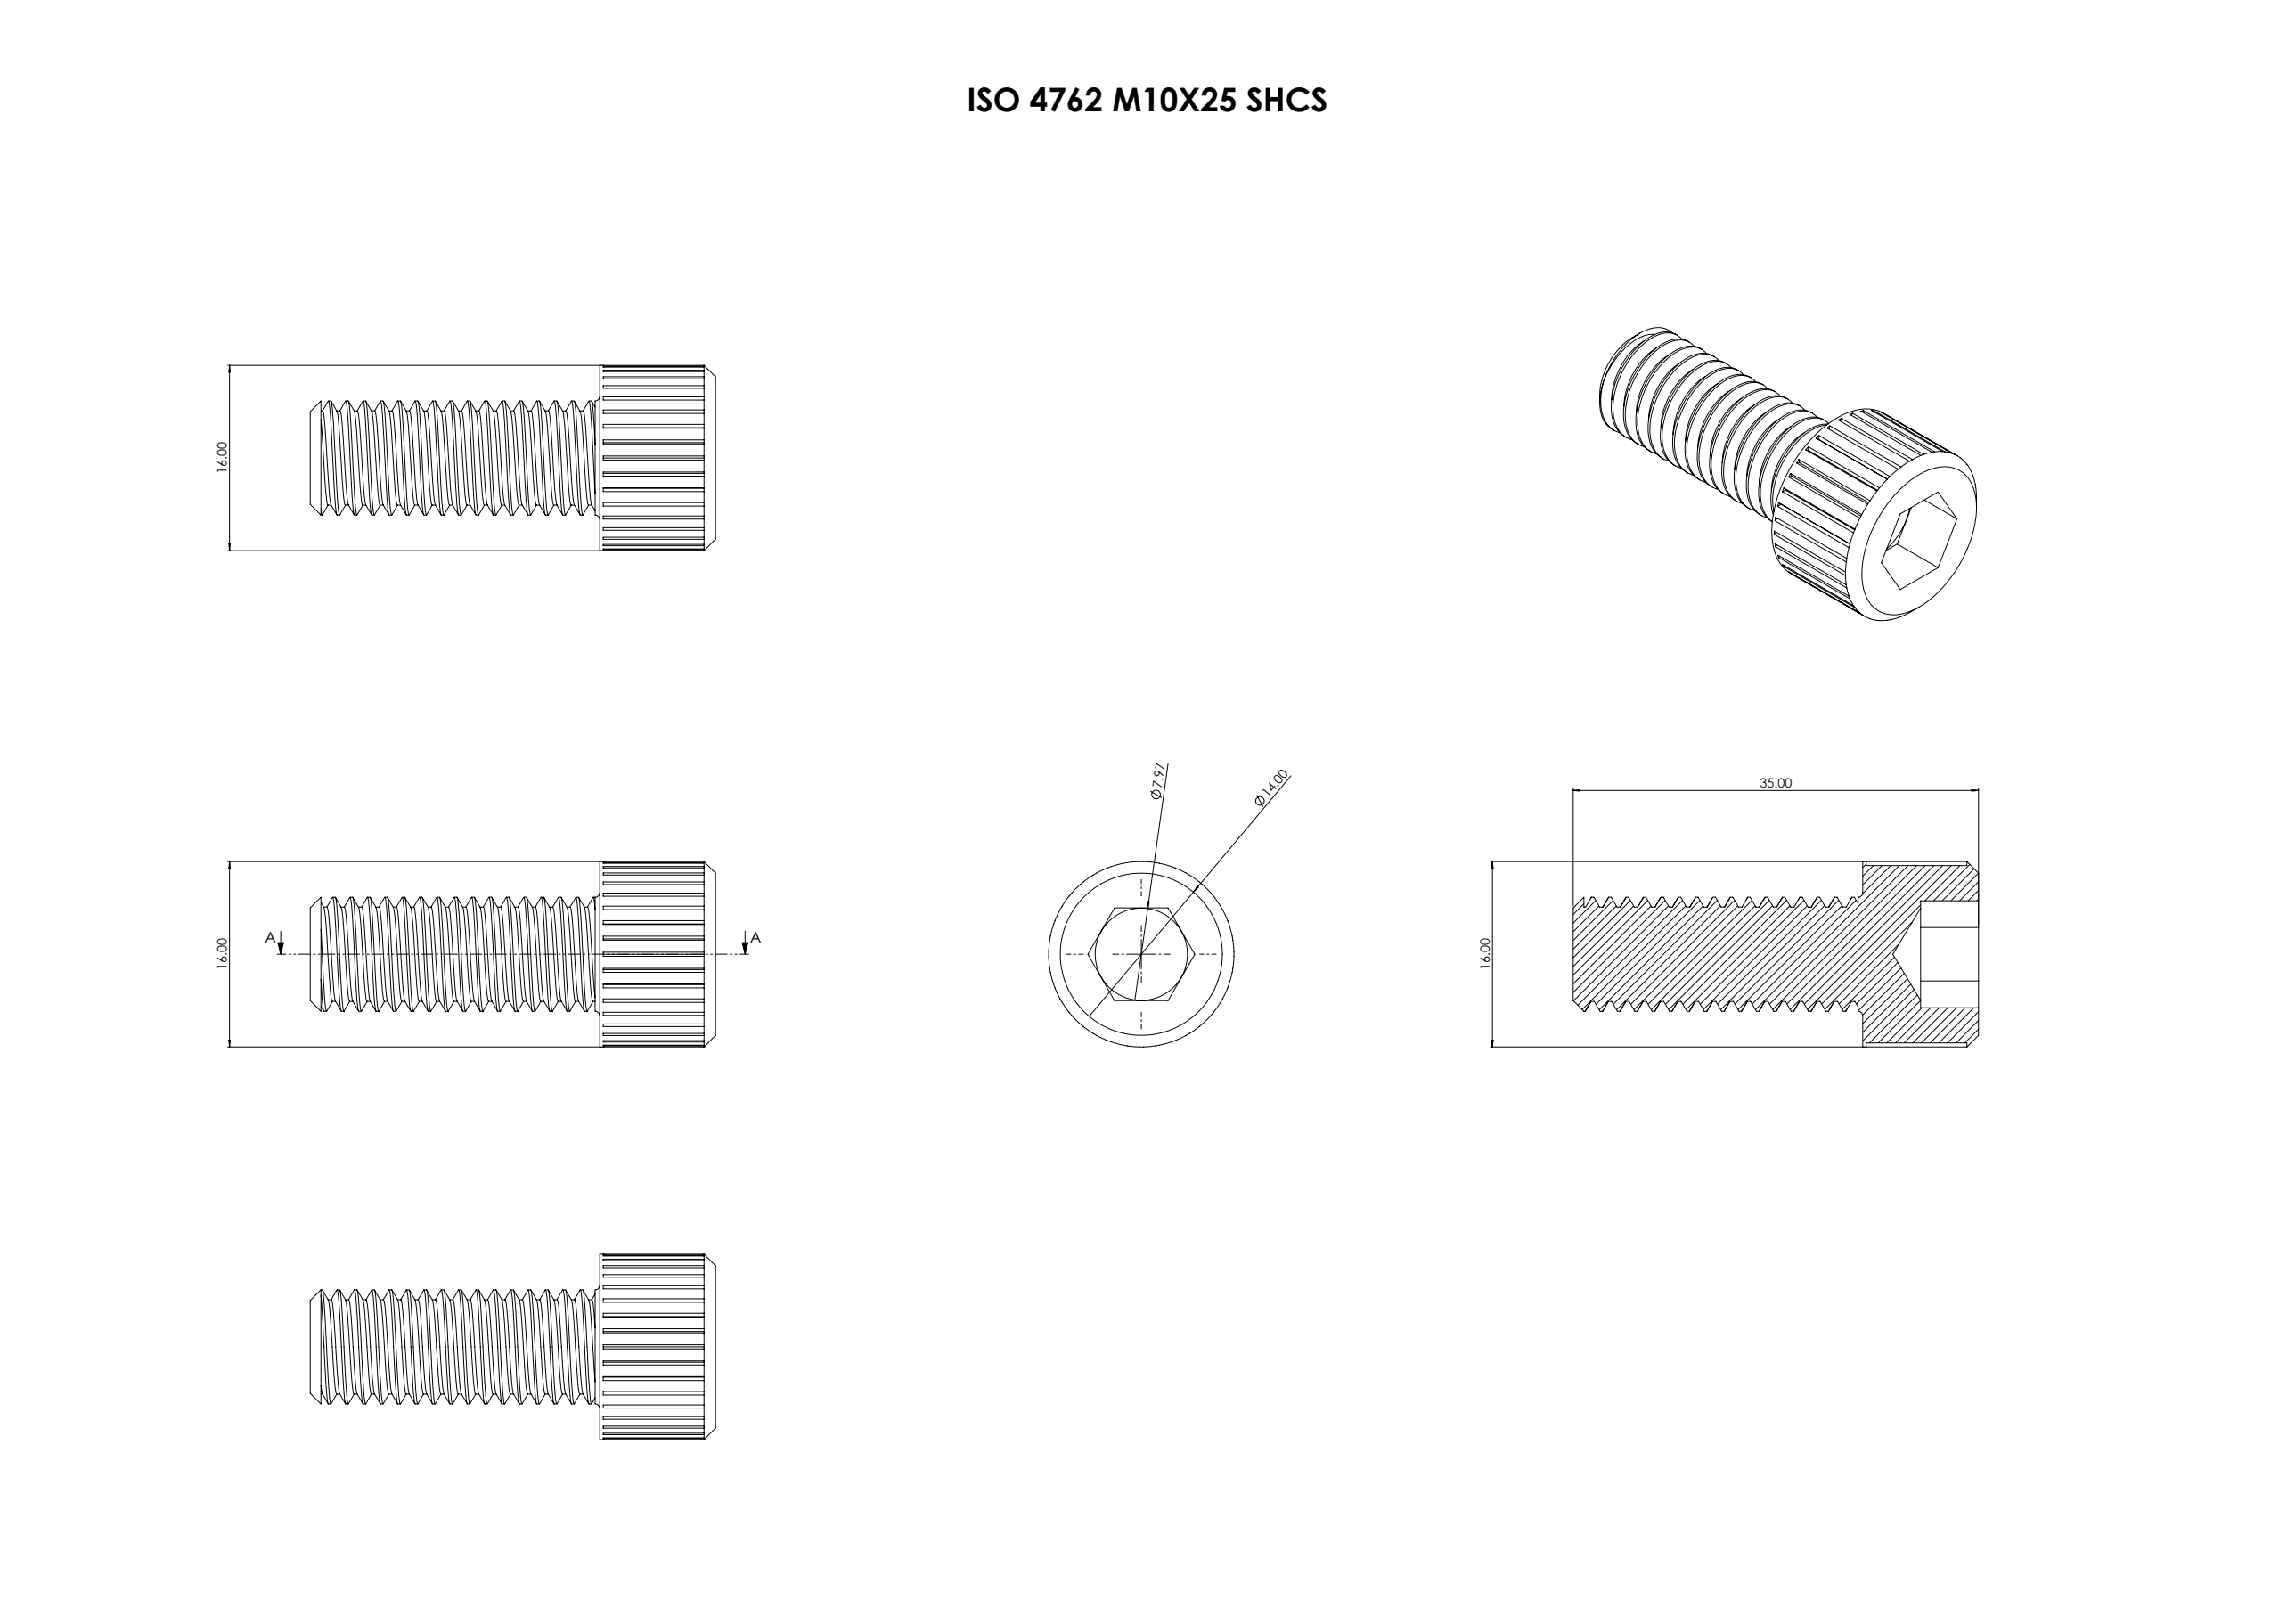
ISO-10303-21;
HEADER;
/* Generated by software containing ST-Developer
 * from STEP Tools, Inc. (www.steptools.com) 
 */

FILE_DESCRIPTION(
/* description */ (''),
/* implementation_level */ '2;1');

FILE_NAME(
/* name */ '06_ISO_4762_M10x25_SHCS.step',
/* time_stamp */ '2026-10-11T08:27:52-07:00',
/* author */ (''),
/* organization */ (''),
/* preprocessor_version */ 'ST-DEVELOPER v20.2',
/* originating_system */ 'Autodesk Translation Framework v15.15.0.0',
/* authorisation */ '');

FILE_SCHEMA (('AUTOMOTIVE_DESIGN { 1 0 10303 214 3 1 1 }'));
ENDSEC;

DATA;
#10=MECHANICAL_DESIGN_GEOMETRIC_PRESENTATION_REPRESENTATION('',(#924),#94301);
#479=B_SPLINE_CURVE_WITH_KNOTS('',3,(#84087,#84088,#84089,#84090,#84091,
#84092,#84093,#84094,#84095,#84096),.UNSPECIFIED.,.F.,.F.,(4,3,3,4),(-4.0932327200247,
-3.97004432054779,-2.97753324041084,-2.06652207565086),.UNSPECIFIED.);
#480=B_SPLINE_CURVE_WITH_KNOTS('',3,(#84099,#84100,#84101,#84102,#84103,
#84104,#84105,#84106,#84107,#84108),.UNSPECIFIED.,.F.,.F.,(4,3,3,4),(0.,
0.496255540068463,0.992511080136944,1.11488200921589),.UNSPECIFIED.);
#481=B_SPLINE_CURVE_WITH_KNOTS('',3,(#84113,#84114,#84115,#84116,#84117,
#84118,#84119,#84120,#84121,#84122,#84123,#84124,#84125,#84126,#84127,#84128,
#84129,#84130,#84131,#84132,#84133,#84134),.UNSPECIFIED.,.F.,.F.,(4,3,3,
3,3,3,3,4),(-10.3764180272043,-9.92511080136948,-8.93259972123253,-7.94008864109558,
-6.94757756095863,-5.95506648082169,-4.96255540068474,-4.0932327200247),
 .UNSPECIFIED.);
#482=B_SPLINE_CURVE_WITH_KNOTS('',3,(#84135,#84136,#84137,#84138,#84139,
#84140,#84141,#84142,#84143,#84144,#84145,#84146,#84147,#84148,#84149,#84150,
#84151,#84152,#84153,#84154,#84155,#84156),.UNSPECIFIED.,.F.,.F.,(4,3,3,
3,3,3,3,4),(1.11488200921589,1.98502216027389,2.97753324041084,3.97004432054779,
4.96255540068474,5.95506648082169,6.94757756095864,7.39806731639547),
 .UNSPECIFIED.);
#483=B_SPLINE_CURVE_WITH_KNOTS('',3,(#84161,#84162,#84163,#84164,#84165,
#84166,#84167,#84168,#84169,#84170,#84171,#84172,#84173,#84174,#84175,#84176,
#84177,#84178,#84179,#84180,#84181,#84182),.UNSPECIFIED.,.F.,.F.,(4,3,3,
3,3,3,3,4),(-16.6596033343839,-15.8801772821912,-14.8876662020542,-13.8951551219173,
-12.9026440417803,-11.9101329616434,-10.9176218815064,-10.3764180272043),
 .UNSPECIFIED.);
#484=B_SPLINE_CURVE_WITH_KNOTS('',3,(#84183,#84184,#84185,#84186,#84187,
#84188,#84189,#84190,#84191,#84192,#84193,#84194,#84195,#84196,#84197,#84198,
#84199,#84200,#84201,#84202,#84203,#84204),.UNSPECIFIED.,.F.,.F.,(4,3,3,
3,3,3,3,4),(7.39806731639547,7.94008864109559,8.93259972123253,9.92511080136948,
10.9176218815064,11.9101329616434,12.9026440417803,13.681252623575),
 .UNSPECIFIED.);
#485=B_SPLINE_CURVE_WITH_KNOTS('',3,(#84209,#84210,#84211,#84212,#84213,
#84214,#84215,#84216,#84217,#84218,#84219,#84220,#84221,#84222,#84223,#84224,
#84225,#84226,#84227,#84228,#84229,#84230,#84231,#84232,#84233),
 .UNSPECIFIED.,.F.,.F.,(4,3,3,3,3,3,3,3,4),(-22.9427886415635,-22.8277548431498,
-21.8352437630129,-20.8427326828759,-19.850221602739,-18.857710522602,-17.8651994424651,
-16.8726883623281,-16.6596033343839),.UNSPECIFIED.);
#486=B_SPLINE_CURVE_WITH_KNOTS('',3,(#84234,#84235,#84236,#84237,#84238,
#84239,#84240,#84241,#84242,#84243,#84244,#84245,#84246,#84247,#84248,#84249,
#84250,#84251,#84252,#84253,#84254,#84255,#84256,#84257,#84258),
 .UNSPECIFIED.,.F.,.F.,(4,3,3,3,3,3,3,3,4),(13.681252623575,13.8951551219173,
14.8876662020542,15.8801772821912,16.8726883623281,17.8651994424651,18.857710522602,
19.8502216027389,19.9644379307546),.UNSPECIFIED.);
#487=B_SPLINE_CURVE_WITH_KNOTS('',3,(#84263,#84264,#84265,#84266,#84267,
#84268,#84269,#84270,#84271,#84272,#84273,#84274,#84275,#84276,#84277,#84278,
#84279,#84280,#84281,#84282,#84283,#84284),.UNSPECIFIED.,.F.,.F.,(4,3,3,
3,3,3,3,4),(-29.225973948743,-28.7828213239715,-27.7903102438345,-26.7977991636976,
-25.8052880835606,-24.8127770034237,-23.8202659232867,-22.9427886415635),
 .UNSPECIFIED.);
#488=B_SPLINE_CURVE_WITH_KNOTS('',3,(#84285,#84286,#84287,#84288,#84289,
#84290,#84291,#84292,#84293,#84294,#84295,#84296,#84297,#84298,#84299,#84300,
#84301,#84302,#84303,#84304,#84305,#84306),.UNSPECIFIED.,.F.,.F.,(4,3,3,
3,3,3,3,4),(19.9644379307546,20.8427326828759,21.8352437630128,22.8277548431498,
23.8202659232867,24.8127770034237,25.8052880835606,26.2476232379342),
 .UNSPECIFIED.);
#489=B_SPLINE_CURVE_WITH_KNOTS('',3,(#84311,#84312,#84313,#84314,#84315,
#84316,#84317,#84318,#84319,#84320,#84321,#84322,#84323,#84324,#84325,#84326,
#84327,#84328,#84329,#84330,#84331,#84332),.UNSPECIFIED.,.F.,.F.,(4,3,3,
3,3,3,3,4),(-35.5091592559226,-34.7378878047932,-33.7453767246562,-32.7528656445193,
-31.7603545643823,-30.7678434842454,-29.7753324041084,-29.225973948743),
 .UNSPECIFIED.);
#490=B_SPLINE_CURVE_WITH_KNOTS('',3,(#84333,#84334,#84335,#84336,#84337,
#84338,#84339,#84340,#84341,#84342,#84343,#84344,#84345,#84346,#84347,#84348,
#84349,#84350,#84351,#84352,#84353,#84354),.UNSPECIFIED.,.F.,.F.,(4,3,3,
3,3,3,3,4),(26.2476232379342,26.7977991636976,27.7903102438345,28.7828213239715,
29.7753324041084,30.7678434842454,31.7603545643823,32.5308085451138),
 .UNSPECIFIED.);
#491=B_SPLINE_CURVE_WITH_KNOTS('',3,(#84359,#84360,#84361,#84362,#84363,
#84364,#84365,#84366,#84367,#84368,#84369,#84370,#84371,#84372,#84373,#84374,
#84375,#84376,#84377,#84378,#84379,#84380,#84381,#84382,#84383),
 .UNSPECIFIED.,.F.,.F.,(4,3,3,3,3,3,3,3,4),(-41.7923445631022,-41.6854653657518,
-40.6929542856149,-39.7004432054779,-38.707932125341,-37.715421045204,-36.7229099650671,
-35.7303988849301,-35.5091592559226),.UNSPECIFIED.);
#492=B_SPLINE_CURVE_WITH_KNOTS('',3,(#84384,#84385,#84386,#84387,#84388,
#84389,#84390,#84391,#84392,#84393,#84394,#84395,#84396,#84397,#84398,#84399,
#84400,#84401,#84402,#84403,#84404,#84405,#84406,#84407,#84408),
 .UNSPECIFIED.,.F.,.F.,(4,3,3,3,3,3,3,3,4),(32.5308085451138,32.7528656445192,
33.7453767246562,34.7378878047931,35.7303988849301,36.722909965067,37.715421045204,
38.7079321253409,38.8139938522934),.UNSPECIFIED.);
#493=B_SPLINE_CURVE_WITH_KNOTS('',3,(#84413,#84414,#84415,#84416,#84417,
#84418,#84419,#84420,#84421,#84422,#84423,#84424,#84425,#84426,#84427,#84428,
#84429,#84430,#84431,#84432,#84433,#84434),.UNSPECIFIED.,.F.,.F.,(4,3,3,
3,3,3,3,4),(-48.0755298702818,-47.6405318465735,-46.6480207664365,-45.6555096862996,
-44.6629986061626,-43.6704875260257,-42.6779764458888,-41.7923445631022),
 .UNSPECIFIED.);
#494=B_SPLINE_CURVE_WITH_KNOTS('',3,(#84435,#84436,#84437,#84438,#84439,
#84440,#84441,#84442,#84443,#84444,#84445,#84446,#84447,#84448,#84449,#84450,
#84451,#84452,#84453,#84454,#84455,#84456),.UNSPECIFIED.,.F.,.F.,(4,3,3,
3,3,3,3,4),(38.8139938522934,39.7004432054779,40.6929542856148,41.6854653657518,
42.6779764458887,43.6704875260257,44.6629986061626,45.097179159473),
 .UNSPECIFIED.);
#495=B_SPLINE_CURVE_WITH_KNOTS('',3,(#84461,#84462,#84463,#84464,#84465,
#84466,#84467,#84468,#84469,#84470,#84471,#84472,#84473,#84474,#84475,#84476,
#84477,#84478,#84479,#84480,#84481,#84482),.UNSPECIFIED.,.F.,.F.,(4,3,3,
3,3,3,3,4),(-54.3587151774614,-53.5955983273952,-52.6030872472582,-51.6105761671213,
-50.6180650869843,-49.6255540068474,-48.6330429267104,-48.0755298702818),
 .UNSPECIFIED.);
#496=B_SPLINE_CURVE_WITH_KNOTS('',3,(#84483,#84484,#84485,#84486,#84487,
#84488,#84489,#84490,#84491,#84492,#84493,#84494,#84495,#84496,#84497,#84498,
#84499,#84500,#84501,#84502,#84503,#84504),.UNSPECIFIED.,.F.,.F.,(4,3,3,
3,3,3,3,4),(45.097179159473,45.6555096862996,46.6480207664365,47.6405318465735,
48.6330429267104,49.6255540068474,50.6180650869843,51.3803644666526),
 .UNSPECIFIED.);
#497=B_SPLINE_CURVE_WITH_KNOTS('',3,(#84509,#84510,#84511,#84512,#84513,
#84514,#84515,#84516,#84517,#84518,#84519,#84520,#84521,#84522,#84523,#84524,
#84525,#84526,#84527,#84528,#84529,#84530,#84531,#84532,#84533),
 .UNSPECIFIED.,.F.,.F.,(4,3,3,3,3,3,3,3,4),(-60.641900484641,-60.5431758883538,
-59.5506648082169,-58.5581537280799,-57.565642647943,-56.573131567806,-55.5806204876691,
-54.5881094075321,-54.3587151774614),.UNSPECIFIED.);
#498=B_SPLINE_CURVE_WITH_KNOTS('',3,(#84534,#84535,#84536,#84537,#84538,
#84539,#84540,#84541,#84542,#84543,#84544,#84545,#84546,#84547,#84548,#84549,
#84550,#84551,#84552,#84553,#84554,#84555,#84556,#84557,#84558),
 .UNSPECIFIED.,.F.,.F.,(4,3,3,3,3,3,3,3,4),(51.3803644666526,51.6105761671213,
52.6030872472582,53.5955983273952,54.5881094075321,55.5806204876691,56.573131567806,
57.565642647943,57.6635497738322),.UNSPECIFIED.);
#499=B_SPLINE_CURVE_WITH_KNOTS('',3,(#84563,#84564,#84565,#84566,#84567,
#84568,#84569,#84570,#84571,#84572,#84573,#84574,#84575,#84576,#84577,#84578,
#84579,#84580,#84581,#84582,#84583,#84584),.UNSPECIFIED.,.F.,.F.,(4,3,3,
3,3,3,3,4),(-66.9250857918206,-66.4982423691755,-65.5057312890386,-64.5132202089016,
-63.5207091287647,-62.5281980486277,-61.5356869684908,-60.641900484641),
 .UNSPECIFIED.);
#500=B_SPLINE_CURVE_WITH_KNOTS('',3,(#84585,#84586,#84587,#84588,#84589,
#84590,#84591,#84592,#84593,#84594,#84595,#84596,#84597,#84598,#84599,#84600,
#84601,#84602,#84603,#84604,#84605,#84606),.UNSPECIFIED.,.F.,.F.,(4,3,3,
3,3,3,3,4),(57.6635497738322,58.5581537280799,59.5506648082169,60.5431758883538,
61.5356869684908,62.5281980486277,63.5207091287646,63.9467350810118),
 .UNSPECIFIED.);
#501=B_SPLINE_CURVE_WITH_KNOTS('',3,(#84611,#84612,#84613,#84614,#84615,
#84616,#84617,#84618,#84619,#84620,#84621,#84622,#84623,#84624,#84625,#84626,
#84627,#84628,#84629,#84630,#84631,#84632),.UNSPECIFIED.,.F.,.F.,(4,3,3,
3,3,3,3,4),(-73.2082710990002,-72.4533088499972,-71.4607977698602,-70.4682866897233,
-69.4757756095863,-68.4832645294494,-67.4907534493124,-66.9250857918206),
 .UNSPECIFIED.);
#502=B_SPLINE_CURVE_WITH_KNOTS('',3,(#84633,#84634,#84635,#84636,#84637,
#84638,#84639,#84640,#84641,#84642,#84643,#84644,#84645,#84646,#84647,#84648,
#84649,#84650,#84651,#84652,#84653,#84654),.UNSPECIFIED.,.F.,.F.,(4,3,3,
3,3,3,3,4),(63.9467350810118,64.5132202089016,65.5057312890385,66.4982423691755,
67.4907534493124,68.4832645294494,69.4757756095863,70.2299203881914),
 .UNSPECIFIED.);
#503=B_SPLINE_CURVE_WITH_KNOTS('',3,(#84659,#84660,#84661,#84662,#84663,
#84664,#84665,#84666,#84667,#84668,#84669,#84670,#84671,#84672,#84673,#84674,
#84675,#84676,#84677,#84678,#84679,#84680,#84681,#84682,#84683),
 .UNSPECIFIED.,.F.,.F.,(4,3,3,3,3,3,3,3,4),(-79.4914564061798,-79.4008864109558,
-78.4083753308189,-77.4158642506819,-76.423353170545,-75.430842090408,-74.4383310102711,
-73.4458199301341,-73.2082710990002),.UNSPECIFIED.);
#504=B_SPLINE_CURVE_WITH_KNOTS('',3,(#84684,#84685,#84686,#84687,#84688,
#84689,#84690,#84691,#84692,#84693,#84694,#84695,#84696,#84697,#84698,#84699,
#84700,#84701,#84702,#84703,#84704,#84705,#84706,#84707,#84708),
 .UNSPECIFIED.,.F.,.F.,(4,3,3,3,3,3,3,3,4),(70.2299203881914,70.4682866897233,
71.4607977698602,72.4533088499972,73.4458199301341,74.4383310102711,75.430842090408,
76.423353170545,76.513105695371),.UNSPECIFIED.);
#505=B_SPLINE_CURVE_WITH_KNOTS('',3,(#84713,#84714,#84715,#84716,#84717,
#84718,#84719,#84720,#84721,#84722,#84723,#84724,#84725,#84726,#84727,#84728,
#84729,#84730,#84731,#84732,#84733,#84734),.UNSPECIFIED.,.F.,.F.,(4,3,3,
3,3,3,3,4),(-85.7746417133594,-85.3559528917775,-84.3634418116406,-83.3709307315036,
-82.3784196513666,-81.3859085712297,-80.3933974910928,-79.4914564061798),
 .UNSPECIFIED.);
#506=B_SPLINE_CURVE_WITH_KNOTS('',3,(#84735,#84736,#84737,#84738,#84739,
#84740,#84741,#84742,#84743,#84744,#84745,#84746,#84747,#84748,#84749,#84750,
#84751,#84752,#84753,#84754,#84755,#84756),.UNSPECIFIED.,.F.,.F.,(4,3,3,
3,3,3,3,4),(76.513105695371,77.4158642506819,78.4083753308189,79.4008864109558,
80.3933974910927,81.3859085712297,82.3784196513666,82.7962910025506),
 .UNSPECIFIED.);
#507=B_SPLINE_CURVE_WITH_KNOTS('',3,(#84761,#84762,#84763,#84764,#84765,
#84766,#84767,#84768,#84769,#84770,#84771,#84772,#84773,#84774,#84775,#84776,
#84777,#84778,#84779,#84780,#84781,#84782),.UNSPECIFIED.,.F.,.F.,(4,3,3,
3,3,3,3,4),(-92.057827020539,-91.3110193725992,-90.3185082924622,-89.3259972123253,
-88.3334861321883,-87.3409750520514,-86.3484639719144,-85.7746417133594),
 .UNSPECIFIED.);
#508=B_SPLINE_CURVE_WITH_KNOTS('',3,(#84783,#84784,#84785,#84786,#84787,
#84788,#84789,#84790,#84791,#84792,#84793,#84794,#84795,#84796,#84797,#84798,
#84799,#84800,#84801,#84802,#84803,#84804),.UNSPECIFIED.,.F.,.F.,(4,3,3,
3,3,3,3,4),(82.7962910025506,83.3709307315036,84.3634418116405,85.3559528917775,
86.3484639719144,87.3409750520514,88.3334861321883,89.0794763097301),
 .UNSPECIFIED.);
#509=B_SPLINE_CURVE_WITH_KNOTS('',3,(#84809,#84810,#84811,#84812,#84813,
#84814,#84815,#84816,#84817,#84818,#84819,#84820,#84821,#84822,#84823,#84824,
#84825,#84826,#84827,#84828,#84829,#84830,#84831,#84832,#84833),
 .UNSPECIFIED.,.F.,.F.,(4,3,3,3,3,3,3,3,4),(-98.3410123277186,-98.2585969335579,
-97.2660858534209,-96.2735747732839,-95.281063693147,-94.28855261301,-93.2960415328731,
-92.3035304527361,-92.057827020539),.UNSPECIFIED.);
#510=B_SPLINE_CURVE_WITH_KNOTS('',3,(#84834,#84835,#84836,#84837,#84838,
#84839,#84840,#84841,#84842,#84843,#84844,#84845,#84846,#84847,#84848,#84849,
#84850,#84851,#84852,#84853,#84854,#84855,#84856,#84857,#84858),
 .UNSPECIFIED.,.F.,.F.,(4,3,3,3,3,3,3,3,4),(89.0794763097301,89.3259972123253,
90.3185082924622,91.3110193725992,92.3035304527361,93.2960415328731,94.28855261301,
95.2810636931469,95.3626616169097),.UNSPECIFIED.);
#511=B_SPLINE_CURVE_WITH_KNOTS('',3,(#84864,#84865,#84866,#84867),
 .UNSPECIFIED.,.F.,.F.,(4,4),(109.955742875643,110.784338646242),
 .UNSPECIFIED.);
#512=B_SPLINE_CURVE_WITH_KNOTS('',3,(#84873,#84874,#84875,#84876,#84877,
#84878,#84879,#84880,#84881,#84882,#84883),.UNSPECIFIED.,.F.,.F.,(4,1,1,
1,1,1,1,1,4),(103.672557568463,103.91826100066,104.910772080797,105.903283160934,
106.895794241071,107.888305321208,108.880816401345,109.873327481482,109.955742875643),
 .UNSPECIFIED.);
#513=B_SPLINE_CURVE_WITH_KNOTS('',3,(#84886,#84887,#84888,#84889,#84890,
#84891,#84892,#84893,#84894,#84895),.UNSPECIFIED.,.F.,.F.,(4,1,1,1,1,1,
1,4),(103.672557568463,104.583470724837,105.575981804974,106.568492885111,
107.561003965248,108.553515045385,109.049770585453,109.546026125522),
 .UNSPECIFIED.);
#514=B_SPLINE_CURVE_WITH_KNOTS('',3,(#84900,#84901,#84902,#84903,#84904,
#84905,#84906,#84907,#84908,#84909),.UNSPECIFIED.,.F.,.F.,(4,1,1,1,1,1,
1,4),(97.3893722612836,97.9631945198386,98.9557055999756,99.9482166801125,
100.940727760249,101.933238840386,102.925749920523,103.672557568463),
 .UNSPECIFIED.);
#515=B_SPLINE_CURVE_WITH_KNOTS('',3,(#84910,#84911,#84912,#84913,#84914,
#84915,#84916,#84917,#84918,#84919,#84920),.UNSPECIFIED.,.F.,.F.,(4,1,1,
1,1,1,1,1,4),(97.3893722612836,97.6358931638786,98.6284042440155,99.6209153241525,
100.613426404289,101.605937484426,102.598448564563,103.5909596447,103.672557568463),
 .UNSPECIFIED.);
#516=B_SPLINE_CURVE_WITH_KNOTS('',3,(#84925,#84926,#84927,#84928,#84929,
#84930,#84931,#84932,#84933,#84934),.UNSPECIFIED.,.F.,.F.,(4,1,1,1,1,1,
1,4),(91.106186954104,92.0081280390169,93.0006391191539,93.9931501992908,
94.9856612794278,95.9781723595647,96.9706834397017,97.3893722612836),
 .UNSPECIFIED.);
#517=B_SPLINE_CURVE_WITH_KNOTS('',3,(#84935,#84936,#84937,#84938,#84939,
#84940,#84941,#84942,#84943,#84944),.UNSPECIFIED.,.F.,.F.,(4,1,1,1,1,1,
1,4),(91.106186954104,91.6808266830569,92.6733377631939,93.6658488433308,
94.6583599234677,95.6508710036047,96.6433820837416,97.3893722612836),
 .UNSPECIFIED.);
#518=B_SPLINE_CURVE_WITH_KNOTS('',3,(#84949,#84950,#84951,#84952,#84953,
#84954,#84955,#84956,#84957,#84958,#84959),.UNSPECIFIED.,.F.,.F.,(4,1,1,
1,1,1,1,1,4),(84.8230016469244,85.0605504780583,86.0530615581953,87.0455726383322,
88.0380837184692,89.0305947986061,90.0231058787431,91.01561695888,91.106186954104),
 .UNSPECIFIED.);
#519=B_SPLINE_CURVE_WITH_KNOTS('',3,(#84960,#84961,#84962,#84963,#84964,
#84965,#84966,#84967,#84968,#84969),.UNSPECIFIED.,.F.,.F.,(4,1,1,1,1,1,
1,4),(84.8230016469244,85.7257602022352,86.7182712823722,87.7107823625091,
88.7032934426461,89.695804522783,90.68831560292,91.106186954104),
 .UNSPECIFIED.);
#520=B_SPLINE_CURVE_WITH_KNOTS('',3,(#84974,#84975,#84976,#84977,#84978,
#84979,#84980,#84981,#84982,#84983),.UNSPECIFIED.,.F.,.F.,(4,1,1,1,1,1,
1,4),(78.5398163397448,79.1054839972366,80.0979950773736,81.0905061575105,
82.0830172376475,83.0755283177844,84.0680393979214,84.8230016469244),
 .UNSPECIFIED.);
#521=B_SPLINE_CURVE_WITH_KNOTS('',3,(#84984,#84985,#84986,#84987,#84988,
#84989,#84990,#84991,#84992,#84993,#84994),.UNSPECIFIED.,.F.,.F.,(4,1,1,
1,1,1,1,1,4),(78.5398163397448,78.7781826412766,79.7706937214135,80.7632048015505,
81.7557158816874,82.7482269618244,83.7407380419613,84.7332491220983,84.8230016469244),
 .UNSPECIFIED.);
#522=B_SPLINE_CURVE_WITH_KNOTS('',3,(#84999,#85000,#85001,#85002,#85003,
#85004,#85005,#85006,#85007,#85008),.UNSPECIFIED.,.F.,.F.,(4,1,1,1,1,1,
1,4),(72.2566310325652,73.1504175164149,74.1429285965519,75.1354396766888,
76.1279507568258,77.1204618369627,78.1129729170997,78.5398163397448),
 .UNSPECIFIED.);
#523=B_SPLINE_CURVE_WITH_KNOTS('',3,(#85009,#85010,#85011,#85012,#85013,
#85014,#85015,#85016,#85017,#85018),.UNSPECIFIED.,.F.,.F.,(4,1,1,1,1,1,
1,4),(72.2566310325652,72.8231161604549,73.8156272405919,74.8081383207288,
75.8006494008658,76.7931604810027,77.7856715611396,78.5398163397448),
 .UNSPECIFIED.);
#524=B_SPLINE_CURVE_WITH_KNOTS('',3,(#85023,#85024,#85025,#85026,#85027,
#85028,#85029,#85030,#85031,#85032,#85033),.UNSPECIFIED.,.F.,.F.,(4,1,1,
1,1,1,1,1,4),(65.9734457253856,66.2028399554563,67.1953510355932,68.1878621157302,
69.1803731958671,70.1728842760041,71.165395356141,72.157906436278,72.2566310325652),
 .UNSPECIFIED.);
#525=B_SPLINE_CURVE_WITH_KNOTS('',3,(#85034,#85035,#85036,#85037,#85038,
#85039,#85040,#85041,#85042,#85043),.UNSPECIFIED.,.F.,.F.,(4,1,1,1,1,1,
1,4),(65.9734457253856,66.8680496796332,67.8605607597702,68.8530718399071,
69.8455829200441,70.838094000181,71.830605080318,72.2566310325652),
 .UNSPECIFIED.);
#526=B_SPLINE_CURVE_WITH_KNOTS('',3,(#85048,#85049,#85050,#85051,#85052,
#85053,#85054,#85055,#85056,#85057),.UNSPECIFIED.,.F.,.F.,(4,1,1,1,1,1,
1,4),(59.690260418206,60.2477734746346,61.2402845547716,62.2327956349085,
63.2253067150455,64.2178177951824,65.2103288753194,65.9734457253856),
 .UNSPECIFIED.);
#527=B_SPLINE_CURVE_WITH_KNOTS('',3,(#85058,#85059,#85060,#85061,#85062,
#85063,#85064,#85065,#85066,#85067,#85068),.UNSPECIFIED.,.F.,.F.,(4,1,1,
1,1,1,1,1,4),(59.690260418206,59.9204721186746,60.9129831988115,61.9054942789485,
62.8980053590854,63.8905164392224,64.8830275193593,65.8755385994963,65.9734457253856),
 .UNSPECIFIED.);
#528=B_SPLINE_CURVE_WITH_KNOTS('',3,(#85073,#85074,#85075,#85076,#85077,
#85078,#85079,#85080,#85081,#85082),.UNSPECIFIED.,.F.,.F.,(4,1,1,1,1,1,
1,4),(53.4070751110264,54.2927069938129,55.2852180739499,56.2777291540868,
57.2702402342238,58.2627513143607,59.2552623944977,59.690260418206),
 .UNSPECIFIED.);
#529=B_SPLINE_CURVE_WITH_KNOTS('',3,(#85083,#85084,#85085,#85086,#85087,
#85088,#85089,#85090,#85091,#85092),.UNSPECIFIED.,.F.,.F.,(4,1,1,1,1,1,
1,4),(53.4070751110264,53.9654056378529,54.9579167179898,55.9504277981268,
56.9429388782637,57.9354499584007,58.9279610385376,59.690260418206),
 .UNSPECIFIED.);
#530=B_SPLINE_CURVE_WITH_KNOTS('',3,(#85097,#85098,#85099,#85100,#85101,
#85102,#85103,#85104,#85105,#85106,#85107),.UNSPECIFIED.,.F.,.F.,(4,1,1,
1,1,1,1,1,4),(47.1238898038468,47.3451294328543,48.3376405129912,49.3301515931282,
50.3226626732651,51.3151737534021,52.307684833539,53.300195913676,53.4070751110264),
 .UNSPECIFIED.);
#531=B_SPLINE_CURVE_WITH_KNOTS('',3,(#85108,#85109,#85110,#85111,#85112,
#85113,#85114,#85115,#85116,#85117),.UNSPECIFIED.,.F.,.F.,(4,1,1,1,1,1,
1,4),(47.1238898038468,48.0103391570312,49.0028502371682,49.9953613173051,
50.9878723974421,51.980383477579,52.972894557716,53.4070751110264),
 .UNSPECIFIED.);
#532=B_SPLINE_CURVE_WITH_KNOTS('',3,(#85122,#85123,#85124,#85125,#85126,
#85127,#85128,#85129,#85130,#85131),.UNSPECIFIED.,.F.,.F.,(4,1,1,1,1,1,
1,4),(40.8407044966672,41.3900629520326,42.3825740321696,43.3750851123065,
44.3675961924435,45.3601072725804,46.3526183527174,47.1238898038468),
 .UNSPECIFIED.);
#533=B_SPLINE_CURVE_WITH_KNOTS('',3,(#85132,#85133,#85134,#85135,#85136,
#85137,#85138,#85139,#85140,#85141,#85142),.UNSPECIFIED.,.F.,.F.,(4,1,1,
1,1,1,1,1,4),(40.8407044966672,41.0627615960726,42.0552726762095,43.0477837563465,
44.0402948364834,45.0328059166204,46.0253169967573,47.0178280768943,47.1238898038468),
 .UNSPECIFIED.);
#534=B_SPLINE_CURVE_WITH_KNOTS('',3,(#85147,#85148,#85149,#85150,#85151,
#85152,#85153,#85154,#85155,#85156),.UNSPECIFIED.,.F.,.F.,(4,1,1,1,1,1,
1,4),(34.5575191894876,35.4349964712109,36.4275075513479,37.4200186314848,
38.4125297116218,39.4050407917587,40.3975518718957,40.8407044966672),
 .UNSPECIFIED.);
#535=B_SPLINE_CURVE_WITH_KNOTS('',3,(#85157,#85158,#85159,#85160,#85161,
#85162,#85163,#85164,#85165,#85166),.UNSPECIFIED.,.F.,.F.,(4,1,1,1,1,1,
1,4),(34.5575191894876,35.1076951152509,36.1002061953878,37.0927172755248,
38.0852283556617,39.0777394357987,40.0702505159356,40.8407044966672),
 .UNSPECIFIED.);
#536=B_SPLINE_CURVE_WITH_KNOTS('',3,(#85171,#85172,#85173,#85174,#85175,
#85176,#85177,#85178,#85179,#85180,#85181),.UNSPECIFIED.,.F.,.F.,(4,1,1,
1,1,1,1,1,4),(28.2743338823081,28.4874189102523,29.4799299903892,30.4724410705262,
31.4649521506631,32.4574632308001,33.449974310937,34.442485391074,34.5575191894876),
 .UNSPECIFIED.);
#537=B_SPLINE_CURVE_WITH_KNOTS('',3,(#85182,#85183,#85184,#85185,#85186,
#85187,#85188,#85189,#85190,#85191),.UNSPECIFIED.,.F.,.F.,(4,1,1,1,1,1,
1,4),(28.2743338823081,29.1526286344292,30.1451397145662,31.1376507947031,
32.1301618748401,33.122672954977,34.115184035114,34.5575191894876),
 .UNSPECIFIED.);
#538=B_SPLINE_CURVE_WITH_KNOTS('',3,(#85196,#85197,#85198,#85199,#85200,
#85201,#85202,#85203,#85204,#85205),.UNSPECIFIED.,.F.,.F.,(4,1,1,1,1,1,
1,4),(21.9911485751285,22.5323524294306,23.5248635095676,24.5173745897045,
25.5098856698415,26.5023967499784,27.4949078301153,28.2743338823081),
 .UNSPECIFIED.);
#539=B_SPLINE_CURVE_WITH_KNOTS('',3,(#85206,#85207,#85208,#85209,#85210,
#85211,#85212,#85213,#85214,#85215,#85216),.UNSPECIFIED.,.F.,.F.,(4,1,1,
1,1,1,1,1,4),(21.9911485751285,22.2050510734706,23.1975621536075,24.1900732337445,
25.1825843138814,26.1750953940184,27.1676064741553,28.1601175542923,28.2743338823081),
 .UNSPECIFIED.);
#540=B_SPLINE_CURVE_WITH_KNOTS('',3,(#85221,#85222,#85223,#85224,#85225,
#85226,#85227,#85228,#85229,#85230),.UNSPECIFIED.,.F.,.F.,(4,1,1,1,1,1,
1,4),(15.7079632679489,16.5772859486089,17.5697970287459,18.5623081088828,
19.5548191890198,20.5473302691567,21.5398413492937,21.9911485751285),
 .UNSPECIFIED.);
#541=B_SPLINE_CURVE_WITH_KNOTS('',3,(#85231,#85232,#85233,#85234,#85235,
#85236,#85237,#85238,#85239,#85240),.UNSPECIFIED.,.F.,.F.,(4,1,1,1,1,1,
1,4),(15.7079632679489,16.2499845926489,17.2424956727859,18.2350067529228,
19.2275178330597,20.2200289131967,21.2125399933336,21.9911485751285),
 .UNSPECIFIED.);
#542=B_SPLINE_CURVE_WITH_KNOTS('',3,(#85243,#85244,#85245,#85246,#85247,
#85248,#85249,#85250,#85251,#85252,#85253,#85254,#85255,#85256,#85257,#85258,
#85259,#85260,#85261,#85262,#85263,#85264,#85265,#85266,#85267,#85268,#85269,
#85270,#85271,#85272,#85273,#85274,#85275,#85276,#85277,#85278,#85279,#85280,
#85281,#85282,#85283,#85284,#85285,#85286,#85287,#85288,#85289,#85290,#85291,
#85292,#85293,#85294,#85295,#85296,#85297,#85298,#85299,#85300,#85301,#85302,
#85303,#85304,#85305,#85306,#85307,#85308,#85309,#85310,#85311,#85312,#85313,
#85314,#85315,#85316,#85317,#85318,#85319,#85320,#85321,#85322,#85323,#85324,
#85325,#85326,#85327,#85328,#85329,#85330,#85331,#85332,#85333,#85334,#85335,
#85336,#85337,#85338,#85339,#85340,#85341,#85342,#85343,#85344,#85345,#85346,
#85347,#85348),.UNSPECIFIED.,.F.,.F.,(4,3,3,3,3,3,3,3,3,3,3,3,3,3,3,3,3,
3,3,3,3,3,3,3,3,3,3,3,3,3,3,3,3,3,3,4),(-0.937740963081717,-0.904107646522432,
-0.866863955687421,-0.842197390067725,-0.832993449352449,-0.824789559002339,
-0.786675044092378,-0.747365526802366,-0.730167612987985,-0.721368607918277,
-0.713926887194103,-0.67422506805026,-0.633949893432139,-0.593512146517175,
-0.563183836330951,-0.549662025807026,-0.544150077215339,-0.502692185308048,
-0.472198905772281,-0.432024673306818,-0.391226520653541,-0.378538710027433,
-0.371922566564841,-0.366074525313514,-0.324929610892798,-0.282818014698314,
-0.241021666268101,-0.210893957984588,-0.197713085610552,-0.18926685442852,
-0.183259350799863,-0.140444090930293,-0.0970669920848681,-0.0537376549097892,
-0.0109807787802793,0.),.UNSPECIFIED.);
#543=B_SPLINE_CURVE_WITH_KNOTS('',3,(#85353,#85354,#85355,#85356,#85357,
#85358,#85359,#85360,#85361,#85362,#85363,#85364,#85365,#85366,#85367,#85368,
#85369,#85370,#85371,#85372,#85373,#85374,#85375,#85376,#85377,#85378,#85379,
#85380,#85381,#85382,#85383,#85384,#85385,#85386,#85387,#85388,#85389,#85390,
#85391,#85392,#85393,#85394,#85395,#85396,#85397,#85398,#85399,#85400,#85401,
#85402,#85403,#85404,#85405,#85406,#85407,#85408,#85409,#85410,#85411,#85412,
#85413,#85414,#85415,#85416,#85417,#85418,#85419,#85420,#85421,#85422,#85423,
#85424,#85425,#85426,#85427,#85428,#85429,#85430,#85431,#85432,#85433,#85434,
#85435,#85436,#85437,#85438,#85439,#85440,#85441,#85442,#85443,#85444,#85445,
#85446,#85447,#85448,#85449,#85450,#85451,#85452,#85453,#85454,#85455,#85456,
#85457,#85458),.UNSPECIFIED.,.F.,.F.,(4,3,3,3,3,3,3,3,3,3,3,3,3,3,3,3,3,
3,3,3,3,3,3,3,3,3,3,3,3,3,3,3,3,3,3,4),(-0.93397589402314,-0.893931319943522,
-0.850589364476838,-0.824132124098182,-0.808860826581905,-0.801881936601205,
-0.75913893284388,-0.717655756040688,-0.698300481629254,-0.686886922860203,
-0.681304646666429,-0.639280691781047,-0.597411580416329,-0.554877064916833,
-0.522976178292211,-0.510638772677517,-0.502211774582474,-0.496747396852542,
-0.456670538628237,-0.427273518418344,-0.386682137037577,-0.346195485729097,
-0.330880632953443,-0.325030908129725,-0.285554599290461,-0.246235559529426,
-0.208611124605633,-0.182534734029929,-0.16943344784353,-0.162203266198673,
-0.156994942118918,-0.117746206589189,-0.0795115062646132,-0.0397557531323066,
-0.00273238855256798,0.),.UNSPECIFIED.);
#544=B_SPLINE_CURVE_WITH_KNOTS('',3,(#85887,#85888,#85889,#85890,#85891,
#85892,#85893,#85894,#85895,#85896,#85897,#85898,#85899),.UNSPECIFIED.,
 .F.,.F.,(4,3,3,3,4),(95.3626616169097,96.2735747732839,97.2660858534208,
98.2585969335578,99.1696080983178),.UNSPECIFIED.);
#545=B_SPLINE_CURVE_WITH_KNOTS('',3,(#85901,#85902,#85903,#85904,#85905,
#85906,#85907,#85908,#85909,#85910,#85911,#85912,#85913,#85914,#85915,#85916,
#85917,#85918,#85919,#85920,#85921,#85922,#85923,#85924,#85925,#85926,#85927,
#85928,#85929,#85930,#85931,#85932,#85933,#85934,#85935,#85936,#85937,#85938,
#85939,#85940,#85941,#85942,#85943,#85944,#85945,#85946,#85947,#85948,#85949,
#85950,#85951,#85952,#85953,#85954,#85955,#85956,#85957,#85958,#85959,#85960,
#85961,#85962,#85963,#85964,#85965,#85966,#85967,#85968,#85969,#85970,#85971,
#85972,#85973,#85974,#85975,#85976,#85977,#85978,#85979,#85980,#85981,#85982,
#85983,#85984,#85985,#85986,#85987,#85988,#85989,#85990,#85991,#85992,#85993,
#85994,#85995,#85996,#85997,#85998,#85999,#86000,#86001,#86002,#86003,#86004,
#86005,#86006),.UNSPECIFIED.,.F.,.F.,(4,3,3,3,3,3,3,3,3,3,3,3,3,3,3,3,3,
3,3,3,3,3,3,3,3,3,3,3,3,3,3,3,3,3,3,4),(-0.93774096308178,-0.904107646522482,
-0.866863932192539,-0.842197368041274,-0.832993371681509,-0.824789553146923,
-0.786675013978796,-0.747365500452983,-0.730167588285441,-0.721368589124621,
-0.71392688849041,-0.674225052886835,-0.633949888794187,-0.593512143038715,
-0.563183833722111,-0.549662020429662,-0.544150075388719,-0.502692242333048,
-0.472198905772298,-0.432024869958226,-0.391226757969465,-0.378539422844806,
-0.371924656072871,-0.366074709533405,-0.324930003430011,-0.282818362179158,
-0.241021666268114,-0.210893957984599,-0.197713085610562,-0.189266835378695,
-0.183259344573423,-0.140443545162322,-0.0970662476713074,-0.0537369172547579,
-0.0109802554493726,0.),.UNSPECIFIED.);
#546=B_SPLINE_CURVE_WITH_KNOTS('',3,(#86007,#86008,#86009,#86010,#86011,
#86012,#86013,#86014,#86015),.UNSPECIFIED.,.F.,.F.,(4,1,1,1,1,1,4),(10.3764180272042,
11.2874291919642,12.2799402721011,13.2724513522381,14.264962432375,15.257473512512,
15.7079632679489),.UNSPECIFIED.);
#547=B_SPLINE_CURVE_WITH_KNOTS('',3,(#86021,#86022,#86023,#86024,#86025,
#86026,#86027,#86028,#86029,#86030,#86031,#86032,#86033,#86034,#86035,#86036,
#86037,#86038,#86039,#86040,#86041,#86042,#86043,#86044,#86045,#86046,#86047,
#86048,#86049,#86050,#86051,#86052,#86053,#86054,#86055,#86056,#86057,#86058,
#86059,#86060,#86061,#86062,#86063,#86064,#86065,#86066,#86067,#86068,#86069,
#86070,#86071,#86072,#86073,#86074,#86075,#86076,#86077,#86078,#86079,#86080,
#86081,#86082,#86083,#86084,#86085,#86086,#86087,#86088,#86089,#86090,#86091,
#86092,#86093,#86094,#86095,#86096,#86097,#86098,#86099,#86100,#86101,#86102,
#86103,#86104,#86105,#86106,#86107,#86108,#86109,#86110,#86111,#86112,#86113,
#86114,#86115,#86116,#86117,#86118,#86119,#86120,#86121,#86122,#86123,#86124,
#86125,#86126),.UNSPECIFIED.,.F.,.F.,(4,3,3,3,3,3,3,3,3,3,3,3,3,3,3,3,3,
3,3,3,3,3,3,3,3,3,3,3,3,3,3,3,3,3,3,4),(-0.933975894023116,-0.893931319943502,
-0.850589369822176,-0.824132129109434,-0.808860828934738,-0.801881933395027,
-0.7591389235175,-0.717655747880102,-0.698300462974381,-0.686886911899595,
-0.681304641078954,-0.639280632763917,-0.597411418690237,-0.554876943622257,
-0.522976087321272,-0.510638738070324,-0.502211740640668,-0.496747389660431,
-0.456670389952576,-0.427273518418318,-0.386682233223811,-0.346195805079578,
-0.330881843116922,-0.325030643604465,-0.285554427098605,-0.246235631641689,
-0.208611124605621,-0.182534734029918,-0.169433445615235,-0.162203295367182,
-0.156994995662412,-0.117746246746809,-0.079511462269274,-0.039755731134637,
-0.00273230733110789,0.),.UNSPECIFIED.);
#548=B_SPLINE_CURVE_WITH_KNOTS('',3,(#86129,#86130,#86131,#86132,#86133,
#86134,#86135,#86136,#86137),.UNSPECIFIED.,.F.,.F.,(4,1,1,1,1,1,4),(11.6147305479242,
12.1109860879927,12.6072416280611,13.5997527081981,14.592263788335,15.584774868472,
15.7079632679489),.UNSPECIFIED.);
#549=B_SPLINE_CURVE_WITH_KNOTS('',3,(#86566,#86567,#86568,#86569,#86570,
#86571,#86572,#86573,#86574,#86575,#86576,#86577,#86578),.UNSPECIFIED.,
 .F.,.F.,(4,3,3,3,4),(-101.236130173969,-100.7398746339,-100.243619093832,
-99.2511080136948,-98.3410123277186),.UNSPECIFIED.);
#885=B_SPLINE_SURFACE_WITH_KNOTS('',3,3,((#85459,#85460,#85461,#85462,#85463,
#85464,#85465,#85466,#85467,#85468,#85469,#85470,#85471,#85472,#85473,#85474,
#85475,#85476,#85477,#85478,#85479,#85480,#85481,#85482,#85483,#85484,#85485,
#85486,#85487,#85488,#85489,#85490,#85491,#85492,#85493,#85494,#85495,#85496,
#85497,#85498,#85499,#85500,#85501,#85502,#85503,#85504,#85505,#85506,#85507,
#85508,#85509,#85510,#85511,#85512,#85513,#85514,#85515,#85516,#85517,#85518,
#85519,#85520,#85521,#85522,#85523,#85524,#85525,#85526,#85527,#85528,#85529,
#85530,#85531,#85532,#85533,#85534,#85535,#85536,#85537,#85538,#85539,#85540,
#85541,#85542,#85543,#85544,#85545,#85546,#85547,#85548,#85549,#85550,#85551,
#85552,#85553,#85554,#85555,#85556,#85557,#85558,#85559,#85560,#85561,#85562,
#85563,#85564,#85565),(#85566,#85567,#85568,#85569,#85570,#85571,#85572,
#85573,#85574,#85575,#85576,#85577,#85578,#85579,#85580,#85581,#85582,#85583,
#85584,#85585,#85586,#85587,#85588,#85589,#85590,#85591,#85592,#85593,#85594,
#85595,#85596,#85597,#85598,#85599,#85600,#85601,#85602,#85603,#85604,#85605,
#85606,#85607,#85608,#85609,#85610,#85611,#85612,#85613,#85614,#85615,#85616,
#85617,#85618,#85619,#85620,#85621,#85622,#85623,#85624,#85625,#85626,#85627,
#85628,#85629,#85630,#85631,#85632,#85633,#85634,#85635,#85636,#85637,#85638,
#85639,#85640,#85641,#85642,#85643,#85644,#85645,#85646,#85647,#85648,#85649,
#85650,#85651,#85652,#85653,#85654,#85655,#85656,#85657,#85658,#85659,#85660,
#85661,#85662,#85663,#85664,#85665,#85666,#85667,#85668,#85669,#85670,#85671,
#85672),(#85673,#85674,#85675,#85676,#85677,#85678,#85679,#85680,#85681,
#85682,#85683,#85684,#85685,#85686,#85687,#85688,#85689,#85690,#85691,#85692,
#85693,#85694,#85695,#85696,#85697,#85698,#85699,#85700,#85701,#85702,#85703,
#85704,#85705,#85706,#85707,#85708,#85709,#85710,#85711,#85712,#85713,#85714,
#85715,#85716,#85717,#85718,#85719,#85720,#85721,#85722,#85723,#85724,#85725,
#85726,#85727,#85728,#85729,#85730,#85731,#85732,#85733,#85734,#85735,#85736,
#85737,#85738,#85739,#85740,#85741,#85742,#85743,#85744,#85745,#85746,#85747,
#85748,#85749,#85750,#85751,#85752,#85753,#85754,#85755,#85756,#85757,#85758,
#85759,#85760,#85761,#85762,#85763,#85764,#85765,#85766,#85767,#85768,#85769,
#85770,#85771,#85772,#85773,#85774,#85775,#85776,#85777,#85778,#85779),
(#85780,#85781,#85782,#85783,#85784,#85785,#85786,#85787,#85788,#85789,
#85790,#85791,#85792,#85793,#85794,#85795,#85796,#85797,#85798,#85799,#85800,
#85801,#85802,#85803,#85804,#85805,#85806,#85807,#85808,#85809,#85810,#85811,
#85812,#85813,#85814,#85815,#85816,#85817,#85818,#85819,#85820,#85821,#85822,
#85823,#85824,#85825,#85826,#85827,#85828,#85829,#85830,#85831,#85832,#85833,
#85834,#85835,#85836,#85837,#85838,#85839,#85840,#85841,#85842,#85843,#85844,
#85845,#85846,#85847,#85848,#85849,#85850,#85851,#85852,#85853,#85854,#85855,
#85856,#85857,#85858,#85859,#85860,#85861,#85862,#85863,#85864,#85865,#85866,
#85867,#85868,#85869,#85870,#85871,#85872,#85873,#85874,#85875,#85876,#85877,
#85878,#85879,#85880,#85881,#85882,#85883,#85884,#85885,#85886)),
 .UNSPECIFIED.,.F.,.F.,.F.,(4,4),(4,1,1,1,1,1,1,1,1,1,1,1,1,1,1,1,1,1,1,
1,1,1,1,1,1,1,1,1,1,1,1,1,1,1,1,1,1,1,1,1,1,1,1,1,1,1,1,1,1,1,1,1,1,1,1,
1,1,1,1,1,1,1,1,1,1,1,1,1,1,1,1,1,1,1,1,1,1,1,1,1,1,1,1,1,1,1,1,1,1,1,1,
1,1,1,1,1,1,1,1,1,1,1,1,1,4),(0.,0.0986691610045069),(8.30989595155332,
8.8061514916218,9.30240703169027,10.2949181118272,11.2874291919642,12.2799402721011,
13.2724513522381,14.264962432375,15.257473512512,16.2499845926489,17.2424956727859,
18.2350067529228,19.2275178330597,20.2200289131967,21.2125399933336,22.2050510734706,
23.1975621536075,24.1900732337445,25.1825843138814,26.1750953940184,27.1676064741553,
28.1601175542923,29.1526286344292,30.1451397145662,31.1376507947031,32.1301618748401,
33.122672954977,34.115184035114,35.1076951152509,36.1002061953878,37.0927172755248,
38.0852283556617,39.0777394357987,40.0702505159356,41.0627615960726,42.0552726762095,
43.0477837563465,44.0402948364834,45.0328059166204,46.0253169967573,47.0178280768943,
48.0103391570312,49.0028502371682,49.9953613173051,50.9878723974421,51.980383477579,
52.972894557716,53.9654056378529,54.9579167179898,55.9504277981268,56.9429388782637,
57.9354499584007,58.9279610385376,59.9204721186746,60.9129831988115,61.9054942789485,
62.8980053590854,63.8905164392224,64.8830275193593,65.8755385994963,66.8680496796332,
67.8605607597702,68.8530718399071,69.8455829200441,70.838094000181,71.830605080318,
72.8231161604549,73.8156272405919,74.8081383207288,75.8006494008658,76.7931604810027,
77.7856715611396,78.7781826412766,79.7706937214135,80.7632048015505,81.7557158816874,
82.7482269618244,83.7407380419613,84.7332491220983,85.7257602022352,86.7182712823722,
87.7107823625091,88.7032934426461,89.695804522783,90.68831560292,91.6808266830569,
92.6733377631939,93.6658488433308,94.6583599234677,95.6508710036047,96.6433820837416,
97.6358931638786,98.6284042440155,99.6209153241525,100.613426404289,101.605937484426,
102.598448564563,103.5909596447,104.583470724837,105.575981804974,106.568492885111,
107.561003965248,108.553515045385,109.049770585453,109.546026125522),
 .UNSPECIFIED.);
#886=B_SPLINE_SURFACE_WITH_KNOTS('',3,3,((#86138,#86139,#86140,#86141,#86142,
#86143,#86144,#86145,#86146,#86147,#86148,#86149,#86150,#86151,#86152,#86153,
#86154,#86155,#86156,#86157,#86158,#86159,#86160,#86161,#86162,#86163,#86164,
#86165,#86166,#86167,#86168,#86169,#86170,#86171,#86172,#86173,#86174,#86175,
#86176,#86177,#86178,#86179,#86180,#86181,#86182,#86183,#86184,#86185,#86186,
#86187,#86188,#86189,#86190,#86191,#86192,#86193,#86194,#86195,#86196,#86197,
#86198,#86199,#86200,#86201,#86202,#86203,#86204,#86205,#86206,#86207,#86208,
#86209,#86210,#86211,#86212,#86213,#86214,#86215,#86216,#86217,#86218,#86219,
#86220,#86221,#86222,#86223,#86224,#86225,#86226,#86227,#86228,#86229,#86230,
#86231,#86232,#86233,#86234,#86235,#86236,#86237,#86238,#86239,#86240,#86241,
#86242,#86243,#86244),(#86245,#86246,#86247,#86248,#86249,#86250,#86251,
#86252,#86253,#86254,#86255,#86256,#86257,#86258,#86259,#86260,#86261,#86262,
#86263,#86264,#86265,#86266,#86267,#86268,#86269,#86270,#86271,#86272,#86273,
#86274,#86275,#86276,#86277,#86278,#86279,#86280,#86281,#86282,#86283,#86284,
#86285,#86286,#86287,#86288,#86289,#86290,#86291,#86292,#86293,#86294,#86295,
#86296,#86297,#86298,#86299,#86300,#86301,#86302,#86303,#86304,#86305,#86306,
#86307,#86308,#86309,#86310,#86311,#86312,#86313,#86314,#86315,#86316,#86317,
#86318,#86319,#86320,#86321,#86322,#86323,#86324,#86325,#86326,#86327,#86328,
#86329,#86330,#86331,#86332,#86333,#86334,#86335,#86336,#86337,#86338,#86339,
#86340,#86341,#86342,#86343,#86344,#86345,#86346,#86347,#86348,#86349,#86350,
#86351),(#86352,#86353,#86354,#86355,#86356,#86357,#86358,#86359,#86360,
#86361,#86362,#86363,#86364,#86365,#86366,#86367,#86368,#86369,#86370,#86371,
#86372,#86373,#86374,#86375,#86376,#86377,#86378,#86379,#86380,#86381,#86382,
#86383,#86384,#86385,#86386,#86387,#86388,#86389,#86390,#86391,#86392,#86393,
#86394,#86395,#86396,#86397,#86398,#86399,#86400,#86401,#86402,#86403,#86404,
#86405,#86406,#86407,#86408,#86409,#86410,#86411,#86412,#86413,#86414,#86415,
#86416,#86417,#86418,#86419,#86420,#86421,#86422,#86423,#86424,#86425,#86426,
#86427,#86428,#86429,#86430,#86431,#86432,#86433,#86434,#86435,#86436,#86437,
#86438,#86439,#86440,#86441,#86442,#86443,#86444,#86445,#86446,#86447,#86448,
#86449,#86450,#86451,#86452,#86453,#86454,#86455,#86456,#86457,#86458),
(#86459,#86460,#86461,#86462,#86463,#86464,#86465,#86466,#86467,#86468,
#86469,#86470,#86471,#86472,#86473,#86474,#86475,#86476,#86477,#86478,#86479,
#86480,#86481,#86482,#86483,#86484,#86485,#86486,#86487,#86488,#86489,#86490,
#86491,#86492,#86493,#86494,#86495,#86496,#86497,#86498,#86499,#86500,#86501,
#86502,#86503,#86504,#86505,#86506,#86507,#86508,#86509,#86510,#86511,#86512,
#86513,#86514,#86515,#86516,#86517,#86518,#86519,#86520,#86521,#86522,#86523,
#86524,#86525,#86526,#86527,#86528,#86529,#86530,#86531,#86532,#86533,#86534,
#86535,#86536,#86537,#86538,#86539,#86540,#86541,#86542,#86543,#86544,#86545,
#86546,#86547,#86548,#86549,#86550,#86551,#86552,#86553,#86554,#86555,#86556,
#86557,#86558,#86559,#86560,#86561,#86562,#86563,#86564,#86565)),
 .UNSPECIFIED.,.F.,.F.,.F.,(4,4),(4,1,1,1,1,1,1,1,1,1,1,1,1,1,1,1,1,1,1,
1,1,1,1,1,1,1,1,1,1,1,1,1,1,1,1,1,1,1,1,1,1,1,1,1,1,1,1,1,1,1,1,1,1,1,1,
1,1,1,1,1,1,1,1,1,1,1,1,1,1,1,1,1,1,1,1,1,1,1,1,1,1,1,1,1,1,1,1,1,1,1,1,
1,1,1,1,1,1,1,1,1,1,1,1,1,4),(0.,0.0986691610045069),(11.6147305479242,
12.1109860879927,12.6072416280611,13.5997527081981,14.592263788335,15.584774868472,
16.5772859486089,17.5697970287459,18.5623081088828,19.5548191890198,20.5473302691567,
21.5398413492937,22.5323524294306,23.5248635095676,24.5173745897045,25.5098856698415,
26.5023967499784,27.4949078301153,28.4874189102523,29.4799299903892,30.4724410705262,
31.4649521506631,32.4574632308001,33.449974310937,34.442485391074,35.4349964712109,
36.4275075513479,37.4200186314848,38.4125297116218,39.4050407917587,40.3975518718957,
41.3900629520326,42.3825740321696,43.3750851123065,44.3675961924435,45.3601072725804,
46.3526183527174,47.3451294328543,48.3376405129912,49.3301515931282,50.3226626732651,
51.3151737534021,52.307684833539,53.300195913676,54.2927069938129,55.2852180739499,
56.2777291540868,57.2702402342238,58.2627513143607,59.2552623944977,60.2477734746346,
61.2402845547716,62.2327956349085,63.2253067150455,64.2178177951824,65.2103288753194,
66.2028399554563,67.1953510355932,68.1878621157302,69.1803731958671,70.1728842760041,
71.165395356141,72.157906436278,73.1504175164149,74.1429285965519,75.1354396766888,
76.1279507568258,77.1204618369627,78.1129729170997,79.1054839972366,80.0979950773736,
81.0905061575105,82.0830172376475,83.0755283177844,84.0680393979214,85.0605504780583,
86.0530615581953,87.0455726383322,88.0380837184692,89.0305947986061,90.0231058787431,
91.01561695888,92.0081280390169,93.0006391191539,93.9931501992908,94.9856612794278,
95.9781723595647,96.9706834397017,97.9631945198386,98.9557055999756,99.9482166801125,
100.940727760249,101.933238840386,102.925749920523,103.91826100066,104.910772080797,
105.903283160934,106.895794241071,107.888305321208,108.880816401345,109.873327481482,
110.865838561619,111.858349641756,112.354605181824,112.850860721893),
 .UNSPECIFIED.);
#896=SHAPE_REPRESENTATION_RELATIONSHIP('SRR','None',#94376,#910);
#910=ADVANCED_BREP_SHAPE_REPRESENTATION('',(#938),#94292);
#924=STYLED_ITEM('',(#94588),#938);
#938=MANIFOLD_SOLID_BREP('Body1',#51023);
#955=TOROIDAL_SURFACE('',#54535,5.325,0.4);
#1030=FACE_BOUND('',#18207,.T.);
#1031=FACE_BOUND('',#18360,.T.);
#1032=FACE_BOUND('',#18366,.T.);
#1157=CYLINDRICAL_SURFACE('',#54492,4.925);
#1158=CYLINDRICAL_SURFACE('',#54494,4.925);
#1159=CYLINDRICAL_SURFACE('',#54495,4.925);
#1160=CYLINDRICAL_SURFACE('',#54496,4.925);
#1161=CYLINDRICAL_SURFACE('',#54497,4.925);
#1162=CYLINDRICAL_SURFACE('',#54498,4.925);
#1163=CYLINDRICAL_SURFACE('',#54499,4.925);
#1164=CYLINDRICAL_SURFACE('',#54500,4.925);
#1165=CYLINDRICAL_SURFACE('',#54501,4.925);
#1166=CYLINDRICAL_SURFACE('',#54502,4.925);
#1167=CYLINDRICAL_SURFACE('',#54503,4.925);
#1168=CYLINDRICAL_SURFACE('',#54504,4.925);
#1169=CYLINDRICAL_SURFACE('',#54505,4.925);
#1170=CYLINDRICAL_SURFACE('',#54506,4.925);
#1171=CYLINDRICAL_SURFACE('',#54507,4.925);
#1172=CYLINDRICAL_SURFACE('',#54508,4.925);
#1173=CYLINDRICAL_SURFACE('',#54509,4.0705);
#1174=CYLINDRICAL_SURFACE('',#54511,4.0705);
#1175=CYLINDRICAL_SURFACE('',#54513,4.0705);
#1176=CYLINDRICAL_SURFACE('',#54514,4.0705);
#1177=CYLINDRICAL_SURFACE('',#54515,4.0705);
#1178=CYLINDRICAL_SURFACE('',#54516,4.0705);
#1179=CYLINDRICAL_SURFACE('',#54517,4.0705);
#1180=CYLINDRICAL_SURFACE('',#54518,4.0705);
#1181=CYLINDRICAL_SURFACE('',#54519,4.0705);
#1182=CYLINDRICAL_SURFACE('',#54520,4.0705);
#1183=CYLINDRICAL_SURFACE('',#54521,4.0705);
#1184=CYLINDRICAL_SURFACE('',#54522,4.0705);
#1185=CYLINDRICAL_SURFACE('',#54523,4.0705);
#1186=CYLINDRICAL_SURFACE('',#54524,4.0705);
#1187=CYLINDRICAL_SURFACE('',#54525,4.0705);
#1188=CYLINDRICAL_SURFACE('',#54526,4.0705);
#1189=CYLINDRICAL_SURFACE('',#54534,4.0705);
#1190=CYLINDRICAL_SURFACE('',#54539,4.925);
#1191=CYLINDRICAL_SURFACE('',#54772,8.);
#5979=LINE('',#84085,#10507);
#5980=LINE('',#84112,#10508);
#5981=LINE('',#84160,#10509);
#5982=LINE('',#84208,#10510);
#5983=LINE('',#84262,#10511);
#5984=LINE('',#84310,#10512);
#5985=LINE('',#84358,#10513);
#5986=LINE('',#84412,#10514);
#5987=LINE('',#84460,#10515);
#5988=LINE('',#84508,#10516);
#5989=LINE('',#84562,#10517);
#5990=LINE('',#84610,#10518);
#5991=LINE('',#84658,#10519);
#5992=LINE('',#84712,#10520);
#5993=LINE('',#84760,#10521);
#5994=LINE('',#84808,#10522);
#5995=LINE('',#84862,#10523);
#5996=LINE('',#84872,#10524);
#5997=LINE('',#84899,#10525);
#5998=LINE('',#84924,#10526);
#5999=LINE('',#84948,#10527);
#6000=LINE('',#84973,#10528);
#6001=LINE('',#84998,#10529);
#6002=LINE('',#85022,#10530);
#6003=LINE('',#85047,#10531);
#6004=LINE('',#85072,#10532);
#6005=LINE('',#85096,#10533);
#6006=LINE('',#85121,#10534);
#6007=LINE('',#85146,#10535);
#6008=LINE('',#85170,#10536);
#6009=LINE('',#85195,#10537);
#6010=LINE('',#85220,#10538);
#6011=LINE('',#86591,#10539);
#6012=LINE('',#86593,#10540);
#6013=LINE('',#86595,#10541);
#6014=LINE('',#86596,#10542);
#6015=LINE('',#86600,#10543);
#6016=LINE('',#86603,#10544);
#6017=LINE('',#86604,#10545);
#6018=LINE('',#86610,#10546);
#6019=LINE('',#86612,#10547);
#6020=LINE('',#86614,#10548);
#6021=LINE('',#86615,#10549);
#6022=LINE('',#86619,#10550);
#6023=LINE('',#86622,#10551);
#6024=LINE('',#86623,#10552);
#6025=LINE('',#86629,#10553);
#6026=LINE('',#86631,#10554);
#6027=LINE('',#86633,#10555);
#6028=LINE('',#86634,#10556);
#6029=LINE('',#86638,#10557);
#6030=LINE('',#86641,#10558);
#6031=LINE('',#86642,#10559);
#6032=LINE('',#86648,#10560);
#6033=LINE('',#86650,#10561);
#6034=LINE('',#86652,#10562);
#6035=LINE('',#86653,#10563);
#6036=LINE('',#86657,#10564);
#6037=LINE('',#86660,#10565);
#6038=LINE('',#86661,#10566);
#6039=LINE('',#86667,#10567);
#6040=LINE('',#86669,#10568);
#6041=LINE('',#86671,#10569);
#6042=LINE('',#86672,#10570);
#6043=LINE('',#86676,#10571);
#6044=LINE('',#86679,#10572);
#6045=LINE('',#86680,#10573);
#6046=LINE('',#86686,#10574);
#6047=LINE('',#86688,#10575);
#6048=LINE('',#86690,#10576);
#6049=LINE('',#86691,#10577);
#6050=LINE('',#86695,#10578);
#6051=LINE('',#86698,#10579);
#6052=LINE('',#86699,#10580);
#6053=LINE('',#86705,#10581);
#6054=LINE('',#86707,#10582);
#6055=LINE('',#86709,#10583);
#6056=LINE('',#86710,#10584);
#6057=LINE('',#86714,#10585);
#6058=LINE('',#86717,#10586);
#6059=LINE('',#86718,#10587);
#6060=LINE('',#86724,#10588);
#6061=LINE('',#86726,#10589);
#6062=LINE('',#86728,#10590);
#6063=LINE('',#86729,#10591);
#6064=LINE('',#86733,#10592);
#6065=LINE('',#86736,#10593);
#6066=LINE('',#86737,#10594);
#6067=LINE('',#86743,#10595);
#6068=LINE('',#86745,#10596);
#6069=LINE('',#86747,#10597);
#6070=LINE('',#86748,#10598);
#6071=LINE('',#86752,#10599);
#6072=LINE('',#86755,#10600);
#6073=LINE('',#86756,#10601);
#6074=LINE('',#86762,#10602);
#6075=LINE('',#86764,#10603);
#6076=LINE('',#86766,#10604);
#6077=LINE('',#86767,#10605);
#6078=LINE('',#86771,#10606);
#6079=LINE('',#86774,#10607);
#6080=LINE('',#86775,#10608);
#6081=LINE('',#86781,#10609);
#6082=LINE('',#86783,#10610);
#6083=LINE('',#86785,#10611);
#6084=LINE('',#86786,#10612);
#6085=LINE('',#86790,#10613);
#6086=LINE('',#86793,#10614);
#6087=LINE('',#86794,#10615);
#6088=LINE('',#86800,#10616);
#6089=LINE('',#86802,#10617);
#6090=LINE('',#86804,#10618);
#6091=LINE('',#86805,#10619);
#6092=LINE('',#86809,#10620);
#6093=LINE('',#86812,#10621);
#6094=LINE('',#86813,#10622);
#6095=LINE('',#86819,#10623);
#6096=LINE('',#86821,#10624);
#6097=LINE('',#86823,#10625);
#6098=LINE('',#86824,#10626);
#6099=LINE('',#86828,#10627);
#6100=LINE('',#86831,#10628);
#6101=LINE('',#86832,#10629);
#6102=LINE('',#86838,#10630);
#6103=LINE('',#86840,#10631);
#6104=LINE('',#86842,#10632);
#6105=LINE('',#86843,#10633);
#6106=LINE('',#86847,#10634);
#6107=LINE('',#86850,#10635);
#6108=LINE('',#86851,#10636);
#6109=LINE('',#86857,#10637);
#6110=LINE('',#86859,#10638);
#6111=LINE('',#86861,#10639);
#6112=LINE('',#86862,#10640);
#6113=LINE('',#86866,#10641);
#6114=LINE('',#86869,#10642);
#6115=LINE('',#86870,#10643);
#6116=LINE('',#86876,#10644);
#6117=LINE('',#86878,#10645);
#6118=LINE('',#86880,#10646);
#6119=LINE('',#86881,#10647);
#6120=LINE('',#86885,#10648);
#6121=LINE('',#86888,#10649);
#6122=LINE('',#86889,#10650);
#6123=LINE('',#86895,#10651);
#6124=LINE('',#86897,#10652);
#6125=LINE('',#86899,#10653);
#6126=LINE('',#86900,#10654);
#6127=LINE('',#86904,#10655);
#6128=LINE('',#86907,#10656);
#6129=LINE('',#86908,#10657);
#6130=LINE('',#86914,#10658);
#6131=LINE('',#86916,#10659);
#6132=LINE('',#86918,#10660);
#6133=LINE('',#86919,#10661);
#6134=LINE('',#86924,#10662);
#6135=LINE('',#86928,#10663);
#6136=LINE('',#86929,#10664);
#6137=LINE('',#86937,#10665);
#6138=LINE('',#86939,#10666);
#6139=LINE('',#86941,#10667);
#6140=LINE('',#86942,#10668);
#6141=LINE('',#86946,#10669);
#6142=LINE('',#86949,#10670);
#6143=LINE('',#86950,#10671);
#6144=LINE('',#86956,#10672);
#6145=LINE('',#86958,#10673);
#6146=LINE('',#86960,#10674);
#6147=LINE('',#86961,#10675);
#6148=LINE('',#86965,#10676);
#6149=LINE('',#86968,#10677);
#6150=LINE('',#86969,#10678);
#6151=LINE('',#86975,#10679);
#6152=LINE('',#86977,#10680);
#6153=LINE('',#86979,#10681);
#6154=LINE('',#86980,#10682);
#6155=LINE('',#86984,#10683);
#6156=LINE('',#86987,#10684);
#6157=LINE('',#86988,#10685);
#6158=LINE('',#86994,#10686);
#6159=LINE('',#86996,#10687);
#6160=LINE('',#86998,#10688);
#6161=LINE('',#86999,#10689);
#6162=LINE('',#87003,#10690);
#6163=LINE('',#87006,#10691);
#6164=LINE('',#87007,#10692);
#6165=LINE('',#87013,#10693);
#6166=LINE('',#87015,#10694);
#6167=LINE('',#87017,#10695);
#6168=LINE('',#87018,#10696);
#6169=LINE('',#87022,#10697);
#6170=LINE('',#87025,#10698);
#6171=LINE('',#87026,#10699);
#6172=LINE('',#87032,#10700);
#6173=LINE('',#87034,#10701);
#6174=LINE('',#87036,#10702);
#6175=LINE('',#87037,#10703);
#6176=LINE('',#87041,#10704);
#6177=LINE('',#87044,#10705);
#6178=LINE('',#87045,#10706);
#6179=LINE('',#87051,#10707);
#6180=LINE('',#87053,#10708);
#6181=LINE('',#87055,#10709);
#6182=LINE('',#87056,#10710);
#6183=LINE('',#87060,#10711);
#6184=LINE('',#87063,#10712);
#6185=LINE('',#87064,#10713);
#6186=LINE('',#87070,#10714);
#6187=LINE('',#87072,#10715);
#6188=LINE('',#87074,#10716);
#6189=LINE('',#87075,#10717);
#6190=LINE('',#87079,#10718);
#6191=LINE('',#87082,#10719);
#6192=LINE('',#87083,#10720);
#6193=LINE('',#87089,#10721);
#6194=LINE('',#87091,#10722);
#6195=LINE('',#87093,#10723);
#6196=LINE('',#87094,#10724);
#6197=LINE('',#87098,#10725);
#6198=LINE('',#87101,#10726);
#6199=LINE('',#87102,#10727);
#6200=LINE('',#87108,#10728);
#6201=LINE('',#87110,#10729);
#6202=LINE('',#87112,#10730);
#6203=LINE('',#87113,#10731);
#6204=LINE('',#87117,#10732);
#6205=LINE('',#87120,#10733);
#6206=LINE('',#87121,#10734);
#6207=LINE('',#87127,#10735);
#6208=LINE('',#87129,#10736);
#6209=LINE('',#87131,#10737);
#6210=LINE('',#87132,#10738);
#6211=LINE('',#87136,#10739);
#6212=LINE('',#87139,#10740);
#6213=LINE('',#87140,#10741);
#6214=LINE('',#87146,#10742);
#6215=LINE('',#87148,#10743);
#6216=LINE('',#87150,#10744);
#6217=LINE('',#87151,#10745);
#6218=LINE('',#87155,#10746);
#6219=LINE('',#87158,#10747);
#6220=LINE('',#87159,#10748);
#6221=LINE('',#87165,#10749);
#6222=LINE('',#87167,#10750);
#6223=LINE('',#87169,#10751);
#6224=LINE('',#87170,#10752);
#6225=LINE('',#87174,#10753);
#6226=LINE('',#87177,#10754);
#6227=LINE('',#87178,#10755);
#6228=LINE('',#87184,#10756);
#6229=LINE('',#87186,#10757);
#6230=LINE('',#87188,#10758);
#6231=LINE('',#87189,#10759);
#6232=LINE('',#87193,#10760);
#6233=LINE('',#87196,#10761);
#6234=LINE('',#87197,#10762);
#6235=LINE('',#87203,#10763);
#6236=LINE('',#87205,#10764);
#6237=LINE('',#87207,#10765);
#6238=LINE('',#87208,#10766);
#6239=LINE('',#87212,#10767);
#6240=LINE('',#87215,#10768);
#6241=LINE('',#87216,#10769);
#6242=LINE('',#87222,#10770);
#6243=LINE('',#87224,#10771);
#6244=LINE('',#87226,#10772);
#6245=LINE('',#87227,#10773);
#6246=LINE('',#87231,#10774);
#6247=LINE('',#87234,#10775);
#6248=LINE('',#87235,#10776);
#6249=LINE('',#87241,#10777);
#6250=LINE('',#87243,#10778);
#6251=LINE('',#87245,#10779);
#6252=LINE('',#87246,#10780);
#6253=LINE('',#87250,#10781);
#6254=LINE('',#87253,#10782);
#6255=LINE('',#87254,#10783);
#6256=LINE('',#87262,#10784);
#6257=LINE('',#87263,#10785);
#6258=LINE('',#87266,#10786);
#6259=LINE('',#87268,#10787);
#6260=LINE('',#87269,#10788);
#6261=LINE('',#87272,#10789);
#6262=LINE('',#87273,#10790);
#6263=LINE('',#87279,#10791);
#6264=LINE('',#87284,#10792);
#6265=LINE('',#87286,#10793);
#6266=LINE('',#87288,#10794);
#6267=LINE('',#87289,#10795);
#6268=LINE('',#87292,#10796);
#6269=LINE('',#87294,#10797);
#6270=LINE('',#87295,#10798);
#6271=LINE('',#87298,#10799);
#6272=LINE('',#87300,#10800);
#6273=LINE('',#87301,#10801);
#6274=LINE('',#87304,#10802);
#6275=LINE('',#87306,#10803);
#6276=LINE('',#87307,#10804);
#6277=LINE('',#87310,#10805);
#6278=LINE('',#87312,#10806);
#6279=LINE('',#87313,#10807);
#6280=LINE('',#87315,#10808);
#6281=LINE('',#87316,#10809);
#6282=LINE('',#87322,#10810);
#6283=LINE('',#87341,#10811);
#6284=LINE('',#87364,#10812);
#10507=VECTOR('',#65799,5.);
#10508=VECTOR('',#65804,5.);
#10509=VECTOR('',#65807,5.);
#10510=VECTOR('',#65810,5.);
#10511=VECTOR('',#65813,5.);
#10512=VECTOR('',#65816,5.);
#10513=VECTOR('',#65819,5.);
#10514=VECTOR('',#65822,5.);
#10515=VECTOR('',#65825,5.);
#10516=VECTOR('',#65828,5.);
#10517=VECTOR('',#65831,5.);
#10518=VECTOR('',#65834,5.);
#10519=VECTOR('',#65837,5.);
#10520=VECTOR('',#65840,5.);
#10521=VECTOR('',#65843,5.);
#10522=VECTOR('',#65846,5.);
#10523=VECTOR('',#65849,4.0705);
#10524=VECTOR('',#65854,4.0705);
#10525=VECTOR('',#65859,4.0705);
#10526=VECTOR('',#65862,4.0705);
#10527=VECTOR('',#65865,4.0705);
#10528=VECTOR('',#65868,4.0705);
#10529=VECTOR('',#65871,4.0705);
#10530=VECTOR('',#65874,4.0705);
#10531=VECTOR('',#65877,4.0705);
#10532=VECTOR('',#65880,4.0705);
#10533=VECTOR('',#65883,4.0705);
#10534=VECTOR('',#65886,4.0705);
#10535=VECTOR('',#65889,4.0705);
#10536=VECTOR('',#65892,4.0705);
#10537=VECTOR('',#65895,4.0705);
#10538=VECTOR('',#65898,4.0705);
#10539=VECTOR('',#65931,10.);
#10540=VECTOR('',#65932,10.);
#10541=VECTOR('',#65933,10.);
#10542=VECTOR('',#65934,10.);
#10543=VECTOR('',#65939,10.);
#10544=VECTOR('',#65942,10.);
#10545=VECTOR('',#65943,10.);
#10546=VECTOR('',#65950,10.);
#10547=VECTOR('',#65951,10.);
#10548=VECTOR('',#65952,10.);
#10549=VECTOR('',#65953,10.);
#10550=VECTOR('',#65958,10.);
#10551=VECTOR('',#65961,10.);
#10552=VECTOR('',#65962,10.);
#10553=VECTOR('',#65969,10.);
#10554=VECTOR('',#65970,10.);
#10555=VECTOR('',#65971,10.);
#10556=VECTOR('',#65972,10.);
#10557=VECTOR('',#65977,10.);
#10558=VECTOR('',#65980,10.);
#10559=VECTOR('',#65981,10.);
#10560=VECTOR('',#65988,10.);
#10561=VECTOR('',#65989,10.);
#10562=VECTOR('',#65990,10.);
#10563=VECTOR('',#65991,10.);
#10564=VECTOR('',#65996,10.);
#10565=VECTOR('',#65999,10.);
#10566=VECTOR('',#66000,10.);
#10567=VECTOR('',#66007,10.);
#10568=VECTOR('',#66008,10.);
#10569=VECTOR('',#66009,10.);
#10570=VECTOR('',#66010,10.);
#10571=VECTOR('',#66015,10.);
#10572=VECTOR('',#66018,10.);
#10573=VECTOR('',#66019,10.);
#10574=VECTOR('',#66026,10.);
#10575=VECTOR('',#66027,10.);
#10576=VECTOR('',#66028,10.);
#10577=VECTOR('',#66029,10.);
#10578=VECTOR('',#66034,10.);
#10579=VECTOR('',#66037,10.);
#10580=VECTOR('',#66038,10.);
#10581=VECTOR('',#66045,10.);
#10582=VECTOR('',#66046,10.);
#10583=VECTOR('',#66047,10.);
#10584=VECTOR('',#66048,10.);
#10585=VECTOR('',#66053,10.);
#10586=VECTOR('',#66056,10.);
#10587=VECTOR('',#66057,10.);
#10588=VECTOR('',#66064,10.);
#10589=VECTOR('',#66065,10.);
#10590=VECTOR('',#66066,10.);
#10591=VECTOR('',#66067,10.);
#10592=VECTOR('',#66072,10.);
#10593=VECTOR('',#66075,10.);
#10594=VECTOR('',#66076,10.);
#10595=VECTOR('',#66083,10.);
#10596=VECTOR('',#66084,10.);
#10597=VECTOR('',#66085,10.);
#10598=VECTOR('',#66086,10.);
#10599=VECTOR('',#66091,10.);
#10600=VECTOR('',#66094,10.);
#10601=VECTOR('',#66095,10.);
#10602=VECTOR('',#66102,10.);
#10603=VECTOR('',#66103,10.);
#10604=VECTOR('',#66104,10.);
#10605=VECTOR('',#66105,10.);
#10606=VECTOR('',#66110,10.);
#10607=VECTOR('',#66113,10.);
#10608=VECTOR('',#66114,10.);
#10609=VECTOR('',#66121,10.);
#10610=VECTOR('',#66122,10.);
#10611=VECTOR('',#66123,10.);
#10612=VECTOR('',#66124,10.);
#10613=VECTOR('',#66129,10.);
#10614=VECTOR('',#66132,10.);
#10615=VECTOR('',#66133,10.);
#10616=VECTOR('',#66140,10.);
#10617=VECTOR('',#66141,10.);
#10618=VECTOR('',#66142,10.);
#10619=VECTOR('',#66143,10.);
#10620=VECTOR('',#66148,10.);
#10621=VECTOR('',#66151,10.);
#10622=VECTOR('',#66152,10.);
#10623=VECTOR('',#66159,10.);
#10624=VECTOR('',#66160,10.);
#10625=VECTOR('',#66161,10.);
#10626=VECTOR('',#66162,10.);
#10627=VECTOR('',#66167,10.);
#10628=VECTOR('',#66170,10.);
#10629=VECTOR('',#66171,10.);
#10630=VECTOR('',#66178,10.);
#10631=VECTOR('',#66179,10.);
#10632=VECTOR('',#66180,10.);
#10633=VECTOR('',#66181,10.);
#10634=VECTOR('',#66186,10.);
#10635=VECTOR('',#66189,10.);
#10636=VECTOR('',#66190,10.);
#10637=VECTOR('',#66197,10.);
#10638=VECTOR('',#66198,10.);
#10639=VECTOR('',#66199,10.);
#10640=VECTOR('',#66200,10.);
#10641=VECTOR('',#66205,10.);
#10642=VECTOR('',#66208,10.);
#10643=VECTOR('',#66209,10.);
#10644=VECTOR('',#66216,10.);
#10645=VECTOR('',#66217,10.);
#10646=VECTOR('',#66218,10.);
#10647=VECTOR('',#66219,10.);
#10648=VECTOR('',#66224,10.);
#10649=VECTOR('',#66227,10.);
#10650=VECTOR('',#66228,10.);
#10651=VECTOR('',#66235,10.);
#10652=VECTOR('',#66236,10.);
#10653=VECTOR('',#66237,10.);
#10654=VECTOR('',#66238,10.);
#10655=VECTOR('',#66243,10.);
#10656=VECTOR('',#66246,10.);
#10657=VECTOR('',#66247,10.);
#10658=VECTOR('',#66254,10.);
#10659=VECTOR('',#66255,10.);
#10660=VECTOR('',#66256,10.);
#10661=VECTOR('',#66257,10.);
#10662=VECTOR('',#66262,10.);
#10663=VECTOR('',#66267,10.);
#10664=VECTOR('',#66268,10.);
#10665=VECTOR('',#66277,10.);
#10666=VECTOR('',#66278,10.);
#10667=VECTOR('',#66279,10.);
#10668=VECTOR('',#66280,10.);
#10669=VECTOR('',#66285,10.);
#10670=VECTOR('',#66288,10.);
#10671=VECTOR('',#66289,10.);
#10672=VECTOR('',#66296,10.);
#10673=VECTOR('',#66297,10.);
#10674=VECTOR('',#66298,10.);
#10675=VECTOR('',#66299,10.);
#10676=VECTOR('',#66304,10.);
#10677=VECTOR('',#66307,10.);
#10678=VECTOR('',#66308,10.);
#10679=VECTOR('',#66315,10.);
#10680=VECTOR('',#66316,10.);
#10681=VECTOR('',#66317,10.);
#10682=VECTOR('',#66318,10.);
#10683=VECTOR('',#66323,10.);
#10684=VECTOR('',#66326,10.);
#10685=VECTOR('',#66327,10.);
#10686=VECTOR('',#66334,10.);
#10687=VECTOR('',#66335,10.);
#10688=VECTOR('',#66336,10.);
#10689=VECTOR('',#66337,10.);
#10690=VECTOR('',#66342,10.);
#10691=VECTOR('',#66345,10.);
#10692=VECTOR('',#66346,10.);
#10693=VECTOR('',#66353,10.);
#10694=VECTOR('',#66354,10.);
#10695=VECTOR('',#66355,10.);
#10696=VECTOR('',#66356,10.);
#10697=VECTOR('',#66361,10.);
#10698=VECTOR('',#66364,10.);
#10699=VECTOR('',#66365,10.);
#10700=VECTOR('',#66372,10.);
#10701=VECTOR('',#66373,10.);
#10702=VECTOR('',#66374,10.);
#10703=VECTOR('',#66375,10.);
#10704=VECTOR('',#66380,10.);
#10705=VECTOR('',#66383,10.);
#10706=VECTOR('',#66384,10.);
#10707=VECTOR('',#66391,10.);
#10708=VECTOR('',#66392,10.);
#10709=VECTOR('',#66393,10.);
#10710=VECTOR('',#66394,10.);
#10711=VECTOR('',#66399,10.);
#10712=VECTOR('',#66402,10.);
#10713=VECTOR('',#66403,10.);
#10714=VECTOR('',#66410,10.);
#10715=VECTOR('',#66411,10.);
#10716=VECTOR('',#66412,10.);
#10717=VECTOR('',#66413,10.);
#10718=VECTOR('',#66418,10.);
#10719=VECTOR('',#66421,10.);
#10720=VECTOR('',#66422,10.);
#10721=VECTOR('',#66429,10.);
#10722=VECTOR('',#66430,10.);
#10723=VECTOR('',#66431,10.);
#10724=VECTOR('',#66432,10.);
#10725=VECTOR('',#66437,10.);
#10726=VECTOR('',#66440,10.);
#10727=VECTOR('',#66441,10.);
#10728=VECTOR('',#66448,10.);
#10729=VECTOR('',#66449,10.);
#10730=VECTOR('',#66450,10.);
#10731=VECTOR('',#66451,10.);
#10732=VECTOR('',#66456,10.);
#10733=VECTOR('',#66459,10.);
#10734=VECTOR('',#66460,10.);
#10735=VECTOR('',#66467,10.);
#10736=VECTOR('',#66468,10.);
#10737=VECTOR('',#66469,10.);
#10738=VECTOR('',#66470,10.);
#10739=VECTOR('',#66475,10.);
#10740=VECTOR('',#66478,10.);
#10741=VECTOR('',#66479,10.);
#10742=VECTOR('',#66486,10.);
#10743=VECTOR('',#66487,10.);
#10744=VECTOR('',#66488,10.);
#10745=VECTOR('',#66489,10.);
#10746=VECTOR('',#66494,10.);
#10747=VECTOR('',#66497,10.);
#10748=VECTOR('',#66498,10.);
#10749=VECTOR('',#66505,10.);
#10750=VECTOR('',#66506,10.);
#10751=VECTOR('',#66507,10.);
#10752=VECTOR('',#66508,10.);
#10753=VECTOR('',#66513,10.);
#10754=VECTOR('',#66516,10.);
#10755=VECTOR('',#66517,10.);
#10756=VECTOR('',#66524,10.);
#10757=VECTOR('',#66525,10.);
#10758=VECTOR('',#66526,10.);
#10759=VECTOR('',#66527,10.);
#10760=VECTOR('',#66532,10.);
#10761=VECTOR('',#66535,10.);
#10762=VECTOR('',#66536,10.);
#10763=VECTOR('',#66543,10.);
#10764=VECTOR('',#66544,10.);
#10765=VECTOR('',#66545,10.);
#10766=VECTOR('',#66546,10.);
#10767=VECTOR('',#66551,10.);
#10768=VECTOR('',#66554,10.);
#10769=VECTOR('',#66555,10.);
#10770=VECTOR('',#66562,10.);
#10771=VECTOR('',#66563,10.);
#10772=VECTOR('',#66564,10.);
#10773=VECTOR('',#66565,10.);
#10774=VECTOR('',#66570,10.);
#10775=VECTOR('',#66573,10.);
#10776=VECTOR('',#66574,10.);
#10777=VECTOR('',#66581,10.);
#10778=VECTOR('',#66582,10.);
#10779=VECTOR('',#66583,10.);
#10780=VECTOR('',#66584,10.);
#10781=VECTOR('',#66589,10.);
#10782=VECTOR('',#66592,10.);
#10783=VECTOR('',#66593,10.);
#10784=VECTOR('',#66602,10.);
#10785=VECTOR('',#66603,10.);
#10786=VECTOR('',#66606,10.);
#10787=VECTOR('',#66607,10.);
#10788=VECTOR('',#66608,10.);
#10789=VECTOR('',#66611,10.);
#10790=VECTOR('',#66612,10.);
#10791=VECTOR('',#66619,2.);
#10792=VECTOR('',#66624,10.);
#10793=VECTOR('',#66625,10.);
#10794=VECTOR('',#66626,10.);
#10795=VECTOR('',#66627,10.);
#10796=VECTOR('',#66630,10.);
#10797=VECTOR('',#66631,10.);
#10798=VECTOR('',#66632,10.);
#10799=VECTOR('',#66635,10.);
#10800=VECTOR('',#66636,10.);
#10801=VECTOR('',#66637,10.);
#10802=VECTOR('',#66640,10.);
#10803=VECTOR('',#66641,10.);
#10804=VECTOR('',#66642,10.);
#10805=VECTOR('',#66645,10.);
#10806=VECTOR('',#66646,10.);
#10807=VECTOR('',#66647,10.);
#10808=VECTOR('',#66650,10.);
#10809=VECTOR('',#66651,10.);
#10810=VECTOR('',#66660,4.5);
#10811=VECTOR('',#66697,8.);
#10812=VECTOR('',#66740,7.5);
#12903=PLANE('',#54527);
#12904=PLANE('',#54530);
#12905=PLANE('',#54540);
#12906=PLANE('',#54542);
#12907=PLANE('',#54543);
#12908=PLANE('',#54545);
#12909=PLANE('',#54546);
#12910=PLANE('',#54548);
#12911=PLANE('',#54549);
#12912=PLANE('',#54551);
#12913=PLANE('',#54552);
#12914=PLANE('',#54554);
#12915=PLANE('',#54555);
#12916=PLANE('',#54557);
#12917=PLANE('',#54558);
#12918=PLANE('',#54560);
#12919=PLANE('',#54561);
#12920=PLANE('',#54563);
#12921=PLANE('',#54564);
#12922=PLANE('',#54566);
#12923=PLANE('',#54567);
#12924=PLANE('',#54569);
#12925=PLANE('',#54570);
#12926=PLANE('',#54572);
#12927=PLANE('',#54573);
#12928=PLANE('',#54575);
#12929=PLANE('',#54576);
#12930=PLANE('',#54578);
#12931=PLANE('',#54579);
#12932=PLANE('',#54581);
#12933=PLANE('',#54582);
#12934=PLANE('',#54584);
#12935=PLANE('',#54585);
#12936=PLANE('',#54587);
#12937=PLANE('',#54588);
#12938=PLANE('',#54590);
#12939=PLANE('',#54591);
#12940=PLANE('',#54593);
#12941=PLANE('',#54594);
#12942=PLANE('',#54596);
#12943=PLANE('',#54597);
#12944=PLANE('',#54599);
#12945=PLANE('',#54600);
#12946=PLANE('',#54602);
#12947=PLANE('',#54603);
#12948=PLANE('',#54605);
#12949=PLANE('',#54606);
#12950=PLANE('',#54608);
#12951=PLANE('',#54609);
#12952=PLANE('',#54611);
#12953=PLANE('',#54612);
#12954=PLANE('',#54614);
#12955=PLANE('',#54615);
#12956=PLANE('',#54617);
#12957=PLANE('',#54618);
#12958=PLANE('',#54620);
#12959=PLANE('',#54621);
#12960=PLANE('',#54623);
#12961=PLANE('',#54624);
#12962=PLANE('',#54626);
#12963=PLANE('',#54627);
#12964=PLANE('',#54629);
#12965=PLANE('',#54630);
#12966=PLANE('',#54632);
#12967=PLANE('',#54633);
#12968=PLANE('',#54635);
#12969=PLANE('',#54636);
#12970=PLANE('',#54638);
#12971=PLANE('',#54639);
#12972=PLANE('',#54641);
#12973=PLANE('',#54642);
#12974=PLANE('',#54644);
#12975=PLANE('',#54645);
#12976=PLANE('',#54648);
#12977=PLANE('',#54649);
#12978=PLANE('',#54652);
#12979=PLANE('',#54653);
#12980=PLANE('',#54655);
#12981=PLANE('',#54656);
#12982=PLANE('',#54658);
#12983=PLANE('',#54659);
#12984=PLANE('',#54661);
#12985=PLANE('',#54662);
#12986=PLANE('',#54664);
#12987=PLANE('',#54665);
#12988=PLANE('',#54667);
#12989=PLANE('',#54668);
#12990=PLANE('',#54670);
#12991=PLANE('',#54671);
#12992=PLANE('',#54673);
#12993=PLANE('',#54674);
#12994=PLANE('',#54676);
#12995=PLANE('',#54677);
#12996=PLANE('',#54679);
#12997=PLANE('',#54680);
#12998=PLANE('',#54682);
#12999=PLANE('',#54683);
#13000=PLANE('',#54685);
#13001=PLANE('',#54686);
#13002=PLANE('',#54688);
#13003=PLANE('',#54689);
#13004=PLANE('',#54691);
#13005=PLANE('',#54692);
#13006=PLANE('',#54694);
#13007=PLANE('',#54695);
#13008=PLANE('',#54697);
#13009=PLANE('',#54698);
#13010=PLANE('',#54700);
#13011=PLANE('',#54701);
#13012=PLANE('',#54703);
#13013=PLANE('',#54704);
#13014=PLANE('',#54706);
#13015=PLANE('',#54707);
#13016=PLANE('',#54709);
#13017=PLANE('',#54710);
#13018=PLANE('',#54712);
#13019=PLANE('',#54713);
#13020=PLANE('',#54715);
#13021=PLANE('',#54716);
#13022=PLANE('',#54718);
#13023=PLANE('',#54719);
#13024=PLANE('',#54721);
#13025=PLANE('',#54722);
#13026=PLANE('',#54724);
#13027=PLANE('',#54725);
#13028=PLANE('',#54727);
#13029=PLANE('',#54728);
#13030=PLANE('',#54730);
#13031=PLANE('',#54731);
#13032=PLANE('',#54733);
#13033=PLANE('',#54734);
#13034=PLANE('',#54736);
#13035=PLANE('',#54737);
#13036=PLANE('',#54739);
#13037=PLANE('',#54740);
#13038=PLANE('',#54742);
#13039=PLANE('',#54743);
#13040=PLANE('',#54745);
#13041=PLANE('',#54746);
#13042=PLANE('',#54748);
#13043=PLANE('',#54749);
#13044=PLANE('',#54751);
#13045=PLANE('',#54752);
#13046=PLANE('',#54754);
#13047=PLANE('',#54756);
#13048=PLANE('',#54757);
#13049=PLANE('',#54758);
#13050=PLANE('',#54762);
#13051=PLANE('',#54763);
#13052=PLANE('',#54764);
#13053=PLANE('',#54765);
#13054=PLANE('',#54766);
#13055=PLANE('',#54767);
#13056=PLANE('',#54768);
#13057=PLANE('',#54769);
#13058=PLANE('',#54811);
#15414=FACE_OUTER_BOUND('',#18167,.T.);
#15415=FACE_OUTER_BOUND('',#18168,.T.);
#15416=FACE_OUTER_BOUND('',#18169,.T.);
#15417=FACE_OUTER_BOUND('',#18170,.T.);
#15418=FACE_OUTER_BOUND('',#18171,.T.);
#15419=FACE_OUTER_BOUND('',#18172,.T.);
#15420=FACE_OUTER_BOUND('',#18173,.T.);
#15421=FACE_OUTER_BOUND('',#18174,.T.);
#15422=FACE_OUTER_BOUND('',#18175,.T.);
#15423=FACE_OUTER_BOUND('',#18176,.T.);
#15424=FACE_OUTER_BOUND('',#18177,.T.);
#15425=FACE_OUTER_BOUND('',#18178,.T.);
#15426=FACE_OUTER_BOUND('',#18179,.T.);
#15427=FACE_OUTER_BOUND('',#18180,.T.);
#15428=FACE_OUTER_BOUND('',#18181,.T.);
#15429=FACE_OUTER_BOUND('',#18182,.T.);
#15430=FACE_OUTER_BOUND('',#18183,.T.);
#15431=FACE_OUTER_BOUND('',#18184,.T.);
#15432=FACE_OUTER_BOUND('',#18185,.T.);
#15433=FACE_OUTER_BOUND('',#18186,.T.);
#15434=FACE_OUTER_BOUND('',#18187,.T.);
#15435=FACE_OUTER_BOUND('',#18188,.T.);
#15436=FACE_OUTER_BOUND('',#18189,.T.);
#15437=FACE_OUTER_BOUND('',#18190,.T.);
#15438=FACE_OUTER_BOUND('',#18191,.T.);
#15439=FACE_OUTER_BOUND('',#18192,.T.);
#15440=FACE_OUTER_BOUND('',#18193,.T.);
#15441=FACE_OUTER_BOUND('',#18194,.T.);
#15442=FACE_OUTER_BOUND('',#18195,.T.);
#15443=FACE_OUTER_BOUND('',#18196,.T.);
#15444=FACE_OUTER_BOUND('',#18197,.T.);
#15445=FACE_OUTER_BOUND('',#18198,.T.);
#15446=FACE_OUTER_BOUND('',#18199,.T.);
#15447=FACE_OUTER_BOUND('',#18200,.T.);
#15448=FACE_OUTER_BOUND('',#18201,.T.);
#15449=FACE_OUTER_BOUND('',#18202,.T.);
#15450=FACE_OUTER_BOUND('',#18203,.T.);
#15451=FACE_OUTER_BOUND('',#18204,.T.);
#15452=FACE_OUTER_BOUND('',#18205,.T.);
#15453=FACE_OUTER_BOUND('',#18206,.T.);
#15454=FACE_OUTER_BOUND('',#18208,.T.);
#15455=FACE_OUTER_BOUND('',#18209,.T.);
#15456=FACE_OUTER_BOUND('',#18210,.T.);
#15457=FACE_OUTER_BOUND('',#18211,.T.);
#15458=FACE_OUTER_BOUND('',#18212,.T.);
#15459=FACE_OUTER_BOUND('',#18213,.T.);
#15460=FACE_OUTER_BOUND('',#18214,.T.);
#15461=FACE_OUTER_BOUND('',#18215,.T.);
#15462=FACE_OUTER_BOUND('',#18216,.T.);
#15463=FACE_OUTER_BOUND('',#18217,.T.);
#15464=FACE_OUTER_BOUND('',#18218,.T.);
#15465=FACE_OUTER_BOUND('',#18219,.T.);
#15466=FACE_OUTER_BOUND('',#18220,.T.);
#15467=FACE_OUTER_BOUND('',#18221,.T.);
#15468=FACE_OUTER_BOUND('',#18222,.T.);
#15469=FACE_OUTER_BOUND('',#18223,.T.);
#15470=FACE_OUTER_BOUND('',#18224,.T.);
#15471=FACE_OUTER_BOUND('',#18225,.T.);
#15472=FACE_OUTER_BOUND('',#18226,.T.);
#15473=FACE_OUTER_BOUND('',#18227,.T.);
#15474=FACE_OUTER_BOUND('',#18228,.T.);
#15475=FACE_OUTER_BOUND('',#18229,.T.);
#15476=FACE_OUTER_BOUND('',#18230,.T.);
#15477=FACE_OUTER_BOUND('',#18231,.T.);
#15478=FACE_OUTER_BOUND('',#18232,.T.);
#15479=FACE_OUTER_BOUND('',#18233,.T.);
#15480=FACE_OUTER_BOUND('',#18234,.T.);
#15481=FACE_OUTER_BOUND('',#18235,.T.);
#15482=FACE_OUTER_BOUND('',#18236,.T.);
#15483=FACE_OUTER_BOUND('',#18237,.T.);
#15484=FACE_OUTER_BOUND('',#18238,.T.);
#15485=FACE_OUTER_BOUND('',#18239,.T.);
#15486=FACE_OUTER_BOUND('',#18240,.T.);
#15487=FACE_OUTER_BOUND('',#18241,.T.);
#15488=FACE_OUTER_BOUND('',#18242,.T.);
#15489=FACE_OUTER_BOUND('',#18243,.T.);
#15490=FACE_OUTER_BOUND('',#18244,.T.);
#15491=FACE_OUTER_BOUND('',#18245,.T.);
#15492=FACE_OUTER_BOUND('',#18246,.T.);
#15493=FACE_OUTER_BOUND('',#18247,.T.);
#15494=FACE_OUTER_BOUND('',#18248,.T.);
#15495=FACE_OUTER_BOUND('',#18249,.T.);
#15496=FACE_OUTER_BOUND('',#18250,.T.);
#15497=FACE_OUTER_BOUND('',#18251,.T.);
#15498=FACE_OUTER_BOUND('',#18252,.T.);
#15499=FACE_OUTER_BOUND('',#18253,.T.);
#15500=FACE_OUTER_BOUND('',#18254,.T.);
#15501=FACE_OUTER_BOUND('',#18255,.T.);
#15502=FACE_OUTER_BOUND('',#18256,.T.);
#15503=FACE_OUTER_BOUND('',#18257,.T.);
#15504=FACE_OUTER_BOUND('',#18258,.T.);
#15505=FACE_OUTER_BOUND('',#18259,.T.);
#15506=FACE_OUTER_BOUND('',#18260,.T.);
#15507=FACE_OUTER_BOUND('',#18261,.T.);
#15508=FACE_OUTER_BOUND('',#18262,.T.);
#15509=FACE_OUTER_BOUND('',#18263,.T.);
#15510=FACE_OUTER_BOUND('',#18264,.T.);
#15511=FACE_OUTER_BOUND('',#18265,.T.);
#15512=FACE_OUTER_BOUND('',#18266,.T.);
#15513=FACE_OUTER_BOUND('',#18267,.T.);
#15514=FACE_OUTER_BOUND('',#18268,.T.);
#15515=FACE_OUTER_BOUND('',#18269,.T.);
#15516=FACE_OUTER_BOUND('',#18270,.T.);
#15517=FACE_OUTER_BOUND('',#18271,.T.);
#15518=FACE_OUTER_BOUND('',#18272,.T.);
#15519=FACE_OUTER_BOUND('',#18273,.T.);
#15520=FACE_OUTER_BOUND('',#18274,.T.);
#15521=FACE_OUTER_BOUND('',#18275,.T.);
#15522=FACE_OUTER_BOUND('',#18276,.T.);
#15523=FACE_OUTER_BOUND('',#18277,.T.);
#15524=FACE_OUTER_BOUND('',#18278,.T.);
#15525=FACE_OUTER_BOUND('',#18279,.T.);
#15526=FACE_OUTER_BOUND('',#18280,.T.);
#15527=FACE_OUTER_BOUND('',#18281,.T.);
#15528=FACE_OUTER_BOUND('',#18282,.T.);
#15529=FACE_OUTER_BOUND('',#18283,.T.);
#15530=FACE_OUTER_BOUND('',#18284,.T.);
#15531=FACE_OUTER_BOUND('',#18285,.T.);
#15532=FACE_OUTER_BOUND('',#18286,.T.);
#15533=FACE_OUTER_BOUND('',#18287,.T.);
#15534=FACE_OUTER_BOUND('',#18288,.T.);
#15535=FACE_OUTER_BOUND('',#18289,.T.);
#15536=FACE_OUTER_BOUND('',#18290,.T.);
#15537=FACE_OUTER_BOUND('',#18291,.T.);
#15538=FACE_OUTER_BOUND('',#18292,.T.);
#15539=FACE_OUTER_BOUND('',#18293,.T.);
#15540=FACE_OUTER_BOUND('',#18294,.T.);
#15541=FACE_OUTER_BOUND('',#18295,.T.);
#15542=FACE_OUTER_BOUND('',#18296,.T.);
#15543=FACE_OUTER_BOUND('',#18297,.T.);
#15544=FACE_OUTER_BOUND('',#18298,.T.);
#15545=FACE_OUTER_BOUND('',#18299,.T.);
#15546=FACE_OUTER_BOUND('',#18300,.T.);
#15547=FACE_OUTER_BOUND('',#18301,.T.);
#15548=FACE_OUTER_BOUND('',#18302,.T.);
#15549=FACE_OUTER_BOUND('',#18303,.T.);
#15550=FACE_OUTER_BOUND('',#18304,.T.);
#15551=FACE_OUTER_BOUND('',#18305,.T.);
#15552=FACE_OUTER_BOUND('',#18306,.T.);
#15553=FACE_OUTER_BOUND('',#18307,.T.);
#15554=FACE_OUTER_BOUND('',#18308,.T.);
#15555=FACE_OUTER_BOUND('',#18309,.T.);
#15556=FACE_OUTER_BOUND('',#18310,.T.);
#15557=FACE_OUTER_BOUND('',#18311,.T.);
#15558=FACE_OUTER_BOUND('',#18312,.T.);
#15559=FACE_OUTER_BOUND('',#18313,.T.);
#15560=FACE_OUTER_BOUND('',#18314,.T.);
#15561=FACE_OUTER_BOUND('',#18315,.T.);
#15562=FACE_OUTER_BOUND('',#18316,.T.);
#15563=FACE_OUTER_BOUND('',#18317,.T.);
#15564=FACE_OUTER_BOUND('',#18318,.T.);
#15565=FACE_OUTER_BOUND('',#18319,.T.);
#15566=FACE_OUTER_BOUND('',#18320,.T.);
#15567=FACE_OUTER_BOUND('',#18321,.T.);
#15568=FACE_OUTER_BOUND('',#18322,.T.);
#15569=FACE_OUTER_BOUND('',#18323,.T.);
#15570=FACE_OUTER_BOUND('',#18324,.T.);
#15571=FACE_OUTER_BOUND('',#18325,.T.);
#15572=FACE_OUTER_BOUND('',#18326,.T.);
#15573=FACE_OUTER_BOUND('',#18327,.T.);
#15574=FACE_OUTER_BOUND('',#18328,.T.);
#15575=FACE_OUTER_BOUND('',#18329,.T.);
#15576=FACE_OUTER_BOUND('',#18330,.T.);
#15577=FACE_OUTER_BOUND('',#18331,.T.);
#15578=FACE_OUTER_BOUND('',#18332,.T.);
#15579=FACE_OUTER_BOUND('',#18333,.T.);
#15580=FACE_OUTER_BOUND('',#18334,.T.);
#15581=FACE_OUTER_BOUND('',#18335,.T.);
#15582=FACE_OUTER_BOUND('',#18336,.T.);
#15583=FACE_OUTER_BOUND('',#18337,.T.);
#15584=FACE_OUTER_BOUND('',#18338,.T.);
#15585=FACE_OUTER_BOUND('',#18339,.T.);
#15586=FACE_OUTER_BOUND('',#18340,.T.);
#15587=FACE_OUTER_BOUND('',#18341,.T.);
#15588=FACE_OUTER_BOUND('',#18342,.T.);
#15589=FACE_OUTER_BOUND('',#18343,.T.);
#15590=FACE_OUTER_BOUND('',#18344,.T.);
#15591=FACE_OUTER_BOUND('',#18345,.T.);
#15592=FACE_OUTER_BOUND('',#18346,.T.);
#15593=FACE_OUTER_BOUND('',#18347,.T.);
#15594=FACE_OUTER_BOUND('',#18348,.T.);
#15595=FACE_OUTER_BOUND('',#18349,.T.);
#15596=FACE_OUTER_BOUND('',#18350,.T.);
#15597=FACE_OUTER_BOUND('',#18351,.T.);
#15598=FACE_OUTER_BOUND('',#18352,.T.);
#15599=FACE_OUTER_BOUND('',#18353,.T.);
#15600=FACE_OUTER_BOUND('',#18354,.T.);
#15601=FACE_OUTER_BOUND('',#18355,.T.);
#15602=FACE_OUTER_BOUND('',#18356,.T.);
#15603=FACE_OUTER_BOUND('',#18357,.T.);
#15604=FACE_OUTER_BOUND('',#18358,.T.);
#15605=FACE_OUTER_BOUND('',#18359,.T.);
#15606=FACE_OUTER_BOUND('',#18361,.T.);
#15607=FACE_OUTER_BOUND('',#18362,.T.);
#15608=FACE_OUTER_BOUND('',#18363,.T.);
#15609=FACE_OUTER_BOUND('',#18364,.T.);
#15610=FACE_OUTER_BOUND('',#18365,.T.);
#18167=EDGE_LOOP('',(#45503,#45504,#45505,#45506));
#18168=EDGE_LOOP('',(#45507,#45508,#45509,#45510));
#18169=EDGE_LOOP('',(#45511,#45512,#45513,#45514));
#18170=EDGE_LOOP('',(#45515,#45516,#45517,#45518));
#18171=EDGE_LOOP('',(#45519,#45520,#45521,#45522));
#18172=EDGE_LOOP('',(#45523,#45524,#45525,#45526));
#18173=EDGE_LOOP('',(#45527,#45528,#45529,#45530));
#18174=EDGE_LOOP('',(#45531,#45532,#45533,#45534));
#18175=EDGE_LOOP('',(#45535,#45536,#45537,#45538));
#18176=EDGE_LOOP('',(#45539,#45540,#45541,#45542));
#18177=EDGE_LOOP('',(#45543,#45544,#45545,#45546));
#18178=EDGE_LOOP('',(#45547,#45548,#45549,#45550));
#18179=EDGE_LOOP('',(#45551,#45552,#45553,#45554));
#18180=EDGE_LOOP('',(#45555,#45556,#45557,#45558));
#18181=EDGE_LOOP('',(#45559,#45560,#45561,#45562));
#18182=EDGE_LOOP('',(#45563,#45564,#45565,#45566));
#18183=EDGE_LOOP('',(#45567,#45568,#45569));
#18184=EDGE_LOOP('',(#45570,#45571,#45572,#45573,#45574));
#18185=EDGE_LOOP('',(#45575,#45576,#45577,#45578));
#18186=EDGE_LOOP('',(#45579,#45580,#45581,#45582));
#18187=EDGE_LOOP('',(#45583,#45584,#45585,#45586));
#18188=EDGE_LOOP('',(#45587,#45588,#45589,#45590));
#18189=EDGE_LOOP('',(#45591,#45592,#45593,#45594));
#18190=EDGE_LOOP('',(#45595,#45596,#45597,#45598));
#18191=EDGE_LOOP('',(#45599,#45600,#45601,#45602));
#18192=EDGE_LOOP('',(#45603,#45604,#45605,#45606));
#18193=EDGE_LOOP('',(#45607,#45608,#45609,#45610));
#18194=EDGE_LOOP('',(#45611,#45612,#45613,#45614));
#18195=EDGE_LOOP('',(#45615,#45616,#45617,#45618));
#18196=EDGE_LOOP('',(#45619,#45620,#45621,#45622));
#18197=EDGE_LOOP('',(#45623,#45624,#45625,#45626));
#18198=EDGE_LOOP('',(#45627,#45628,#45629,#45630));
#18199=EDGE_LOOP('',(#45631,#45632,#45633,#45634,#45635,#45636));
#18200=EDGE_LOOP('',(#45637,#45638,#45639,#45640,#45641,#45642,#45643,#45644,
#45645,#45646,#45647,#45648,#45649,#45650,#45651,#45652,#45653,#45654,#45655,
#45656,#45657,#45658,#45659,#45660,#45661,#45662,#45663,#45664,#45665,#45666,
#45667,#45668,#45669,#45670,#45671));
#18201=EDGE_LOOP('',(#45672,#45673,#45674,#45675,#45676));
#18202=EDGE_LOOP('',(#45677,#45678,#45679,#45680));
#18203=EDGE_LOOP('',(#45681,#45682,#45683,#45684,#45685,#45686,#45687,#45688,
#45689,#45690,#45691,#45692,#45693,#45694,#45695,#45696,#45697,#45698,#45699,
#45700,#45701,#45702,#45703,#45704,#45705,#45706,#45707,#45708,#45709,#45710,
#45711,#45712,#45713,#45714,#45715,#45716));
#18204=EDGE_LOOP('',(#45717,#45718,#45719,#45720,#45721,#45722));
#18205=EDGE_LOOP('',(#45723,#45724,#45725,#45726));
#18206=EDGE_LOOP('',(#45727));
#18207=EDGE_LOOP('',(#45728));
#18208=EDGE_LOOP('',(#45729,#45730,#45731,#45732));
#18209=EDGE_LOOP('',(#45733,#45734,#45735));
#18210=EDGE_LOOP('',(#45736,#45737,#45738,#45739));
#18211=EDGE_LOOP('',(#45740,#45741,#45742));
#18212=EDGE_LOOP('',(#45743,#45744,#45745,#45746));
#18213=EDGE_LOOP('',(#45747,#45748,#45749));
#18214=EDGE_LOOP('',(#45750,#45751,#45752,#45753));
#18215=EDGE_LOOP('',(#45754,#45755,#45756));
#18216=EDGE_LOOP('',(#45757,#45758,#45759,#45760));
#18217=EDGE_LOOP('',(#45761,#45762,#45763));
#18218=EDGE_LOOP('',(#45764,#45765,#45766,#45767));
#18219=EDGE_LOOP('',(#45768,#45769,#45770));
#18220=EDGE_LOOP('',(#45771,#45772,#45773,#45774));
#18221=EDGE_LOOP('',(#45775,#45776,#45777));
#18222=EDGE_LOOP('',(#45778,#45779,#45780,#45781));
#18223=EDGE_LOOP('',(#45782,#45783,#45784));
#18224=EDGE_LOOP('',(#45785,#45786,#45787,#45788));
#18225=EDGE_LOOP('',(#45789,#45790,#45791));
#18226=EDGE_LOOP('',(#45792,#45793,#45794,#45795));
#18227=EDGE_LOOP('',(#45796,#45797,#45798));
#18228=EDGE_LOOP('',(#45799,#45800,#45801,#45802));
#18229=EDGE_LOOP('',(#45803,#45804,#45805));
#18230=EDGE_LOOP('',(#45806,#45807,#45808,#45809));
#18231=EDGE_LOOP('',(#45810,#45811,#45812));
#18232=EDGE_LOOP('',(#45813,#45814,#45815,#45816));
#18233=EDGE_LOOP('',(#45817,#45818,#45819));
#18234=EDGE_LOOP('',(#45820,#45821,#45822,#45823));
#18235=EDGE_LOOP('',(#45824,#45825,#45826));
#18236=EDGE_LOOP('',(#45827,#45828,#45829,#45830));
#18237=EDGE_LOOP('',(#45831,#45832,#45833));
#18238=EDGE_LOOP('',(#45834,#45835,#45836,#45837));
#18239=EDGE_LOOP('',(#45838,#45839,#45840));
#18240=EDGE_LOOP('',(#45841,#45842,#45843,#45844));
#18241=EDGE_LOOP('',(#45845,#45846,#45847));
#18242=EDGE_LOOP('',(#45848,#45849,#45850,#45851));
#18243=EDGE_LOOP('',(#45852,#45853,#45854));
#18244=EDGE_LOOP('',(#45855,#45856,#45857,#45858));
#18245=EDGE_LOOP('',(#45859,#45860,#45861));
#18246=EDGE_LOOP('',(#45862,#45863,#45864,#45865));
#18247=EDGE_LOOP('',(#45866,#45867,#45868));
#18248=EDGE_LOOP('',(#45869,#45870,#45871,#45872));
#18249=EDGE_LOOP('',(#45873,#45874,#45875));
#18250=EDGE_LOOP('',(#45876,#45877,#45878,#45879));
#18251=EDGE_LOOP('',(#45880,#45881,#45882));
#18252=EDGE_LOOP('',(#45883,#45884,#45885,#45886));
#18253=EDGE_LOOP('',(#45887,#45888,#45889));
#18254=EDGE_LOOP('',(#45890,#45891,#45892,#45893));
#18255=EDGE_LOOP('',(#45894,#45895,#45896));
#18256=EDGE_LOOP('',(#45897,#45898,#45899,#45900));
#18257=EDGE_LOOP('',(#45901,#45902,#45903));
#18258=EDGE_LOOP('',(#45904,#45905,#45906,#45907));
#18259=EDGE_LOOP('',(#45908,#45909,#45910));
#18260=EDGE_LOOP('',(#45911,#45912,#45913,#45914));
#18261=EDGE_LOOP('',(#45915,#45916,#45917));
#18262=EDGE_LOOP('',(#45918,#45919,#45920,#45921));
#18263=EDGE_LOOP('',(#45922,#45923,#45924));
#18264=EDGE_LOOP('',(#45925,#45926,#45927,#45928));
#18265=EDGE_LOOP('',(#45929,#45930,#45931));
#18266=EDGE_LOOP('',(#45932,#45933,#45934,#45935));
#18267=EDGE_LOOP('',(#45936,#45937,#45938));
#18268=EDGE_LOOP('',(#45939,#45940,#45941,#45942));
#18269=EDGE_LOOP('',(#45943,#45944,#45945));
#18270=EDGE_LOOP('',(#45946,#45947,#45948,#45949));
#18271=EDGE_LOOP('',(#45950,#45951,#45952));
#18272=EDGE_LOOP('',(#45953,#45954,#45955,#45956));
#18273=EDGE_LOOP('',(#45957,#45958,#45959));
#18274=EDGE_LOOP('',(#45960,#45961,#45962,#45963));
#18275=EDGE_LOOP('',(#45964,#45965,#45966));
#18276=EDGE_LOOP('',(#45967,#45968,#45969,#45970));
#18277=EDGE_LOOP('',(#45971,#45972,#45973,#45974));
#18278=EDGE_LOOP('',(#45975,#45976,#45977,#45978));
#18279=EDGE_LOOP('',(#45979,#45980,#45981,#45982));
#18280=EDGE_LOOP('',(#45983,#45984,#45985,#45986));
#18281=EDGE_LOOP('',(#45987,#45988,#45989));
#18282=EDGE_LOOP('',(#45990,#45991,#45992,#45993));
#18283=EDGE_LOOP('',(#45994,#45995,#45996));
#18284=EDGE_LOOP('',(#45997,#45998,#45999,#46000));
#18285=EDGE_LOOP('',(#46001,#46002,#46003));
#18286=EDGE_LOOP('',(#46004,#46005,#46006,#46007));
#18287=EDGE_LOOP('',(#46008,#46009,#46010));
#18288=EDGE_LOOP('',(#46011,#46012,#46013,#46014));
#18289=EDGE_LOOP('',(#46015,#46016,#46017));
#18290=EDGE_LOOP('',(#46018,#46019,#46020,#46021));
#18291=EDGE_LOOP('',(#46022,#46023,#46024));
#18292=EDGE_LOOP('',(#46025,#46026,#46027,#46028));
#18293=EDGE_LOOP('',(#46029,#46030,#46031));
#18294=EDGE_LOOP('',(#46032,#46033,#46034,#46035));
#18295=EDGE_LOOP('',(#46036,#46037,#46038));
#18296=EDGE_LOOP('',(#46039,#46040,#46041,#46042));
#18297=EDGE_LOOP('',(#46043,#46044,#46045));
#18298=EDGE_LOOP('',(#46046,#46047,#46048,#46049));
#18299=EDGE_LOOP('',(#46050,#46051,#46052));
#18300=EDGE_LOOP('',(#46053,#46054,#46055,#46056));
#18301=EDGE_LOOP('',(#46057,#46058,#46059));
#18302=EDGE_LOOP('',(#46060,#46061,#46062,#46063));
#18303=EDGE_LOOP('',(#46064,#46065,#46066));
#18304=EDGE_LOOP('',(#46067,#46068,#46069,#46070));
#18305=EDGE_LOOP('',(#46071,#46072,#46073));
#18306=EDGE_LOOP('',(#46074,#46075,#46076,#46077));
#18307=EDGE_LOOP('',(#46078,#46079,#46080));
#18308=EDGE_LOOP('',(#46081,#46082,#46083,#46084));
#18309=EDGE_LOOP('',(#46085,#46086,#46087));
#18310=EDGE_LOOP('',(#46088,#46089,#46090,#46091));
#18311=EDGE_LOOP('',(#46092,#46093,#46094));
#18312=EDGE_LOOP('',(#46095,#46096,#46097,#46098));
#18313=EDGE_LOOP('',(#46099,#46100,#46101));
#18314=EDGE_LOOP('',(#46102,#46103,#46104,#46105));
#18315=EDGE_LOOP('',(#46106,#46107,#46108));
#18316=EDGE_LOOP('',(#46109,#46110,#46111,#46112));
#18317=EDGE_LOOP('',(#46113,#46114,#46115));
#18318=EDGE_LOOP('',(#46116,#46117,#46118,#46119));
#18319=EDGE_LOOP('',(#46120,#46121,#46122));
#18320=EDGE_LOOP('',(#46123,#46124,#46125,#46126));
#18321=EDGE_LOOP('',(#46127,#46128,#46129));
#18322=EDGE_LOOP('',(#46130,#46131,#46132,#46133));
#18323=EDGE_LOOP('',(#46134,#46135,#46136));
#18324=EDGE_LOOP('',(#46137,#46138,#46139,#46140));
#18325=EDGE_LOOP('',(#46141,#46142,#46143));
#18326=EDGE_LOOP('',(#46144,#46145,#46146,#46147));
#18327=EDGE_LOOP('',(#46148,#46149,#46150));
#18328=EDGE_LOOP('',(#46151,#46152,#46153,#46154));
#18329=EDGE_LOOP('',(#46155,#46156,#46157));
#18330=EDGE_LOOP('',(#46158,#46159,#46160,#46161));
#18331=EDGE_LOOP('',(#46162,#46163,#46164));
#18332=EDGE_LOOP('',(#46165,#46166,#46167,#46168));
#18333=EDGE_LOOP('',(#46169,#46170,#46171));
#18334=EDGE_LOOP('',(#46172,#46173,#46174,#46175));
#18335=EDGE_LOOP('',(#46176,#46177,#46178));
#18336=EDGE_LOOP('',(#46179,#46180,#46181,#46182));
#18337=EDGE_LOOP('',(#46183,#46184,#46185));
#18338=EDGE_LOOP('',(#46186,#46187,#46188,#46189));
#18339=EDGE_LOOP('',(#46190,#46191,#46192));
#18340=EDGE_LOOP('',(#46193,#46194,#46195,#46196));
#18341=EDGE_LOOP('',(#46197,#46198,#46199));
#18342=EDGE_LOOP('',(#46200,#46201,#46202,#46203));
#18343=EDGE_LOOP('',(#46204,#46205,#46206));
#18344=EDGE_LOOP('',(#46207,#46208,#46209,#46210));
#18345=EDGE_LOOP('',(#46211,#46212,#46213));
#18346=EDGE_LOOP('',(#46214,#46215,#46216,#46217));
#18347=EDGE_LOOP('',(#46218,#46219,#46220));
#18348=EDGE_LOOP('',(#46221,#46222,#46223));
#18349=EDGE_LOOP('',(#46224,#46225,#46226,#46227));
#18350=EDGE_LOOP('',(#46228,#46229,#46230,#46231));
#18351=EDGE_LOOP('',(#46232,#46233,#46234));
#18352=EDGE_LOOP('',(#46235,#46236,#46237));
#18353=EDGE_LOOP('',(#46238,#46239,#46240,#46241));
#18354=EDGE_LOOP('',(#46242,#46243,#46244,#46245));
#18355=EDGE_LOOP('',(#46246,#46247,#46248,#46249));
#18356=EDGE_LOOP('',(#46250,#46251,#46252,#46253));
#18357=EDGE_LOOP('',(#46254,#46255,#46256,#46257));
#18358=EDGE_LOOP('',(#46258,#46259,#46260,#46261));
#18359=EDGE_LOOP('',(#46262,#46263,#46264,#46265,#46266,#46267));
#18360=EDGE_LOOP('',(#46268));
#18361=EDGE_LOOP('',(#46269));
#18362=EDGE_LOOP('',(#46270,#46271,#46272,#46273,#46274,#46275));
#18363=EDGE_LOOP('',(#46276,#46277,#46278,#46279,#46280,#46281,#46282,#46283,
#46284,#46285,#46286,#46287,#46288,#46289,#46290,#46291,#46292,#46293,#46294,
#46295,#46296,#46297,#46298,#46299,#46300,#46301,#46302,#46303,#46304,#46305,
#46306,#46307,#46308,#46309,#46310,#46311,#46312,#46313,#46314,#46315,#46316,
#46317,#46318,#46319,#46320,#46321,#46322,#46323,#46324,#46325,#46326,#46327,
#46328,#46329,#46330,#46331,#46332,#46333,#46334,#46335,#46336,#46337,#46338,
#46339,#46340,#46341,#46342,#46343,#46344,#46345,#46346,#46347,#46348,#46349,
#46350,#46351,#46352,#46353,#46354,#46355,#46356,#46357,#46358,#46359,#46360,
#46361,#46362,#46363,#46364,#46365,#46366,#46367,#46368,#46369,#46370,#46371,
#46372,#46373,#46374,#46375,#46376,#46377,#46378,#46379,#46380,#46381,#46382,
#46383,#46384,#46385,#46386,#46387,#46388,#46389,#46390,#46391,#46392,#46393,
#46394,#46395,#46396,#46397,#46398,#46399,#46400,#46401,#46402,#46403,#46404,
#46405,#46406,#46407,#46408,#46409,#46410,#46411,#46412,#46413,#46414,#46415,
#46416,#46417,#46418,#46419,#46420,#46421,#46422,#46423));
#18364=EDGE_LOOP('',(#46424,#46425,#46426,#46427,#46428,#46429,#46430,#46431,
#46432,#46433,#46434,#46435,#46436,#46437,#46438,#46439,#46440,#46441,#46442,
#46443,#46444,#46445,#46446,#46447,#46448,#46449,#46450,#46451,#46452,#46453,
#46454,#46455,#46456,#46457,#46458,#46459,#46460,#46461,#46462,#46463,#46464,
#46465,#46466,#46467,#46468,#46469,#46470,#46471,#46472,#46473,#46474,#46475,
#46476,#46477,#46478,#46479,#46480,#46481,#46482,#46483,#46484,#46485,#46486,
#46487,#46488,#46489,#46490,#46491,#46492,#46493,#46494,#46495,#46496,#46497,
#46498,#46499));
#18365=EDGE_LOOP('',(#46500));
#18366=EDGE_LOOP('',(#46501,#46502,#46503,#46504,#46505,#46506));
#20009=CIRCLE('',#54493,4.925);
#20010=CIRCLE('',#54510,4.0705);
#20011=CIRCLE('',#54512,4.0705);
#20012=CIRCLE('',#54528,4.925);
#20013=CIRCLE('',#54529,4.925);
#20014=CIRCLE('',#54531,4.925);
#20015=CIRCLE('',#54532,4.925);
#20016=CIRCLE('',#54533,4.0705);
#20017=CIRCLE('',#54536,0.4);
#20018=CIRCLE('',#54537,5.325);
#20019=CIRCLE('',#54538,4.925);
#20020=CIRCLE('',#54541,8.);
#20021=CIRCLE('',#54544,8.);
#20022=CIRCLE('',#54547,8.);
#20023=CIRCLE('',#54550,8.);
#20024=CIRCLE('',#54553,8.);
#20025=CIRCLE('',#54556,8.);
#20026=CIRCLE('',#54559,8.);
#20027=CIRCLE('',#54562,8.);
#20028=CIRCLE('',#54565,8.);
#20029=CIRCLE('',#54568,8.);
#20030=CIRCLE('',#54571,8.);
#20031=CIRCLE('',#54574,8.);
#20032=CIRCLE('',#54577,8.);
#20033=CIRCLE('',#54580,8.);
#20034=CIRCLE('',#54583,8.);
#20035=CIRCLE('',#54586,8.);
#20036=CIRCLE('',#54589,8.);
#20037=CIRCLE('',#54592,8.);
#20038=CIRCLE('',#54595,8.);
#20039=CIRCLE('',#54598,8.);
#20040=CIRCLE('',#54601,8.);
#20041=CIRCLE('',#54604,8.);
#20042=CIRCLE('',#54607,8.);
#20043=CIRCLE('',#54610,8.);
#20044=CIRCLE('',#54613,8.);
#20045=CIRCLE('',#54616,8.);
#20046=CIRCLE('',#54619,8.);
#20047=CIRCLE('',#54622,8.);
#20048=CIRCLE('',#54625,8.);
#20049=CIRCLE('',#54628,8.);
#20050=CIRCLE('',#54631,8.);
#20051=CIRCLE('',#54634,8.);
#20052=CIRCLE('',#54637,8.);
#20053=CIRCLE('',#54640,8.);
#20054=CIRCLE('',#54643,8.);
#20055=CIRCLE('',#54646,8.);
#20056=CIRCLE('',#54647,8.);
#20057=CIRCLE('',#54650,8.);
#20058=CIRCLE('',#54651,8.);
#20059=CIRCLE('',#54654,8.);
#20060=CIRCLE('',#54657,8.);
#20061=CIRCLE('',#54660,8.);
#20062=CIRCLE('',#54663,8.);
#20063=CIRCLE('',#54666,8.);
#20064=CIRCLE('',#54669,8.);
#20065=CIRCLE('',#54672,8.);
#20066=CIRCLE('',#54675,8.);
#20067=CIRCLE('',#54678,8.);
#20068=CIRCLE('',#54681,8.);
#20069=CIRCLE('',#54684,8.);
#20070=CIRCLE('',#54687,8.);
#20071=CIRCLE('',#54690,8.);
#20072=CIRCLE('',#54693,8.);
#20073=CIRCLE('',#54696,8.);
#20074=CIRCLE('',#54699,8.);
#20075=CIRCLE('',#54702,8.);
#20076=CIRCLE('',#54705,8.);
#20077=CIRCLE('',#54708,8.);
#20078=CIRCLE('',#54711,8.);
#20079=CIRCLE('',#54714,8.);
#20080=CIRCLE('',#54717,8.);
#20081=CIRCLE('',#54720,8.);
#20082=CIRCLE('',#54723,8.);
#20083=CIRCLE('',#54726,8.);
#20084=CIRCLE('',#54729,8.);
#20085=CIRCLE('',#54732,8.);
#20086=CIRCLE('',#54735,8.);
#20087=CIRCLE('',#54738,8.);
#20088=CIRCLE('',#54741,8.);
#20089=CIRCLE('',#54744,8.);
#20090=CIRCLE('',#54747,8.);
#20091=CIRCLE('',#54750,8.);
#20092=CIRCLE('',#54753,8.);
#20093=CIRCLE('',#54755,8.);
#20094=CIRCLE('',#54759,8.);
#20095=CIRCLE('',#54761,3.98342616391485);
#20096=CIRCLE('',#54770,4.);
#20097=CIRCLE('',#54773,8.);
#20098=CIRCLE('',#54774,8.);
#20099=CIRCLE('',#54775,8.);
#20100=CIRCLE('',#54776,8.);
#20101=CIRCLE('',#54777,8.);
#20102=CIRCLE('',#54778,8.);
#20103=CIRCLE('',#54779,8.);
#20104=CIRCLE('',#54780,8.);
#20105=CIRCLE('',#54781,8.);
#20106=CIRCLE('',#54782,8.);
#20107=CIRCLE('',#54783,8.);
#20108=CIRCLE('',#54784,8.);
#20109=CIRCLE('',#54785,8.);
#20110=CIRCLE('',#54786,8.);
#20111=CIRCLE('',#54787,8.);
#20112=CIRCLE('',#54788,8.);
#20113=CIRCLE('',#54789,8.);
#20114=CIRCLE('',#54790,8.);
#20115=CIRCLE('',#54791,8.);
#20116=CIRCLE('',#54792,8.);
#20117=CIRCLE('',#54793,8.);
#20118=CIRCLE('',#54794,8.);
#20119=CIRCLE('',#54795,8.);
#20120=CIRCLE('',#54796,8.);
#20121=CIRCLE('',#54797,8.);
#20122=CIRCLE('',#54798,8.);
#20123=CIRCLE('',#54799,8.);
#20124=CIRCLE('',#54800,8.);
#20125=CIRCLE('',#54801,8.);
#20126=CIRCLE('',#54802,8.);
#20127=CIRCLE('',#54803,8.);
#20128=CIRCLE('',#54804,8.);
#20129=CIRCLE('',#54805,8.);
#20130=CIRCLE('',#54806,8.);
#20131=CIRCLE('',#54807,8.);
#20132=CIRCLE('',#54808,8.);
#20133=CIRCLE('',#54810,7.);
#24506=VERTEX_POINT('',#84083);
#24507=VERTEX_POINT('',#84084);
#24508=VERTEX_POINT('',#84086);
#24509=VERTEX_POINT('',#84097);
#24510=VERTEX_POINT('',#84110);
#24511=VERTEX_POINT('',#84111);
#24512=VERTEX_POINT('',#84158);
#24513=VERTEX_POINT('',#84159);
#24514=VERTEX_POINT('',#84206);
#24515=VERTEX_POINT('',#84207);
#24516=VERTEX_POINT('',#84260);
#24517=VERTEX_POINT('',#84261);
#24518=VERTEX_POINT('',#84308);
#24519=VERTEX_POINT('',#84309);
#24520=VERTEX_POINT('',#84356);
#24521=VERTEX_POINT('',#84357);
#24522=VERTEX_POINT('',#84410);
#24523=VERTEX_POINT('',#84411);
#24524=VERTEX_POINT('',#84458);
#24525=VERTEX_POINT('',#84459);
#24526=VERTEX_POINT('',#84506);
#24527=VERTEX_POINT('',#84507);
#24528=VERTEX_POINT('',#84560);
#24529=VERTEX_POINT('',#84561);
#24530=VERTEX_POINT('',#84608);
#24531=VERTEX_POINT('',#84609);
#24532=VERTEX_POINT('',#84656);
#24533=VERTEX_POINT('',#84657);
#24534=VERTEX_POINT('',#84710);
#24535=VERTEX_POINT('',#84711);
#24536=VERTEX_POINT('',#84758);
#24537=VERTEX_POINT('',#84759);
#24538=VERTEX_POINT('',#84806);
#24539=VERTEX_POINT('',#84807);
#24540=VERTEX_POINT('',#84860);
#24541=VERTEX_POINT('',#84861);
#24542=VERTEX_POINT('',#84863);
#24543=VERTEX_POINT('',#84870);
#24544=VERTEX_POINT('',#84871);
#24545=VERTEX_POINT('',#84884);
#24546=VERTEX_POINT('',#84897);
#24547=VERTEX_POINT('',#84898);
#24548=VERTEX_POINT('',#84922);
#24549=VERTEX_POINT('',#84923);
#24550=VERTEX_POINT('',#84946);
#24551=VERTEX_POINT('',#84947);
#24552=VERTEX_POINT('',#84971);
#24553=VERTEX_POINT('',#84972);
#24554=VERTEX_POINT('',#84996);
#24555=VERTEX_POINT('',#84997);
#24556=VERTEX_POINT('',#85020);
#24557=VERTEX_POINT('',#85021);
#24558=VERTEX_POINT('',#85045);
#24559=VERTEX_POINT('',#85046);
#24560=VERTEX_POINT('',#85070);
#24561=VERTEX_POINT('',#85071);
#24562=VERTEX_POINT('',#85094);
#24563=VERTEX_POINT('',#85095);
#24564=VERTEX_POINT('',#85119);
#24565=VERTEX_POINT('',#85120);
#24566=VERTEX_POINT('',#85144);
#24567=VERTEX_POINT('',#85145);
#24568=VERTEX_POINT('',#85168);
#24569=VERTEX_POINT('',#85169);
#24570=VERTEX_POINT('',#85193);
#24571=VERTEX_POINT('',#85194);
#24572=VERTEX_POINT('',#85218);
#24573=VERTEX_POINT('',#85219);
#24574=VERTEX_POINT('',#85242);
#24575=VERTEX_POINT('',#85349);
#24576=VERTEX_POINT('',#85351);
#24577=VERTEX_POINT('',#85900);
#24578=VERTEX_POINT('',#86017);
#24579=VERTEX_POINT('',#86020);
#24580=VERTEX_POINT('',#86580);
#24581=VERTEX_POINT('',#86586);
#24582=VERTEX_POINT('',#86589);
#24583=VERTEX_POINT('',#86590);
#24584=VERTEX_POINT('',#86592);
#24585=VERTEX_POINT('',#86594);
#24586=VERTEX_POINT('',#86598);
#24587=VERTEX_POINT('',#86602);
#24588=VERTEX_POINT('',#86608);
#24589=VERTEX_POINT('',#86609);
#24590=VERTEX_POINT('',#86611);
#24591=VERTEX_POINT('',#86613);
#24592=VERTEX_POINT('',#86617);
#24593=VERTEX_POINT('',#86621);
#24594=VERTEX_POINT('',#86627);
#24595=VERTEX_POINT('',#86628);
#24596=VERTEX_POINT('',#86630);
#24597=VERTEX_POINT('',#86632);
#24598=VERTEX_POINT('',#86636);
#24599=VERTEX_POINT('',#86640);
#24600=VERTEX_POINT('',#86646);
#24601=VERTEX_POINT('',#86647);
#24602=VERTEX_POINT('',#86649);
#24603=VERTEX_POINT('',#86651);
#24604=VERTEX_POINT('',#86655);
#24605=VERTEX_POINT('',#86659);
#24606=VERTEX_POINT('',#86665);
#24607=VERTEX_POINT('',#86666);
#24608=VERTEX_POINT('',#86668);
#24609=VERTEX_POINT('',#86670);
#24610=VERTEX_POINT('',#86674);
#24611=VERTEX_POINT('',#86678);
#24612=VERTEX_POINT('',#86684);
#24613=VERTEX_POINT('',#86685);
#24614=VERTEX_POINT('',#86687);
#24615=VERTEX_POINT('',#86689);
#24616=VERTEX_POINT('',#86693);
#24617=VERTEX_POINT('',#86697);
#24618=VERTEX_POINT('',#86703);
#24619=VERTEX_POINT('',#86704);
#24620=VERTEX_POINT('',#86706);
#24621=VERTEX_POINT('',#86708);
#24622=VERTEX_POINT('',#86712);
#24623=VERTEX_POINT('',#86716);
#24624=VERTEX_POINT('',#86722);
#24625=VERTEX_POINT('',#86723);
#24626=VERTEX_POINT('',#86725);
#24627=VERTEX_POINT('',#86727);
#24628=VERTEX_POINT('',#86731);
#24629=VERTEX_POINT('',#86735);
#24630=VERTEX_POINT('',#86741);
#24631=VERTEX_POINT('',#86742);
#24632=VERTEX_POINT('',#86744);
#24633=VERTEX_POINT('',#86746);
#24634=VERTEX_POINT('',#86750);
#24635=VERTEX_POINT('',#86754);
#24636=VERTEX_POINT('',#86760);
#24637=VERTEX_POINT('',#86761);
#24638=VERTEX_POINT('',#86763);
#24639=VERTEX_POINT('',#86765);
#24640=VERTEX_POINT('',#86769);
#24641=VERTEX_POINT('',#86773);
#24642=VERTEX_POINT('',#86779);
#24643=VERTEX_POINT('',#86780);
#24644=VERTEX_POINT('',#86782);
#24645=VERTEX_POINT('',#86784);
#24646=VERTEX_POINT('',#86788);
#24647=VERTEX_POINT('',#86792);
#24648=VERTEX_POINT('',#86798);
#24649=VERTEX_POINT('',#86799);
#24650=VERTEX_POINT('',#86801);
#24651=VERTEX_POINT('',#86803);
#24652=VERTEX_POINT('',#86807);
#24653=VERTEX_POINT('',#86811);
#24654=VERTEX_POINT('',#86817);
#24655=VERTEX_POINT('',#86818);
#24656=VERTEX_POINT('',#86820);
#24657=VERTEX_POINT('',#86822);
#24658=VERTEX_POINT('',#86826);
#24659=VERTEX_POINT('',#86830);
#24660=VERTEX_POINT('',#86836);
#24661=VERTEX_POINT('',#86837);
#24662=VERTEX_POINT('',#86839);
#24663=VERTEX_POINT('',#86841);
#24664=VERTEX_POINT('',#86845);
#24665=VERTEX_POINT('',#86849);
#24666=VERTEX_POINT('',#86855);
#24667=VERTEX_POINT('',#86856);
#24668=VERTEX_POINT('',#86858);
#24669=VERTEX_POINT('',#86860);
#24670=VERTEX_POINT('',#86864);
#24671=VERTEX_POINT('',#86868);
#24672=VERTEX_POINT('',#86874);
#24673=VERTEX_POINT('',#86875);
#24674=VERTEX_POINT('',#86877);
#24675=VERTEX_POINT('',#86879);
#24676=VERTEX_POINT('',#86883);
#24677=VERTEX_POINT('',#86887);
#24678=VERTEX_POINT('',#86893);
#24679=VERTEX_POINT('',#86894);
#24680=VERTEX_POINT('',#86896);
#24681=VERTEX_POINT('',#86898);
#24682=VERTEX_POINT('',#86902);
#24683=VERTEX_POINT('',#86906);
#24684=VERTEX_POINT('',#86912);
#24685=VERTEX_POINT('',#86913);
#24686=VERTEX_POINT('',#86915);
#24687=VERTEX_POINT('',#86917);
#24688=VERTEX_POINT('',#86921);
#24689=VERTEX_POINT('',#86923);
#24690=VERTEX_POINT('',#86927);
#24691=VERTEX_POINT('',#86931);
#24692=VERTEX_POINT('',#86935);
#24693=VERTEX_POINT('',#86936);
#24694=VERTEX_POINT('',#86938);
#24695=VERTEX_POINT('',#86940);
#24696=VERTEX_POINT('',#86944);
#24697=VERTEX_POINT('',#86948);
#24698=VERTEX_POINT('',#86954);
#24699=VERTEX_POINT('',#86955);
#24700=VERTEX_POINT('',#86957);
#24701=VERTEX_POINT('',#86959);
#24702=VERTEX_POINT('',#86963);
#24703=VERTEX_POINT('',#86967);
#24704=VERTEX_POINT('',#86973);
#24705=VERTEX_POINT('',#86974);
#24706=VERTEX_POINT('',#86976);
#24707=VERTEX_POINT('',#86978);
#24708=VERTEX_POINT('',#86982);
#24709=VERTEX_POINT('',#86986);
#24710=VERTEX_POINT('',#86992);
#24711=VERTEX_POINT('',#86993);
#24712=VERTEX_POINT('',#86995);
#24713=VERTEX_POINT('',#86997);
#24714=VERTEX_POINT('',#87001);
#24715=VERTEX_POINT('',#87005);
#24716=VERTEX_POINT('',#87011);
#24717=VERTEX_POINT('',#87012);
#24718=VERTEX_POINT('',#87014);
#24719=VERTEX_POINT('',#87016);
#24720=VERTEX_POINT('',#87020);
#24721=VERTEX_POINT('',#87024);
#24722=VERTEX_POINT('',#87030);
#24723=VERTEX_POINT('',#87031);
#24724=VERTEX_POINT('',#87033);
#24725=VERTEX_POINT('',#87035);
#24726=VERTEX_POINT('',#87039);
#24727=VERTEX_POINT('',#87043);
#24728=VERTEX_POINT('',#87049);
#24729=VERTEX_POINT('',#87050);
#24730=VERTEX_POINT('',#87052);
#24731=VERTEX_POINT('',#87054);
#24732=VERTEX_POINT('',#87058);
#24733=VERTEX_POINT('',#87062);
#24734=VERTEX_POINT('',#87068);
#24735=VERTEX_POINT('',#87069);
#24736=VERTEX_POINT('',#87071);
#24737=VERTEX_POINT('',#87073);
#24738=VERTEX_POINT('',#87077);
#24739=VERTEX_POINT('',#87081);
#24740=VERTEX_POINT('',#87087);
#24741=VERTEX_POINT('',#87088);
#24742=VERTEX_POINT('',#87090);
#24743=VERTEX_POINT('',#87092);
#24744=VERTEX_POINT('',#87096);
#24745=VERTEX_POINT('',#87100);
#24746=VERTEX_POINT('',#87106);
#24747=VERTEX_POINT('',#87107);
#24748=VERTEX_POINT('',#87109);
#24749=VERTEX_POINT('',#87111);
#24750=VERTEX_POINT('',#87115);
#24751=VERTEX_POINT('',#87119);
#24752=VERTEX_POINT('',#87125);
#24753=VERTEX_POINT('',#87126);
#24754=VERTEX_POINT('',#87128);
#24755=VERTEX_POINT('',#87130);
#24756=VERTEX_POINT('',#87134);
#24757=VERTEX_POINT('',#87138);
#24758=VERTEX_POINT('',#87144);
#24759=VERTEX_POINT('',#87145);
#24760=VERTEX_POINT('',#87147);
#24761=VERTEX_POINT('',#87149);
#24762=VERTEX_POINT('',#87153);
#24763=VERTEX_POINT('',#87157);
#24764=VERTEX_POINT('',#87163);
#24765=VERTEX_POINT('',#87164);
#24766=VERTEX_POINT('',#87166);
#24767=VERTEX_POINT('',#87168);
#24768=VERTEX_POINT('',#87172);
#24769=VERTEX_POINT('',#87176);
#24770=VERTEX_POINT('',#87182);
#24771=VERTEX_POINT('',#87183);
#24772=VERTEX_POINT('',#87185);
#24773=VERTEX_POINT('',#87187);
#24774=VERTEX_POINT('',#87191);
#24775=VERTEX_POINT('',#87195);
#24776=VERTEX_POINT('',#87201);
#24777=VERTEX_POINT('',#87202);
#24778=VERTEX_POINT('',#87204);
#24779=VERTEX_POINT('',#87206);
#24780=VERTEX_POINT('',#87210);
#24781=VERTEX_POINT('',#87214);
#24782=VERTEX_POINT('',#87220);
#24783=VERTEX_POINT('',#87221);
#24784=VERTEX_POINT('',#87223);
#24785=VERTEX_POINT('',#87225);
#24786=VERTEX_POINT('',#87229);
#24787=VERTEX_POINT('',#87233);
#24788=VERTEX_POINT('',#87239);
#24789=VERTEX_POINT('',#87240);
#24790=VERTEX_POINT('',#87242);
#24791=VERTEX_POINT('',#87244);
#24792=VERTEX_POINT('',#87248);
#24793=VERTEX_POINT('',#87252);
#24794=VERTEX_POINT('',#87258);
#24795=VERTEX_POINT('',#87259);
#24796=VERTEX_POINT('',#87261);
#24797=VERTEX_POINT('',#87265);
#24798=VERTEX_POINT('',#87267);
#24799=VERTEX_POINT('',#87271);
#24800=VERTEX_POINT('',#87277);
#24801=VERTEX_POINT('',#87278);
#24802=VERTEX_POINT('',#87282);
#24803=VERTEX_POINT('',#87283);
#24804=VERTEX_POINT('',#87285);
#24805=VERTEX_POINT('',#87287);
#24806=VERTEX_POINT('',#87291);
#24807=VERTEX_POINT('',#87293);
#24808=VERTEX_POINT('',#87297);
#24809=VERTEX_POINT('',#87299);
#24810=VERTEX_POINT('',#87303);
#24811=VERTEX_POINT('',#87305);
#24812=VERTEX_POINT('',#87309);
#24813=VERTEX_POINT('',#87311);
#24814=VERTEX_POINT('',#87319);
#24815=VERTEX_POINT('',#87362);
#31613=EDGE_CURVE('',#24506,#24507,#5979,.T.);
#31614=EDGE_CURVE('',#24506,#24508,#479,.T.);
#31615=EDGE_CURVE('',#24508,#24509,#20009,.T.);
#31616=EDGE_CURVE('',#24509,#24507,#480,.T.);
#31617=EDGE_CURVE('',#24510,#24511,#5980,.T.);
#31618=EDGE_CURVE('',#24510,#24506,#481,.T.);
#31619=EDGE_CURVE('',#24507,#24511,#482,.T.);
#31620=EDGE_CURVE('',#24512,#24513,#5981,.T.);
#31621=EDGE_CURVE('',#24512,#24510,#483,.T.);
#31622=EDGE_CURVE('',#24511,#24513,#484,.T.);
#31623=EDGE_CURVE('',#24514,#24515,#5982,.T.);
#31624=EDGE_CURVE('',#24514,#24512,#485,.T.);
#31625=EDGE_CURVE('',#24513,#24515,#486,.T.);
#31626=EDGE_CURVE('',#24516,#24517,#5983,.T.);
#31627=EDGE_CURVE('',#24516,#24514,#487,.T.);
#31628=EDGE_CURVE('',#24515,#24517,#488,.T.);
#31629=EDGE_CURVE('',#24518,#24519,#5984,.T.);
#31630=EDGE_CURVE('',#24518,#24516,#489,.T.);
#31631=EDGE_CURVE('',#24517,#24519,#490,.T.);
#31632=EDGE_CURVE('',#24520,#24521,#5985,.T.);
#31633=EDGE_CURVE('',#24520,#24518,#491,.T.);
#31634=EDGE_CURVE('',#24519,#24521,#492,.T.);
#31635=EDGE_CURVE('',#24522,#24523,#5986,.T.);
#31636=EDGE_CURVE('',#24522,#24520,#493,.T.);
#31637=EDGE_CURVE('',#24521,#24523,#494,.T.);
#31638=EDGE_CURVE('',#24524,#24525,#5987,.T.);
#31639=EDGE_CURVE('',#24524,#24522,#495,.T.);
#31640=EDGE_CURVE('',#24523,#24525,#496,.T.);
#31641=EDGE_CURVE('',#24526,#24527,#5988,.T.);
#31642=EDGE_CURVE('',#24526,#24524,#497,.T.);
#31643=EDGE_CURVE('',#24525,#24527,#498,.T.);
#31644=EDGE_CURVE('',#24528,#24529,#5989,.T.);
#31645=EDGE_CURVE('',#24528,#24526,#499,.T.);
#31646=EDGE_CURVE('',#24527,#24529,#500,.T.);
#31647=EDGE_CURVE('',#24530,#24531,#5990,.T.);
#31648=EDGE_CURVE('',#24530,#24528,#501,.T.);
#31649=EDGE_CURVE('',#24529,#24531,#502,.T.);
#31650=EDGE_CURVE('',#24532,#24533,#5991,.T.);
#31651=EDGE_CURVE('',#24532,#24530,#503,.T.);
#31652=EDGE_CURVE('',#24531,#24533,#504,.T.);
#31653=EDGE_CURVE('',#24534,#24535,#5992,.T.);
#31654=EDGE_CURVE('',#24534,#24532,#505,.T.);
#31655=EDGE_CURVE('',#24533,#24535,#506,.T.);
#31656=EDGE_CURVE('',#24536,#24537,#5993,.T.);
#31657=EDGE_CURVE('',#24536,#24534,#507,.T.);
#31658=EDGE_CURVE('',#24535,#24537,#508,.T.);
#31659=EDGE_CURVE('',#24538,#24539,#5994,.T.);
#31660=EDGE_CURVE('',#24538,#24536,#509,.T.);
#31661=EDGE_CURVE('',#24537,#24539,#510,.T.);
#31662=EDGE_CURVE('',#24540,#24541,#5995,.T.);
#31663=EDGE_CURVE('',#24540,#24542,#511,.T.);
#31664=EDGE_CURVE('',#24541,#24542,#20010,.T.);
#31665=EDGE_CURVE('',#24543,#24544,#5996,.T.);
#31666=EDGE_CURVE('',#24543,#24540,#512,.T.);
#31667=EDGE_CURVE('',#24545,#24541,#20011,.T.);
#31668=EDGE_CURVE('',#24544,#24545,#513,.T.);
#31669=EDGE_CURVE('',#24546,#24547,#5997,.T.);
#31670=EDGE_CURVE('',#24546,#24543,#514,.T.);
#31671=EDGE_CURVE('',#24547,#24544,#515,.T.);
#31672=EDGE_CURVE('',#24548,#24549,#5998,.T.);
#31673=EDGE_CURVE('',#24548,#24546,#516,.T.);
#31674=EDGE_CURVE('',#24549,#24547,#517,.T.);
#31675=EDGE_CURVE('',#24550,#24551,#5999,.T.);
#31676=EDGE_CURVE('',#24550,#24548,#518,.T.);
#31677=EDGE_CURVE('',#24551,#24549,#519,.T.);
#31678=EDGE_CURVE('',#24552,#24553,#6000,.T.);
#31679=EDGE_CURVE('',#24552,#24550,#520,.T.);
#31680=EDGE_CURVE('',#24553,#24551,#521,.T.);
#31681=EDGE_CURVE('',#24554,#24555,#6001,.T.);
#31682=EDGE_CURVE('',#24554,#24552,#522,.T.);
#31683=EDGE_CURVE('',#24555,#24553,#523,.T.);
#31684=EDGE_CURVE('',#24556,#24557,#6002,.T.);
#31685=EDGE_CURVE('',#24556,#24554,#524,.T.);
#31686=EDGE_CURVE('',#24557,#24555,#525,.T.);
#31687=EDGE_CURVE('',#24558,#24559,#6003,.T.);
#31688=EDGE_CURVE('',#24558,#24556,#526,.T.);
#31689=EDGE_CURVE('',#24559,#24557,#527,.T.);
#31690=EDGE_CURVE('',#24560,#24561,#6004,.T.);
#31691=EDGE_CURVE('',#24560,#24558,#528,.T.);
#31692=EDGE_CURVE('',#24561,#24559,#529,.T.);
#31693=EDGE_CURVE('',#24562,#24563,#6005,.T.);
#31694=EDGE_CURVE('',#24562,#24560,#530,.T.);
#31695=EDGE_CURVE('',#24563,#24561,#531,.T.);
#31696=EDGE_CURVE('',#24564,#24565,#6006,.T.);
#31697=EDGE_CURVE('',#24564,#24562,#532,.T.);
#31698=EDGE_CURVE('',#24565,#24563,#533,.T.);
#31699=EDGE_CURVE('',#24566,#24567,#6007,.T.);
#31700=EDGE_CURVE('',#24566,#24564,#534,.T.);
#31701=EDGE_CURVE('',#24567,#24565,#535,.T.);
#31702=EDGE_CURVE('',#24568,#24569,#6008,.T.);
#31703=EDGE_CURVE('',#24568,#24566,#536,.T.);
#31704=EDGE_CURVE('',#24569,#24567,#537,.T.);
#31705=EDGE_CURVE('',#24570,#24571,#6009,.T.);
#31706=EDGE_CURVE('',#24570,#24568,#538,.T.);
#31707=EDGE_CURVE('',#24571,#24569,#539,.T.);
#31708=EDGE_CURVE('',#24572,#24573,#6010,.T.);
#31709=EDGE_CURVE('',#24572,#24570,#540,.T.);
#31710=EDGE_CURVE('',#24573,#24571,#541,.T.);
#31711=EDGE_CURVE('',#24542,#24574,#542,.T.);
#31712=EDGE_CURVE('',#24575,#24574,#20012,.T.);
#31713=EDGE_CURVE('',#24576,#24575,#20013,.T.);
#31714=EDGE_CURVE('',#24576,#24545,#543,.T.);
#31715=EDGE_CURVE('',#24539,#24576,#544,.T.);
#31716=EDGE_CURVE('',#24577,#24509,#545,.T.);
#31717=EDGE_CURVE('',#24577,#24573,#546,.T.);
#31718=EDGE_CURVE('',#24509,#24578,#20014,.T.);
#31719=EDGE_CURVE('',#24578,#24508,#20015,.T.);
#31720=EDGE_CURVE('',#24508,#24579,#547,.T.);
#31721=EDGE_CURVE('',#24579,#24577,#20016,.T.);
#31722=EDGE_CURVE('',#24579,#24572,#548,.T.);
#31723=EDGE_CURVE('',#24574,#24538,#549,.T.);
#31724=EDGE_CURVE('',#24575,#24580,#20017,.T.);
#31725=EDGE_CURVE('',#24580,#24580,#20018,.T.);
#31726=EDGE_CURVE('',#24574,#24576,#20019,.T.);
#31727=EDGE_CURVE('',#24581,#24581,#20020,.T.);
#31728=EDGE_CURVE('',#24582,#24583,#6011,.T.);
#31729=EDGE_CURVE('',#24582,#24584,#6012,.T.);
#31730=EDGE_CURVE('',#24584,#24585,#6013,.T.);
#31731=EDGE_CURVE('',#24585,#24583,#6014,.T.);
#31732=EDGE_CURVE('',#24583,#24586,#20021,.T.);
#31733=EDGE_CURVE('',#24586,#24585,#6015,.T.);
#31734=EDGE_CURVE('',#24586,#24587,#6016,.T.);
#31735=EDGE_CURVE('',#24584,#24587,#6017,.T.);
#31736=EDGE_CURVE('',#24587,#24582,#20022,.T.);
#31737=EDGE_CURVE('',#24588,#24589,#6018,.T.);
#31738=EDGE_CURVE('',#24588,#24590,#6019,.T.);
#31739=EDGE_CURVE('',#24590,#24591,#6020,.T.);
#31740=EDGE_CURVE('',#24591,#24589,#6021,.T.);
#31741=EDGE_CURVE('',#24589,#24592,#20023,.T.);
#31742=EDGE_CURVE('',#24592,#24591,#6022,.T.);
#31743=EDGE_CURVE('',#24592,#24593,#6023,.T.);
#31744=EDGE_CURVE('',#24590,#24593,#6024,.T.);
#31745=EDGE_CURVE('',#24593,#24588,#20024,.T.);
#31746=EDGE_CURVE('',#24594,#24595,#6025,.T.);
#31747=EDGE_CURVE('',#24594,#24596,#6026,.T.);
#31748=EDGE_CURVE('',#24596,#24597,#6027,.T.);
#31749=EDGE_CURVE('',#24597,#24595,#6028,.T.);
#31750=EDGE_CURVE('',#24595,#24598,#20025,.T.);
#31751=EDGE_CURVE('',#24598,#24597,#6029,.T.);
#31752=EDGE_CURVE('',#24598,#24599,#6030,.T.);
#31753=EDGE_CURVE('',#24596,#24599,#6031,.T.);
#31754=EDGE_CURVE('',#24599,#24594,#20026,.T.);
#31755=EDGE_CURVE('',#24600,#24601,#6032,.T.);
#31756=EDGE_CURVE('',#24600,#24602,#6033,.T.);
#31757=EDGE_CURVE('',#24602,#24603,#6034,.T.);
#31758=EDGE_CURVE('',#24603,#24601,#6035,.T.);
#31759=EDGE_CURVE('',#24601,#24604,#20027,.T.);
#31760=EDGE_CURVE('',#24604,#24603,#6036,.T.);
#31761=EDGE_CURVE('',#24604,#24605,#6037,.T.);
#31762=EDGE_CURVE('',#24602,#24605,#6038,.T.);
#31763=EDGE_CURVE('',#24605,#24600,#20028,.T.);
#31764=EDGE_CURVE('',#24606,#24607,#6039,.T.);
#31765=EDGE_CURVE('',#24606,#24608,#6040,.T.);
#31766=EDGE_CURVE('',#24608,#24609,#6041,.T.);
#31767=EDGE_CURVE('',#24609,#24607,#6042,.T.);
#31768=EDGE_CURVE('',#24607,#24610,#20029,.T.);
#31769=EDGE_CURVE('',#24610,#24609,#6043,.T.);
#31770=EDGE_CURVE('',#24610,#24611,#6044,.T.);
#31771=EDGE_CURVE('',#24608,#24611,#6045,.T.);
#31772=EDGE_CURVE('',#24611,#24606,#20030,.T.);
#31773=EDGE_CURVE('',#24612,#24613,#6046,.T.);
#31774=EDGE_CURVE('',#24612,#24614,#6047,.T.);
#31775=EDGE_CURVE('',#24614,#24615,#6048,.T.);
#31776=EDGE_CURVE('',#24615,#24613,#6049,.T.);
#31777=EDGE_CURVE('',#24613,#24616,#20031,.T.);
#31778=EDGE_CURVE('',#24616,#24615,#6050,.T.);
#31779=EDGE_CURVE('',#24616,#24617,#6051,.T.);
#31780=EDGE_CURVE('',#24614,#24617,#6052,.T.);
#31781=EDGE_CURVE('',#24617,#24612,#20032,.T.);
#31782=EDGE_CURVE('',#24618,#24619,#6053,.T.);
#31783=EDGE_CURVE('',#24618,#24620,#6054,.T.);
#31784=EDGE_CURVE('',#24620,#24621,#6055,.T.);
#31785=EDGE_CURVE('',#24621,#24619,#6056,.T.);
#31786=EDGE_CURVE('',#24619,#24622,#20033,.T.);
#31787=EDGE_CURVE('',#24622,#24621,#6057,.T.);
#31788=EDGE_CURVE('',#24622,#24623,#6058,.T.);
#31789=EDGE_CURVE('',#24620,#24623,#6059,.T.);
#31790=EDGE_CURVE('',#24623,#24618,#20034,.T.);
#31791=EDGE_CURVE('',#24624,#24625,#6060,.T.);
#31792=EDGE_CURVE('',#24624,#24626,#6061,.T.);
#31793=EDGE_CURVE('',#24626,#24627,#6062,.T.);
#31794=EDGE_CURVE('',#24627,#24625,#6063,.T.);
#31795=EDGE_CURVE('',#24625,#24628,#20035,.T.);
#31796=EDGE_CURVE('',#24628,#24627,#6064,.T.);
#31797=EDGE_CURVE('',#24628,#24629,#6065,.T.);
#31798=EDGE_CURVE('',#24626,#24629,#6066,.T.);
#31799=EDGE_CURVE('',#24629,#24624,#20036,.T.);
#31800=EDGE_CURVE('',#24630,#24631,#6067,.T.);
#31801=EDGE_CURVE('',#24630,#24632,#6068,.T.);
#31802=EDGE_CURVE('',#24632,#24633,#6069,.T.);
#31803=EDGE_CURVE('',#24633,#24631,#6070,.T.);
#31804=EDGE_CURVE('',#24631,#24634,#20037,.T.);
#31805=EDGE_CURVE('',#24634,#24633,#6071,.T.);
#31806=EDGE_CURVE('',#24634,#24635,#6072,.T.);
#31807=EDGE_CURVE('',#24632,#24635,#6073,.T.);
#31808=EDGE_CURVE('',#24635,#24630,#20038,.T.);
#31809=EDGE_CURVE('',#24636,#24637,#6074,.T.);
#31810=EDGE_CURVE('',#24636,#24638,#6075,.T.);
#31811=EDGE_CURVE('',#24638,#24639,#6076,.T.);
#31812=EDGE_CURVE('',#24639,#24637,#6077,.T.);
#31813=EDGE_CURVE('',#24637,#24640,#20039,.T.);
#31814=EDGE_CURVE('',#24640,#24639,#6078,.T.);
#31815=EDGE_CURVE('',#24640,#24641,#6079,.T.);
#31816=EDGE_CURVE('',#24638,#24641,#6080,.T.);
#31817=EDGE_CURVE('',#24641,#24636,#20040,.T.);
#31818=EDGE_CURVE('',#24642,#24643,#6081,.T.);
#31819=EDGE_CURVE('',#24642,#24644,#6082,.T.);
#31820=EDGE_CURVE('',#24644,#24645,#6083,.T.);
#31821=EDGE_CURVE('',#24645,#24643,#6084,.T.);
#31822=EDGE_CURVE('',#24643,#24646,#20041,.T.);
#31823=EDGE_CURVE('',#24646,#24645,#6085,.T.);
#31824=EDGE_CURVE('',#24646,#24647,#6086,.T.);
#31825=EDGE_CURVE('',#24644,#24647,#6087,.T.);
#31826=EDGE_CURVE('',#24647,#24642,#20042,.T.);
#31827=EDGE_CURVE('',#24648,#24649,#6088,.T.);
#31828=EDGE_CURVE('',#24648,#24650,#6089,.T.);
#31829=EDGE_CURVE('',#24650,#24651,#6090,.T.);
#31830=EDGE_CURVE('',#24651,#24649,#6091,.T.);
#31831=EDGE_CURVE('',#24649,#24652,#20043,.T.);
#31832=EDGE_CURVE('',#24652,#24651,#6092,.T.);
#31833=EDGE_CURVE('',#24652,#24653,#6093,.T.);
#31834=EDGE_CURVE('',#24650,#24653,#6094,.T.);
#31835=EDGE_CURVE('',#24653,#24648,#20044,.T.);
#31836=EDGE_CURVE('',#24654,#24655,#6095,.T.);
#31837=EDGE_CURVE('',#24654,#24656,#6096,.T.);
#31838=EDGE_CURVE('',#24656,#24657,#6097,.T.);
#31839=EDGE_CURVE('',#24657,#24655,#6098,.T.);
#31840=EDGE_CURVE('',#24655,#24658,#20045,.T.);
#31841=EDGE_CURVE('',#24658,#24657,#6099,.T.);
#31842=EDGE_CURVE('',#24658,#24659,#6100,.T.);
#31843=EDGE_CURVE('',#24656,#24659,#6101,.T.);
#31844=EDGE_CURVE('',#24659,#24654,#20046,.T.);
#31845=EDGE_CURVE('',#24660,#24661,#6102,.T.);
#31846=EDGE_CURVE('',#24660,#24662,#6103,.T.);
#31847=EDGE_CURVE('',#24662,#24663,#6104,.T.);
#31848=EDGE_CURVE('',#24663,#24661,#6105,.T.);
#31849=EDGE_CURVE('',#24661,#24664,#20047,.T.);
#31850=EDGE_CURVE('',#24664,#24663,#6106,.T.);
#31851=EDGE_CURVE('',#24664,#24665,#6107,.T.);
#31852=EDGE_CURVE('',#24662,#24665,#6108,.T.);
#31853=EDGE_CURVE('',#24665,#24660,#20048,.T.);
#31854=EDGE_CURVE('',#24666,#24667,#6109,.T.);
#31855=EDGE_CURVE('',#24666,#24668,#6110,.T.);
#31856=EDGE_CURVE('',#24668,#24669,#6111,.T.);
#31857=EDGE_CURVE('',#24669,#24667,#6112,.T.);
#31858=EDGE_CURVE('',#24667,#24670,#20049,.T.);
#31859=EDGE_CURVE('',#24670,#24669,#6113,.T.);
#31860=EDGE_CURVE('',#24670,#24671,#6114,.T.);
#31861=EDGE_CURVE('',#24668,#24671,#6115,.T.);
#31862=EDGE_CURVE('',#24671,#24666,#20050,.T.);
#31863=EDGE_CURVE('',#24672,#24673,#6116,.T.);
#31864=EDGE_CURVE('',#24672,#24674,#6117,.T.);
#31865=EDGE_CURVE('',#24674,#24675,#6118,.T.);
#31866=EDGE_CURVE('',#24675,#24673,#6119,.T.);
#31867=EDGE_CURVE('',#24673,#24676,#20051,.T.);
#31868=EDGE_CURVE('',#24676,#24675,#6120,.T.);
#31869=EDGE_CURVE('',#24676,#24677,#6121,.T.);
#31870=EDGE_CURVE('',#24674,#24677,#6122,.T.);
#31871=EDGE_CURVE('',#24677,#24672,#20052,.T.);
#31872=EDGE_CURVE('',#24678,#24679,#6123,.T.);
#31873=EDGE_CURVE('',#24678,#24680,#6124,.T.);
#31874=EDGE_CURVE('',#24680,#24681,#6125,.T.);
#31875=EDGE_CURVE('',#24681,#24679,#6126,.T.);
#31876=EDGE_CURVE('',#24679,#24682,#20053,.T.);
#31877=EDGE_CURVE('',#24682,#24681,#6127,.T.);
#31878=EDGE_CURVE('',#24682,#24683,#6128,.T.);
#31879=EDGE_CURVE('',#24680,#24683,#6129,.T.);
#31880=EDGE_CURVE('',#24683,#24678,#20054,.T.);
#31881=EDGE_CURVE('',#24684,#24685,#6130,.T.);
#31882=EDGE_CURVE('',#24684,#24686,#6131,.T.);
#31883=EDGE_CURVE('',#24686,#24687,#6132,.T.);
#31884=EDGE_CURVE('',#24687,#24685,#6133,.T.);
#31885=EDGE_CURVE('',#24685,#24688,#20055,.T.);
#31886=EDGE_CURVE('',#24689,#24687,#6134,.T.);
#31887=EDGE_CURVE('',#24688,#24689,#20056,.T.);
#31888=EDGE_CURVE('',#24689,#24690,#6135,.T.);
#31889=EDGE_CURVE('',#24686,#24690,#6136,.T.);
#31890=EDGE_CURVE('',#24690,#24691,#20057,.T.);
#31891=EDGE_CURVE('',#24691,#24684,#20058,.T.);
#31892=EDGE_CURVE('',#24692,#24693,#6137,.T.);
#31893=EDGE_CURVE('',#24692,#24694,#6138,.T.);
#31894=EDGE_CURVE('',#24694,#24695,#6139,.T.);
#31895=EDGE_CURVE('',#24695,#24693,#6140,.T.);
#31896=EDGE_CURVE('',#24693,#24696,#20059,.T.);
#31897=EDGE_CURVE('',#24696,#24695,#6141,.T.);
#31898=EDGE_CURVE('',#24696,#24697,#6142,.T.);
#31899=EDGE_CURVE('',#24694,#24697,#6143,.T.);
#31900=EDGE_CURVE('',#24697,#24692,#20060,.T.);
#31901=EDGE_CURVE('',#24698,#24699,#6144,.T.);
#31902=EDGE_CURVE('',#24698,#24700,#6145,.T.);
#31903=EDGE_CURVE('',#24700,#24701,#6146,.T.);
#31904=EDGE_CURVE('',#24701,#24699,#6147,.T.);
#31905=EDGE_CURVE('',#24699,#24702,#20061,.T.);
#31906=EDGE_CURVE('',#24702,#24701,#6148,.T.);
#31907=EDGE_CURVE('',#24702,#24703,#6149,.T.);
#31908=EDGE_CURVE('',#24700,#24703,#6150,.T.);
#31909=EDGE_CURVE('',#24703,#24698,#20062,.T.);
#31910=EDGE_CURVE('',#24704,#24705,#6151,.T.);
#31911=EDGE_CURVE('',#24704,#24706,#6152,.T.);
#31912=EDGE_CURVE('',#24706,#24707,#6153,.T.);
#31913=EDGE_CURVE('',#24707,#24705,#6154,.T.);
#31914=EDGE_CURVE('',#24705,#24708,#20063,.T.);
#31915=EDGE_CURVE('',#24708,#24707,#6155,.T.);
#31916=EDGE_CURVE('',#24708,#24709,#6156,.T.);
#31917=EDGE_CURVE('',#24706,#24709,#6157,.T.);
#31918=EDGE_CURVE('',#24709,#24704,#20064,.T.);
#31919=EDGE_CURVE('',#24710,#24711,#6158,.T.);
#31920=EDGE_CURVE('',#24710,#24712,#6159,.T.);
#31921=EDGE_CURVE('',#24712,#24713,#6160,.T.);
#31922=EDGE_CURVE('',#24713,#24711,#6161,.T.);
#31923=EDGE_CURVE('',#24711,#24714,#20065,.T.);
#31924=EDGE_CURVE('',#24714,#24713,#6162,.T.);
#31925=EDGE_CURVE('',#24714,#24715,#6163,.T.);
#31926=EDGE_CURVE('',#24712,#24715,#6164,.T.);
#31927=EDGE_CURVE('',#24715,#24710,#20066,.T.);
#31928=EDGE_CURVE('',#24716,#24717,#6165,.T.);
#31929=EDGE_CURVE('',#24716,#24718,#6166,.T.);
#31930=EDGE_CURVE('',#24718,#24719,#6167,.T.);
#31931=EDGE_CURVE('',#24719,#24717,#6168,.T.);
#31932=EDGE_CURVE('',#24717,#24720,#20067,.T.);
#31933=EDGE_CURVE('',#24720,#24719,#6169,.T.);
#31934=EDGE_CURVE('',#24720,#24721,#6170,.T.);
#31935=EDGE_CURVE('',#24718,#24721,#6171,.T.);
#31936=EDGE_CURVE('',#24721,#24716,#20068,.T.);
#31937=EDGE_CURVE('',#24722,#24723,#6172,.T.);
#31938=EDGE_CURVE('',#24722,#24724,#6173,.T.);
#31939=EDGE_CURVE('',#24724,#24725,#6174,.T.);
#31940=EDGE_CURVE('',#24725,#24723,#6175,.T.);
#31941=EDGE_CURVE('',#24723,#24726,#20069,.T.);
#31942=EDGE_CURVE('',#24726,#24725,#6176,.T.);
#31943=EDGE_CURVE('',#24726,#24727,#6177,.T.);
#31944=EDGE_CURVE('',#24724,#24727,#6178,.T.);
#31945=EDGE_CURVE('',#24727,#24722,#20070,.T.);
#31946=EDGE_CURVE('',#24728,#24729,#6179,.T.);
#31947=EDGE_CURVE('',#24728,#24730,#6180,.T.);
#31948=EDGE_CURVE('',#24730,#24731,#6181,.T.);
#31949=EDGE_CURVE('',#24731,#24729,#6182,.T.);
#31950=EDGE_CURVE('',#24729,#24732,#20071,.T.);
#31951=EDGE_CURVE('',#24732,#24731,#6183,.T.);
#31952=EDGE_CURVE('',#24732,#24733,#6184,.T.);
#31953=EDGE_CURVE('',#24730,#24733,#6185,.T.);
#31954=EDGE_CURVE('',#24733,#24728,#20072,.T.);
#31955=EDGE_CURVE('',#24734,#24735,#6186,.T.);
#31956=EDGE_CURVE('',#24734,#24736,#6187,.T.);
#31957=EDGE_CURVE('',#24736,#24737,#6188,.T.);
#31958=EDGE_CURVE('',#24737,#24735,#6189,.T.);
#31959=EDGE_CURVE('',#24735,#24738,#20073,.T.);
#31960=EDGE_CURVE('',#24738,#24737,#6190,.T.);
#31961=EDGE_CURVE('',#24738,#24739,#6191,.T.);
#31962=EDGE_CURVE('',#24736,#24739,#6192,.T.);
#31963=EDGE_CURVE('',#24739,#24734,#20074,.T.);
#31964=EDGE_CURVE('',#24740,#24741,#6193,.T.);
#31965=EDGE_CURVE('',#24740,#24742,#6194,.T.);
#31966=EDGE_CURVE('',#24742,#24743,#6195,.T.);
#31967=EDGE_CURVE('',#24743,#24741,#6196,.T.);
#31968=EDGE_CURVE('',#24741,#24744,#20075,.T.);
#31969=EDGE_CURVE('',#24744,#24743,#6197,.T.);
#31970=EDGE_CURVE('',#24744,#24745,#6198,.T.);
#31971=EDGE_CURVE('',#24742,#24745,#6199,.T.);
#31972=EDGE_CURVE('',#24745,#24740,#20076,.T.);
#31973=EDGE_CURVE('',#24746,#24747,#6200,.T.);
#31974=EDGE_CURVE('',#24746,#24748,#6201,.T.);
#31975=EDGE_CURVE('',#24748,#24749,#6202,.T.);
#31976=EDGE_CURVE('',#24749,#24747,#6203,.T.);
#31977=EDGE_CURVE('',#24747,#24750,#20077,.T.);
#31978=EDGE_CURVE('',#24750,#24749,#6204,.T.);
#31979=EDGE_CURVE('',#24750,#24751,#6205,.T.);
#31980=EDGE_CURVE('',#24748,#24751,#6206,.T.);
#31981=EDGE_CURVE('',#24751,#24746,#20078,.T.);
#31982=EDGE_CURVE('',#24752,#24753,#6207,.T.);
#31983=EDGE_CURVE('',#24752,#24754,#6208,.T.);
#31984=EDGE_CURVE('',#24754,#24755,#6209,.T.);
#31985=EDGE_CURVE('',#24755,#24753,#6210,.T.);
#31986=EDGE_CURVE('',#24753,#24756,#20079,.T.);
#31987=EDGE_CURVE('',#24756,#24755,#6211,.T.);
#31988=EDGE_CURVE('',#24756,#24757,#6212,.T.);
#31989=EDGE_CURVE('',#24754,#24757,#6213,.T.);
#31990=EDGE_CURVE('',#24757,#24752,#20080,.T.);
#31991=EDGE_CURVE('',#24758,#24759,#6214,.T.);
#31992=EDGE_CURVE('',#24758,#24760,#6215,.T.);
#31993=EDGE_CURVE('',#24760,#24761,#6216,.T.);
#31994=EDGE_CURVE('',#24761,#24759,#6217,.T.);
#31995=EDGE_CURVE('',#24759,#24762,#20081,.T.);
#31996=EDGE_CURVE('',#24762,#24761,#6218,.T.);
#31997=EDGE_CURVE('',#24762,#24763,#6219,.T.);
#31998=EDGE_CURVE('',#24760,#24763,#6220,.T.);
#31999=EDGE_CURVE('',#24763,#24758,#20082,.T.);
#32000=EDGE_CURVE('',#24764,#24765,#6221,.T.);
#32001=EDGE_CURVE('',#24764,#24766,#6222,.T.);
#32002=EDGE_CURVE('',#24766,#24767,#6223,.T.);
#32003=EDGE_CURVE('',#24767,#24765,#6224,.T.);
#32004=EDGE_CURVE('',#24765,#24768,#20083,.T.);
#32005=EDGE_CURVE('',#24768,#24767,#6225,.T.);
#32006=EDGE_CURVE('',#24768,#24769,#6226,.T.);
#32007=EDGE_CURVE('',#24766,#24769,#6227,.T.);
#32008=EDGE_CURVE('',#24769,#24764,#20084,.T.);
#32009=EDGE_CURVE('',#24770,#24771,#6228,.T.);
#32010=EDGE_CURVE('',#24770,#24772,#6229,.T.);
#32011=EDGE_CURVE('',#24772,#24773,#6230,.T.);
#32012=EDGE_CURVE('',#24773,#24771,#6231,.T.);
#32013=EDGE_CURVE('',#24771,#24774,#20085,.T.);
#32014=EDGE_CURVE('',#24774,#24773,#6232,.T.);
#32015=EDGE_CURVE('',#24774,#24775,#6233,.T.);
#32016=EDGE_CURVE('',#24772,#24775,#6234,.T.);
#32017=EDGE_CURVE('',#24775,#24770,#20086,.T.);
#32018=EDGE_CURVE('',#24776,#24777,#6235,.T.);
#32019=EDGE_CURVE('',#24776,#24778,#6236,.T.);
#32020=EDGE_CURVE('',#24778,#24779,#6237,.T.);
#32021=EDGE_CURVE('',#24779,#24777,#6238,.T.);
#32022=EDGE_CURVE('',#24777,#24780,#20087,.T.);
#32023=EDGE_CURVE('',#24780,#24779,#6239,.T.);
#32024=EDGE_CURVE('',#24780,#24781,#6240,.T.);
#32025=EDGE_CURVE('',#24778,#24781,#6241,.T.);
#32026=EDGE_CURVE('',#24781,#24776,#20088,.T.);
#32027=EDGE_CURVE('',#24782,#24783,#6242,.T.);
#32028=EDGE_CURVE('',#24782,#24784,#6243,.T.);
#32029=EDGE_CURVE('',#24784,#24785,#6244,.T.);
#32030=EDGE_CURVE('',#24785,#24783,#6245,.T.);
#32031=EDGE_CURVE('',#24783,#24786,#20089,.T.);
#32032=EDGE_CURVE('',#24786,#24785,#6246,.T.);
#32033=EDGE_CURVE('',#24786,#24787,#6247,.T.);
#32034=EDGE_CURVE('',#24784,#24787,#6248,.T.);
#32035=EDGE_CURVE('',#24787,#24782,#20090,.T.);
#32036=EDGE_CURVE('',#24788,#24789,#6249,.T.);
#32037=EDGE_CURVE('',#24788,#24790,#6250,.T.);
#32038=EDGE_CURVE('',#24790,#24791,#6251,.T.);
#32039=EDGE_CURVE('',#24791,#24789,#6252,.T.);
#32040=EDGE_CURVE('',#24789,#24792,#20091,.T.);
#32041=EDGE_CURVE('',#24792,#24791,#6253,.T.);
#32042=EDGE_CURVE('',#24792,#24793,#6254,.T.);
#32043=EDGE_CURVE('',#24790,#24793,#6255,.T.);
#32044=EDGE_CURVE('',#24793,#24788,#20092,.T.);
#32045=EDGE_CURVE('',#24794,#24795,#20093,.T.);
#32046=EDGE_CURVE('',#24796,#24794,#6256,.T.);
#32047=EDGE_CURVE('',#24795,#24796,#6257,.T.);
#32048=EDGE_CURVE('',#24797,#24794,#6258,.T.);
#32049=EDGE_CURVE('',#24797,#24798,#6259,.T.);
#32050=EDGE_CURVE('',#24798,#24796,#6260,.T.);
#32051=EDGE_CURVE('',#24795,#24799,#6261,.T.);
#32052=EDGE_CURVE('',#24798,#24799,#6262,.T.);
#32053=EDGE_CURVE('',#24799,#24797,#20094,.T.);
#32054=EDGE_CURVE('',#24800,#24801,#6263,.T.);
#32055=EDGE_CURVE('',#24801,#24801,#20095,.T.);
#32056=EDGE_CURVE('',#24802,#24803,#6264,.T.);
#32057=EDGE_CURVE('',#24804,#24802,#6265,.T.);
#32058=EDGE_CURVE('',#24805,#24804,#6266,.T.);
#32059=EDGE_CURVE('',#24805,#24803,#6267,.T.);
#32060=EDGE_CURVE('',#24803,#24806,#6268,.T.);
#32061=EDGE_CURVE('',#24807,#24805,#6269,.T.);
#32062=EDGE_CURVE('',#24807,#24806,#6270,.T.);
#32063=EDGE_CURVE('',#24806,#24808,#6271,.T.);
#32064=EDGE_CURVE('',#24809,#24807,#6272,.T.);
#32065=EDGE_CURVE('',#24809,#24808,#6273,.T.);
#32066=EDGE_CURVE('',#24808,#24810,#6274,.T.);
#32067=EDGE_CURVE('',#24811,#24809,#6275,.T.);
#32068=EDGE_CURVE('',#24811,#24810,#6276,.T.);
#32069=EDGE_CURVE('',#24810,#24812,#6277,.T.);
#32070=EDGE_CURVE('',#24813,#24811,#6278,.T.);
#32071=EDGE_CURVE('',#24813,#24812,#6279,.T.);
#32072=EDGE_CURVE('',#24812,#24802,#6280,.T.);
#32073=EDGE_CURVE('',#24804,#24813,#6281,.T.);
#32074=EDGE_CURVE('',#24814,#24814,#20096,.T.);
#32075=EDGE_CURVE('',#24578,#24814,#6282,.T.);
#32076=EDGE_CURVE('',#24592,#24583,#20097,.T.);
#32077=EDGE_CURVE('',#24598,#24589,#20098,.T.);
#32078=EDGE_CURVE('',#24604,#24595,#20099,.T.);
#32079=EDGE_CURVE('',#24610,#24601,#20100,.T.);
#32080=EDGE_CURVE('',#24616,#24607,#20101,.T.);
#32081=EDGE_CURVE('',#24622,#24613,#20102,.T.);
#32082=EDGE_CURVE('',#24628,#24619,#20103,.T.);
#32083=EDGE_CURVE('',#24634,#24625,#20104,.T.);
#32084=EDGE_CURVE('',#24640,#24631,#20105,.T.);
#32085=EDGE_CURVE('',#24646,#24637,#20106,.T.);
#32086=EDGE_CURVE('',#24652,#24643,#20107,.T.);
#32087=EDGE_CURVE('',#24658,#24649,#20108,.T.);
#32088=EDGE_CURVE('',#24664,#24655,#20109,.T.);
#32089=EDGE_CURVE('',#24670,#24661,#20110,.T.);
#32090=EDGE_CURVE('',#24676,#24667,#20111,.T.);
#32091=EDGE_CURVE('',#24682,#24673,#20112,.T.);
#32092=EDGE_CURVE('',#24689,#24679,#20113,.T.);
#32093=EDGE_CURVE('',#24691,#24581,#6283,.T.);
#32094=EDGE_CURVE('',#24696,#24685,#20114,.T.);
#32095=EDGE_CURVE('',#24702,#24693,#20115,.T.);
#32096=EDGE_CURVE('',#24708,#24699,#20116,.T.);
#32097=EDGE_CURVE('',#24714,#24705,#20117,.T.);
#32098=EDGE_CURVE('',#24720,#24711,#20118,.T.);
#32099=EDGE_CURVE('',#24726,#24717,#20119,.T.);
#32100=EDGE_CURVE('',#24732,#24723,#20120,.T.);
#32101=EDGE_CURVE('',#24738,#24729,#20121,.T.);
#32102=EDGE_CURVE('',#24744,#24735,#20122,.T.);
#32103=EDGE_CURVE('',#24750,#24741,#20123,.T.);
#32104=EDGE_CURVE('',#24756,#24747,#20124,.T.);
#32105=EDGE_CURVE('',#24762,#24753,#20125,.T.);
#32106=EDGE_CURVE('',#24768,#24759,#20126,.T.);
#32107=EDGE_CURVE('',#24774,#24765,#20127,.T.);
#32108=EDGE_CURVE('',#24780,#24771,#20128,.T.);
#32109=EDGE_CURVE('',#24786,#24777,#20129,.T.);
#32110=EDGE_CURVE('',#24792,#24783,#20130,.T.);
#32111=EDGE_CURVE('',#24795,#24789,#20131,.T.);
#32112=EDGE_CURVE('',#24586,#24794,#20132,.T.);
#32113=EDGE_CURVE('',#24815,#24815,#20133,.T.);
#32114=EDGE_CURVE('',#24815,#24688,#6284,.T.);
#45503=ORIENTED_EDGE('',*,*,#31613,.F.);
#45504=ORIENTED_EDGE('',*,*,#31614,.T.);
#45505=ORIENTED_EDGE('',*,*,#31615,.T.);
#45506=ORIENTED_EDGE('',*,*,#31616,.T.);
#45507=ORIENTED_EDGE('',*,*,#31617,.F.);
#45508=ORIENTED_EDGE('',*,*,#31618,.T.);
#45509=ORIENTED_EDGE('',*,*,#31613,.T.);
#45510=ORIENTED_EDGE('',*,*,#31619,.T.);
#45511=ORIENTED_EDGE('',*,*,#31620,.F.);
#45512=ORIENTED_EDGE('',*,*,#31621,.T.);
#45513=ORIENTED_EDGE('',*,*,#31617,.T.);
#45514=ORIENTED_EDGE('',*,*,#31622,.T.);
#45515=ORIENTED_EDGE('',*,*,#31623,.F.);
#45516=ORIENTED_EDGE('',*,*,#31624,.T.);
#45517=ORIENTED_EDGE('',*,*,#31620,.T.);
#45518=ORIENTED_EDGE('',*,*,#31625,.T.);
#45519=ORIENTED_EDGE('',*,*,#31626,.F.);
#45520=ORIENTED_EDGE('',*,*,#31627,.T.);
#45521=ORIENTED_EDGE('',*,*,#31623,.T.);
#45522=ORIENTED_EDGE('',*,*,#31628,.T.);
#45523=ORIENTED_EDGE('',*,*,#31629,.F.);
#45524=ORIENTED_EDGE('',*,*,#31630,.T.);
#45525=ORIENTED_EDGE('',*,*,#31626,.T.);
#45526=ORIENTED_EDGE('',*,*,#31631,.T.);
#45527=ORIENTED_EDGE('',*,*,#31632,.F.);
#45528=ORIENTED_EDGE('',*,*,#31633,.T.);
#45529=ORIENTED_EDGE('',*,*,#31629,.T.);
#45530=ORIENTED_EDGE('',*,*,#31634,.T.);
#45531=ORIENTED_EDGE('',*,*,#31635,.F.);
#45532=ORIENTED_EDGE('',*,*,#31636,.T.);
#45533=ORIENTED_EDGE('',*,*,#31632,.T.);
#45534=ORIENTED_EDGE('',*,*,#31637,.T.);
#45535=ORIENTED_EDGE('',*,*,#31638,.F.);
#45536=ORIENTED_EDGE('',*,*,#31639,.T.);
#45537=ORIENTED_EDGE('',*,*,#31635,.T.);
#45538=ORIENTED_EDGE('',*,*,#31640,.T.);
#45539=ORIENTED_EDGE('',*,*,#31641,.F.);
#45540=ORIENTED_EDGE('',*,*,#31642,.T.);
#45541=ORIENTED_EDGE('',*,*,#31638,.T.);
#45542=ORIENTED_EDGE('',*,*,#31643,.T.);
#45543=ORIENTED_EDGE('',*,*,#31644,.F.);
#45544=ORIENTED_EDGE('',*,*,#31645,.T.);
#45545=ORIENTED_EDGE('',*,*,#31641,.T.);
#45546=ORIENTED_EDGE('',*,*,#31646,.T.);
#45547=ORIENTED_EDGE('',*,*,#31647,.F.);
#45548=ORIENTED_EDGE('',*,*,#31648,.T.);
#45549=ORIENTED_EDGE('',*,*,#31644,.T.);
#45550=ORIENTED_EDGE('',*,*,#31649,.T.);
#45551=ORIENTED_EDGE('',*,*,#31650,.F.);
#45552=ORIENTED_EDGE('',*,*,#31651,.T.);
#45553=ORIENTED_EDGE('',*,*,#31647,.T.);
#45554=ORIENTED_EDGE('',*,*,#31652,.T.);
#45555=ORIENTED_EDGE('',*,*,#31653,.F.);
#45556=ORIENTED_EDGE('',*,*,#31654,.T.);
#45557=ORIENTED_EDGE('',*,*,#31650,.T.);
#45558=ORIENTED_EDGE('',*,*,#31655,.T.);
#45559=ORIENTED_EDGE('',*,*,#31656,.F.);
#45560=ORIENTED_EDGE('',*,*,#31657,.T.);
#45561=ORIENTED_EDGE('',*,*,#31653,.T.);
#45562=ORIENTED_EDGE('',*,*,#31658,.T.);
#45563=ORIENTED_EDGE('',*,*,#31659,.F.);
#45564=ORIENTED_EDGE('',*,*,#31660,.T.);
#45565=ORIENTED_EDGE('',*,*,#31656,.T.);
#45566=ORIENTED_EDGE('',*,*,#31661,.T.);
#45567=ORIENTED_EDGE('',*,*,#31662,.F.);
#45568=ORIENTED_EDGE('',*,*,#31663,.T.);
#45569=ORIENTED_EDGE('',*,*,#31664,.F.);
#45570=ORIENTED_EDGE('',*,*,#31665,.F.);
#45571=ORIENTED_EDGE('',*,*,#31666,.T.);
#45572=ORIENTED_EDGE('',*,*,#31662,.T.);
#45573=ORIENTED_EDGE('',*,*,#31667,.F.);
#45574=ORIENTED_EDGE('',*,*,#31668,.F.);
#45575=ORIENTED_EDGE('',*,*,#31669,.F.);
#45576=ORIENTED_EDGE('',*,*,#31670,.T.);
#45577=ORIENTED_EDGE('',*,*,#31665,.T.);
#45578=ORIENTED_EDGE('',*,*,#31671,.F.);
#45579=ORIENTED_EDGE('',*,*,#31672,.F.);
#45580=ORIENTED_EDGE('',*,*,#31673,.T.);
#45581=ORIENTED_EDGE('',*,*,#31669,.T.);
#45582=ORIENTED_EDGE('',*,*,#31674,.F.);
#45583=ORIENTED_EDGE('',*,*,#31675,.F.);
#45584=ORIENTED_EDGE('',*,*,#31676,.T.);
#45585=ORIENTED_EDGE('',*,*,#31672,.T.);
#45586=ORIENTED_EDGE('',*,*,#31677,.F.);
#45587=ORIENTED_EDGE('',*,*,#31678,.F.);
#45588=ORIENTED_EDGE('',*,*,#31679,.T.);
#45589=ORIENTED_EDGE('',*,*,#31675,.T.);
#45590=ORIENTED_EDGE('',*,*,#31680,.F.);
#45591=ORIENTED_EDGE('',*,*,#31681,.F.);
#45592=ORIENTED_EDGE('',*,*,#31682,.T.);
#45593=ORIENTED_EDGE('',*,*,#31678,.T.);
#45594=ORIENTED_EDGE('',*,*,#31683,.F.);
#45595=ORIENTED_EDGE('',*,*,#31684,.F.);
#45596=ORIENTED_EDGE('',*,*,#31685,.T.);
#45597=ORIENTED_EDGE('',*,*,#31681,.T.);
#45598=ORIENTED_EDGE('',*,*,#31686,.F.);
#45599=ORIENTED_EDGE('',*,*,#31687,.F.);
#45600=ORIENTED_EDGE('',*,*,#31688,.T.);
#45601=ORIENTED_EDGE('',*,*,#31684,.T.);
#45602=ORIENTED_EDGE('',*,*,#31689,.F.);
#45603=ORIENTED_EDGE('',*,*,#31690,.F.);
#45604=ORIENTED_EDGE('',*,*,#31691,.T.);
#45605=ORIENTED_EDGE('',*,*,#31687,.T.);
#45606=ORIENTED_EDGE('',*,*,#31692,.F.);
#45607=ORIENTED_EDGE('',*,*,#31693,.F.);
#45608=ORIENTED_EDGE('',*,*,#31694,.T.);
#45609=ORIENTED_EDGE('',*,*,#31690,.T.);
#45610=ORIENTED_EDGE('',*,*,#31695,.F.);
#45611=ORIENTED_EDGE('',*,*,#31696,.F.);
#45612=ORIENTED_EDGE('',*,*,#31697,.T.);
#45613=ORIENTED_EDGE('',*,*,#31693,.T.);
#45614=ORIENTED_EDGE('',*,*,#31698,.F.);
#45615=ORIENTED_EDGE('',*,*,#31699,.F.);
#45616=ORIENTED_EDGE('',*,*,#31700,.T.);
#45617=ORIENTED_EDGE('',*,*,#31696,.T.);
#45618=ORIENTED_EDGE('',*,*,#31701,.F.);
#45619=ORIENTED_EDGE('',*,*,#31702,.F.);
#45620=ORIENTED_EDGE('',*,*,#31703,.T.);
#45621=ORIENTED_EDGE('',*,*,#31699,.T.);
#45622=ORIENTED_EDGE('',*,*,#31704,.F.);
#45623=ORIENTED_EDGE('',*,*,#31705,.F.);
#45624=ORIENTED_EDGE('',*,*,#31706,.T.);
#45625=ORIENTED_EDGE('',*,*,#31702,.T.);
#45626=ORIENTED_EDGE('',*,*,#31707,.F.);
#45627=ORIENTED_EDGE('',*,*,#31708,.F.);
#45628=ORIENTED_EDGE('',*,*,#31709,.T.);
#45629=ORIENTED_EDGE('',*,*,#31705,.T.);
#45630=ORIENTED_EDGE('',*,*,#31710,.F.);
#45631=ORIENTED_EDGE('',*,*,#31667,.T.);
#45632=ORIENTED_EDGE('',*,*,#31664,.T.);
#45633=ORIENTED_EDGE('',*,*,#31711,.T.);
#45634=ORIENTED_EDGE('',*,*,#31712,.F.);
#45635=ORIENTED_EDGE('',*,*,#31713,.F.);
#45636=ORIENTED_EDGE('',*,*,#31714,.T.);
#45637=ORIENTED_EDGE('',*,*,#31714,.F.);
#45638=ORIENTED_EDGE('',*,*,#31715,.F.);
#45639=ORIENTED_EDGE('',*,*,#31661,.F.);
#45640=ORIENTED_EDGE('',*,*,#31658,.F.);
#45641=ORIENTED_EDGE('',*,*,#31655,.F.);
#45642=ORIENTED_EDGE('',*,*,#31652,.F.);
#45643=ORIENTED_EDGE('',*,*,#31649,.F.);
#45644=ORIENTED_EDGE('',*,*,#31646,.F.);
#45645=ORIENTED_EDGE('',*,*,#31643,.F.);
#45646=ORIENTED_EDGE('',*,*,#31640,.F.);
#45647=ORIENTED_EDGE('',*,*,#31637,.F.);
#45648=ORIENTED_EDGE('',*,*,#31634,.F.);
#45649=ORIENTED_EDGE('',*,*,#31631,.F.);
#45650=ORIENTED_EDGE('',*,*,#31628,.F.);
#45651=ORIENTED_EDGE('',*,*,#31625,.F.);
#45652=ORIENTED_EDGE('',*,*,#31622,.F.);
#45653=ORIENTED_EDGE('',*,*,#31619,.F.);
#45654=ORIENTED_EDGE('',*,*,#31616,.F.);
#45655=ORIENTED_EDGE('',*,*,#31716,.F.);
#45656=ORIENTED_EDGE('',*,*,#31717,.T.);
#45657=ORIENTED_EDGE('',*,*,#31710,.T.);
#45658=ORIENTED_EDGE('',*,*,#31707,.T.);
#45659=ORIENTED_EDGE('',*,*,#31704,.T.);
#45660=ORIENTED_EDGE('',*,*,#31701,.T.);
#45661=ORIENTED_EDGE('',*,*,#31698,.T.);
#45662=ORIENTED_EDGE('',*,*,#31695,.T.);
#45663=ORIENTED_EDGE('',*,*,#31692,.T.);
#45664=ORIENTED_EDGE('',*,*,#31689,.T.);
#45665=ORIENTED_EDGE('',*,*,#31686,.T.);
#45666=ORIENTED_EDGE('',*,*,#31683,.T.);
#45667=ORIENTED_EDGE('',*,*,#31680,.T.);
#45668=ORIENTED_EDGE('',*,*,#31677,.T.);
#45669=ORIENTED_EDGE('',*,*,#31674,.T.);
#45670=ORIENTED_EDGE('',*,*,#31671,.T.);
#45671=ORIENTED_EDGE('',*,*,#31668,.T.);
#45672=ORIENTED_EDGE('',*,*,#31718,.T.);
#45673=ORIENTED_EDGE('',*,*,#31719,.T.);
#45674=ORIENTED_EDGE('',*,*,#31720,.T.);
#45675=ORIENTED_EDGE('',*,*,#31721,.T.);
#45676=ORIENTED_EDGE('',*,*,#31716,.T.);
#45677=ORIENTED_EDGE('',*,*,#31708,.T.);
#45678=ORIENTED_EDGE('',*,*,#31717,.F.);
#45679=ORIENTED_EDGE('',*,*,#31721,.F.);
#45680=ORIENTED_EDGE('',*,*,#31722,.T.);
#45681=ORIENTED_EDGE('',*,*,#31711,.F.);
#45682=ORIENTED_EDGE('',*,*,#31663,.F.);
#45683=ORIENTED_EDGE('',*,*,#31666,.F.);
#45684=ORIENTED_EDGE('',*,*,#31670,.F.);
#45685=ORIENTED_EDGE('',*,*,#31673,.F.);
#45686=ORIENTED_EDGE('',*,*,#31676,.F.);
#45687=ORIENTED_EDGE('',*,*,#31679,.F.);
#45688=ORIENTED_EDGE('',*,*,#31682,.F.);
#45689=ORIENTED_EDGE('',*,*,#31685,.F.);
#45690=ORIENTED_EDGE('',*,*,#31688,.F.);
#45691=ORIENTED_EDGE('',*,*,#31691,.F.);
#45692=ORIENTED_EDGE('',*,*,#31694,.F.);
#45693=ORIENTED_EDGE('',*,*,#31697,.F.);
#45694=ORIENTED_EDGE('',*,*,#31700,.F.);
#45695=ORIENTED_EDGE('',*,*,#31703,.F.);
#45696=ORIENTED_EDGE('',*,*,#31706,.F.);
#45697=ORIENTED_EDGE('',*,*,#31709,.F.);
#45698=ORIENTED_EDGE('',*,*,#31722,.F.);
#45699=ORIENTED_EDGE('',*,*,#31720,.F.);
#45700=ORIENTED_EDGE('',*,*,#31614,.F.);
#45701=ORIENTED_EDGE('',*,*,#31618,.F.);
#45702=ORIENTED_EDGE('',*,*,#31621,.F.);
#45703=ORIENTED_EDGE('',*,*,#31624,.F.);
#45704=ORIENTED_EDGE('',*,*,#31627,.F.);
#45705=ORIENTED_EDGE('',*,*,#31630,.F.);
#45706=ORIENTED_EDGE('',*,*,#31633,.F.);
#45707=ORIENTED_EDGE('',*,*,#31636,.F.);
#45708=ORIENTED_EDGE('',*,*,#31639,.F.);
#45709=ORIENTED_EDGE('',*,*,#31642,.F.);
#45710=ORIENTED_EDGE('',*,*,#31645,.F.);
#45711=ORIENTED_EDGE('',*,*,#31648,.F.);
#45712=ORIENTED_EDGE('',*,*,#31651,.F.);
#45713=ORIENTED_EDGE('',*,*,#31654,.F.);
#45714=ORIENTED_EDGE('',*,*,#31657,.F.);
#45715=ORIENTED_EDGE('',*,*,#31660,.F.);
#45716=ORIENTED_EDGE('',*,*,#31723,.F.);
#45717=ORIENTED_EDGE('',*,*,#31713,.T.);
#45718=ORIENTED_EDGE('',*,*,#31724,.T.);
#45719=ORIENTED_EDGE('',*,*,#31725,.T.);
#45720=ORIENTED_EDGE('',*,*,#31724,.F.);
#45721=ORIENTED_EDGE('',*,*,#31712,.T.);
#45722=ORIENTED_EDGE('',*,*,#31726,.T.);
#45723=ORIENTED_EDGE('',*,*,#31659,.T.);
#45724=ORIENTED_EDGE('',*,*,#31715,.T.);
#45725=ORIENTED_EDGE('',*,*,#31726,.F.);
#45726=ORIENTED_EDGE('',*,*,#31723,.T.);
#45727=ORIENTED_EDGE('',*,*,#31727,.F.);
#45728=ORIENTED_EDGE('',*,*,#31725,.F.);
#45729=ORIENTED_EDGE('',*,*,#31728,.F.);
#45730=ORIENTED_EDGE('',*,*,#31729,.T.);
#45731=ORIENTED_EDGE('',*,*,#31730,.T.);
#45732=ORIENTED_EDGE('',*,*,#31731,.T.);
#45733=ORIENTED_EDGE('',*,*,#31732,.F.);
#45734=ORIENTED_EDGE('',*,*,#31731,.F.);
#45735=ORIENTED_EDGE('',*,*,#31733,.F.);
#45736=ORIENTED_EDGE('',*,*,#31734,.F.);
#45737=ORIENTED_EDGE('',*,*,#31733,.T.);
#45738=ORIENTED_EDGE('',*,*,#31730,.F.);
#45739=ORIENTED_EDGE('',*,*,#31735,.T.);
#45740=ORIENTED_EDGE('',*,*,#31736,.F.);
#45741=ORIENTED_EDGE('',*,*,#31735,.F.);
#45742=ORIENTED_EDGE('',*,*,#31729,.F.);
#45743=ORIENTED_EDGE('',*,*,#31737,.F.);
#45744=ORIENTED_EDGE('',*,*,#31738,.T.);
#45745=ORIENTED_EDGE('',*,*,#31739,.T.);
#45746=ORIENTED_EDGE('',*,*,#31740,.T.);
#45747=ORIENTED_EDGE('',*,*,#31741,.F.);
#45748=ORIENTED_EDGE('',*,*,#31740,.F.);
#45749=ORIENTED_EDGE('',*,*,#31742,.F.);
#45750=ORIENTED_EDGE('',*,*,#31743,.F.);
#45751=ORIENTED_EDGE('',*,*,#31742,.T.);
#45752=ORIENTED_EDGE('',*,*,#31739,.F.);
#45753=ORIENTED_EDGE('',*,*,#31744,.T.);
#45754=ORIENTED_EDGE('',*,*,#31745,.F.);
#45755=ORIENTED_EDGE('',*,*,#31744,.F.);
#45756=ORIENTED_EDGE('',*,*,#31738,.F.);
#45757=ORIENTED_EDGE('',*,*,#31746,.F.);
#45758=ORIENTED_EDGE('',*,*,#31747,.T.);
#45759=ORIENTED_EDGE('',*,*,#31748,.T.);
#45760=ORIENTED_EDGE('',*,*,#31749,.T.);
#45761=ORIENTED_EDGE('',*,*,#31750,.F.);
#45762=ORIENTED_EDGE('',*,*,#31749,.F.);
#45763=ORIENTED_EDGE('',*,*,#31751,.F.);
#45764=ORIENTED_EDGE('',*,*,#31752,.F.);
#45765=ORIENTED_EDGE('',*,*,#31751,.T.);
#45766=ORIENTED_EDGE('',*,*,#31748,.F.);
#45767=ORIENTED_EDGE('',*,*,#31753,.T.);
#45768=ORIENTED_EDGE('',*,*,#31754,.F.);
#45769=ORIENTED_EDGE('',*,*,#31753,.F.);
#45770=ORIENTED_EDGE('',*,*,#31747,.F.);
#45771=ORIENTED_EDGE('',*,*,#31755,.F.);
#45772=ORIENTED_EDGE('',*,*,#31756,.T.);
#45773=ORIENTED_EDGE('',*,*,#31757,.T.);
#45774=ORIENTED_EDGE('',*,*,#31758,.T.);
#45775=ORIENTED_EDGE('',*,*,#31759,.F.);
#45776=ORIENTED_EDGE('',*,*,#31758,.F.);
#45777=ORIENTED_EDGE('',*,*,#31760,.F.);
#45778=ORIENTED_EDGE('',*,*,#31761,.F.);
#45779=ORIENTED_EDGE('',*,*,#31760,.T.);
#45780=ORIENTED_EDGE('',*,*,#31757,.F.);
#45781=ORIENTED_EDGE('',*,*,#31762,.T.);
#45782=ORIENTED_EDGE('',*,*,#31763,.F.);
#45783=ORIENTED_EDGE('',*,*,#31762,.F.);
#45784=ORIENTED_EDGE('',*,*,#31756,.F.);
#45785=ORIENTED_EDGE('',*,*,#31764,.F.);
#45786=ORIENTED_EDGE('',*,*,#31765,.T.);
#45787=ORIENTED_EDGE('',*,*,#31766,.T.);
#45788=ORIENTED_EDGE('',*,*,#31767,.T.);
#45789=ORIENTED_EDGE('',*,*,#31768,.F.);
#45790=ORIENTED_EDGE('',*,*,#31767,.F.);
#45791=ORIENTED_EDGE('',*,*,#31769,.F.);
#45792=ORIENTED_EDGE('',*,*,#31770,.F.);
#45793=ORIENTED_EDGE('',*,*,#31769,.T.);
#45794=ORIENTED_EDGE('',*,*,#31766,.F.);
#45795=ORIENTED_EDGE('',*,*,#31771,.T.);
#45796=ORIENTED_EDGE('',*,*,#31772,.F.);
#45797=ORIENTED_EDGE('',*,*,#31771,.F.);
#45798=ORIENTED_EDGE('',*,*,#31765,.F.);
#45799=ORIENTED_EDGE('',*,*,#31773,.F.);
#45800=ORIENTED_EDGE('',*,*,#31774,.T.);
#45801=ORIENTED_EDGE('',*,*,#31775,.T.);
#45802=ORIENTED_EDGE('',*,*,#31776,.T.);
#45803=ORIENTED_EDGE('',*,*,#31777,.F.);
#45804=ORIENTED_EDGE('',*,*,#31776,.F.);
#45805=ORIENTED_EDGE('',*,*,#31778,.F.);
#45806=ORIENTED_EDGE('',*,*,#31779,.F.);
#45807=ORIENTED_EDGE('',*,*,#31778,.T.);
#45808=ORIENTED_EDGE('',*,*,#31775,.F.);
#45809=ORIENTED_EDGE('',*,*,#31780,.T.);
#45810=ORIENTED_EDGE('',*,*,#31781,.F.);
#45811=ORIENTED_EDGE('',*,*,#31780,.F.);
#45812=ORIENTED_EDGE('',*,*,#31774,.F.);
#45813=ORIENTED_EDGE('',*,*,#31782,.F.);
#45814=ORIENTED_EDGE('',*,*,#31783,.T.);
#45815=ORIENTED_EDGE('',*,*,#31784,.T.);
#45816=ORIENTED_EDGE('',*,*,#31785,.T.);
#45817=ORIENTED_EDGE('',*,*,#31786,.F.);
#45818=ORIENTED_EDGE('',*,*,#31785,.F.);
#45819=ORIENTED_EDGE('',*,*,#31787,.F.);
#45820=ORIENTED_EDGE('',*,*,#31788,.F.);
#45821=ORIENTED_EDGE('',*,*,#31787,.T.);
#45822=ORIENTED_EDGE('',*,*,#31784,.F.);
#45823=ORIENTED_EDGE('',*,*,#31789,.T.);
#45824=ORIENTED_EDGE('',*,*,#31790,.F.);
#45825=ORIENTED_EDGE('',*,*,#31789,.F.);
#45826=ORIENTED_EDGE('',*,*,#31783,.F.);
#45827=ORIENTED_EDGE('',*,*,#31791,.F.);
#45828=ORIENTED_EDGE('',*,*,#31792,.T.);
#45829=ORIENTED_EDGE('',*,*,#31793,.T.);
#45830=ORIENTED_EDGE('',*,*,#31794,.T.);
#45831=ORIENTED_EDGE('',*,*,#31795,.F.);
#45832=ORIENTED_EDGE('',*,*,#31794,.F.);
#45833=ORIENTED_EDGE('',*,*,#31796,.F.);
#45834=ORIENTED_EDGE('',*,*,#31797,.F.);
#45835=ORIENTED_EDGE('',*,*,#31796,.T.);
#45836=ORIENTED_EDGE('',*,*,#31793,.F.);
#45837=ORIENTED_EDGE('',*,*,#31798,.T.);
#45838=ORIENTED_EDGE('',*,*,#31799,.F.);
#45839=ORIENTED_EDGE('',*,*,#31798,.F.);
#45840=ORIENTED_EDGE('',*,*,#31792,.F.);
#45841=ORIENTED_EDGE('',*,*,#31800,.F.);
#45842=ORIENTED_EDGE('',*,*,#31801,.T.);
#45843=ORIENTED_EDGE('',*,*,#31802,.T.);
#45844=ORIENTED_EDGE('',*,*,#31803,.T.);
#45845=ORIENTED_EDGE('',*,*,#31804,.F.);
#45846=ORIENTED_EDGE('',*,*,#31803,.F.);
#45847=ORIENTED_EDGE('',*,*,#31805,.F.);
#45848=ORIENTED_EDGE('',*,*,#31806,.F.);
#45849=ORIENTED_EDGE('',*,*,#31805,.T.);
#45850=ORIENTED_EDGE('',*,*,#31802,.F.);
#45851=ORIENTED_EDGE('',*,*,#31807,.T.);
#45852=ORIENTED_EDGE('',*,*,#31808,.F.);
#45853=ORIENTED_EDGE('',*,*,#31807,.F.);
#45854=ORIENTED_EDGE('',*,*,#31801,.F.);
#45855=ORIENTED_EDGE('',*,*,#31809,.F.);
#45856=ORIENTED_EDGE('',*,*,#31810,.T.);
#45857=ORIENTED_EDGE('',*,*,#31811,.T.);
#45858=ORIENTED_EDGE('',*,*,#31812,.T.);
#45859=ORIENTED_EDGE('',*,*,#31813,.F.);
#45860=ORIENTED_EDGE('',*,*,#31812,.F.);
#45861=ORIENTED_EDGE('',*,*,#31814,.F.);
#45862=ORIENTED_EDGE('',*,*,#31815,.F.);
#45863=ORIENTED_EDGE('',*,*,#31814,.T.);
#45864=ORIENTED_EDGE('',*,*,#31811,.F.);
#45865=ORIENTED_EDGE('',*,*,#31816,.T.);
#45866=ORIENTED_EDGE('',*,*,#31817,.F.);
#45867=ORIENTED_EDGE('',*,*,#31816,.F.);
#45868=ORIENTED_EDGE('',*,*,#31810,.F.);
#45869=ORIENTED_EDGE('',*,*,#31818,.F.);
#45870=ORIENTED_EDGE('',*,*,#31819,.T.);
#45871=ORIENTED_EDGE('',*,*,#31820,.T.);
#45872=ORIENTED_EDGE('',*,*,#31821,.T.);
#45873=ORIENTED_EDGE('',*,*,#31822,.F.);
#45874=ORIENTED_EDGE('',*,*,#31821,.F.);
#45875=ORIENTED_EDGE('',*,*,#31823,.F.);
#45876=ORIENTED_EDGE('',*,*,#31824,.F.);
#45877=ORIENTED_EDGE('',*,*,#31823,.T.);
#45878=ORIENTED_EDGE('',*,*,#31820,.F.);
#45879=ORIENTED_EDGE('',*,*,#31825,.T.);
#45880=ORIENTED_EDGE('',*,*,#31826,.F.);
#45881=ORIENTED_EDGE('',*,*,#31825,.F.);
#45882=ORIENTED_EDGE('',*,*,#31819,.F.);
#45883=ORIENTED_EDGE('',*,*,#31827,.F.);
#45884=ORIENTED_EDGE('',*,*,#31828,.T.);
#45885=ORIENTED_EDGE('',*,*,#31829,.T.);
#45886=ORIENTED_EDGE('',*,*,#31830,.T.);
#45887=ORIENTED_EDGE('',*,*,#31831,.F.);
#45888=ORIENTED_EDGE('',*,*,#31830,.F.);
#45889=ORIENTED_EDGE('',*,*,#31832,.F.);
#45890=ORIENTED_EDGE('',*,*,#31833,.F.);
#45891=ORIENTED_EDGE('',*,*,#31832,.T.);
#45892=ORIENTED_EDGE('',*,*,#31829,.F.);
#45893=ORIENTED_EDGE('',*,*,#31834,.T.);
#45894=ORIENTED_EDGE('',*,*,#31835,.F.);
#45895=ORIENTED_EDGE('',*,*,#31834,.F.);
#45896=ORIENTED_EDGE('',*,*,#31828,.F.);
#45897=ORIENTED_EDGE('',*,*,#31836,.F.);
#45898=ORIENTED_EDGE('',*,*,#31837,.T.);
#45899=ORIENTED_EDGE('',*,*,#31838,.T.);
#45900=ORIENTED_EDGE('',*,*,#31839,.T.);
#45901=ORIENTED_EDGE('',*,*,#31840,.F.);
#45902=ORIENTED_EDGE('',*,*,#31839,.F.);
#45903=ORIENTED_EDGE('',*,*,#31841,.F.);
#45904=ORIENTED_EDGE('',*,*,#31842,.F.);
#45905=ORIENTED_EDGE('',*,*,#31841,.T.);
#45906=ORIENTED_EDGE('',*,*,#31838,.F.);
#45907=ORIENTED_EDGE('',*,*,#31843,.T.);
#45908=ORIENTED_EDGE('',*,*,#31844,.F.);
#45909=ORIENTED_EDGE('',*,*,#31843,.F.);
#45910=ORIENTED_EDGE('',*,*,#31837,.F.);
#45911=ORIENTED_EDGE('',*,*,#31845,.F.);
#45912=ORIENTED_EDGE('',*,*,#31846,.T.);
#45913=ORIENTED_EDGE('',*,*,#31847,.T.);
#45914=ORIENTED_EDGE('',*,*,#31848,.T.);
#45915=ORIENTED_EDGE('',*,*,#31849,.F.);
#45916=ORIENTED_EDGE('',*,*,#31848,.F.);
#45917=ORIENTED_EDGE('',*,*,#31850,.F.);
#45918=ORIENTED_EDGE('',*,*,#31851,.F.);
#45919=ORIENTED_EDGE('',*,*,#31850,.T.);
#45920=ORIENTED_EDGE('',*,*,#31847,.F.);
#45921=ORIENTED_EDGE('',*,*,#31852,.T.);
#45922=ORIENTED_EDGE('',*,*,#31853,.F.);
#45923=ORIENTED_EDGE('',*,*,#31852,.F.);
#45924=ORIENTED_EDGE('',*,*,#31846,.F.);
#45925=ORIENTED_EDGE('',*,*,#31854,.F.);
#45926=ORIENTED_EDGE('',*,*,#31855,.T.);
#45927=ORIENTED_EDGE('',*,*,#31856,.T.);
#45928=ORIENTED_EDGE('',*,*,#31857,.T.);
#45929=ORIENTED_EDGE('',*,*,#31858,.F.);
#45930=ORIENTED_EDGE('',*,*,#31857,.F.);
#45931=ORIENTED_EDGE('',*,*,#31859,.F.);
#45932=ORIENTED_EDGE('',*,*,#31860,.F.);
#45933=ORIENTED_EDGE('',*,*,#31859,.T.);
#45934=ORIENTED_EDGE('',*,*,#31856,.F.);
#45935=ORIENTED_EDGE('',*,*,#31861,.T.);
#45936=ORIENTED_EDGE('',*,*,#31862,.F.);
#45937=ORIENTED_EDGE('',*,*,#31861,.F.);
#45938=ORIENTED_EDGE('',*,*,#31855,.F.);
#45939=ORIENTED_EDGE('',*,*,#31863,.F.);
#45940=ORIENTED_EDGE('',*,*,#31864,.T.);
#45941=ORIENTED_EDGE('',*,*,#31865,.T.);
#45942=ORIENTED_EDGE('',*,*,#31866,.T.);
#45943=ORIENTED_EDGE('',*,*,#31867,.F.);
#45944=ORIENTED_EDGE('',*,*,#31866,.F.);
#45945=ORIENTED_EDGE('',*,*,#31868,.F.);
#45946=ORIENTED_EDGE('',*,*,#31869,.F.);
#45947=ORIENTED_EDGE('',*,*,#31868,.T.);
#45948=ORIENTED_EDGE('',*,*,#31865,.F.);
#45949=ORIENTED_EDGE('',*,*,#31870,.T.);
#45950=ORIENTED_EDGE('',*,*,#31871,.F.);
#45951=ORIENTED_EDGE('',*,*,#31870,.F.);
#45952=ORIENTED_EDGE('',*,*,#31864,.F.);
#45953=ORIENTED_EDGE('',*,*,#31872,.F.);
#45954=ORIENTED_EDGE('',*,*,#31873,.T.);
#45955=ORIENTED_EDGE('',*,*,#31874,.T.);
#45956=ORIENTED_EDGE('',*,*,#31875,.T.);
#45957=ORIENTED_EDGE('',*,*,#31876,.F.);
#45958=ORIENTED_EDGE('',*,*,#31875,.F.);
#45959=ORIENTED_EDGE('',*,*,#31877,.F.);
#45960=ORIENTED_EDGE('',*,*,#31878,.F.);
#45961=ORIENTED_EDGE('',*,*,#31877,.T.);
#45962=ORIENTED_EDGE('',*,*,#31874,.F.);
#45963=ORIENTED_EDGE('',*,*,#31879,.T.);
#45964=ORIENTED_EDGE('',*,*,#31880,.F.);
#45965=ORIENTED_EDGE('',*,*,#31879,.F.);
#45966=ORIENTED_EDGE('',*,*,#31873,.F.);
#45967=ORIENTED_EDGE('',*,*,#31881,.F.);
#45968=ORIENTED_EDGE('',*,*,#31882,.T.);
#45969=ORIENTED_EDGE('',*,*,#31883,.T.);
#45970=ORIENTED_EDGE('',*,*,#31884,.T.);
#45971=ORIENTED_EDGE('',*,*,#31885,.F.);
#45972=ORIENTED_EDGE('',*,*,#31884,.F.);
#45973=ORIENTED_EDGE('',*,*,#31886,.F.);
#45974=ORIENTED_EDGE('',*,*,#31887,.F.);
#45975=ORIENTED_EDGE('',*,*,#31888,.F.);
#45976=ORIENTED_EDGE('',*,*,#31886,.T.);
#45977=ORIENTED_EDGE('',*,*,#31883,.F.);
#45978=ORIENTED_EDGE('',*,*,#31889,.T.);
#45979=ORIENTED_EDGE('',*,*,#31890,.F.);
#45980=ORIENTED_EDGE('',*,*,#31889,.F.);
#45981=ORIENTED_EDGE('',*,*,#31882,.F.);
#45982=ORIENTED_EDGE('',*,*,#31891,.F.);
#45983=ORIENTED_EDGE('',*,*,#31892,.F.);
#45984=ORIENTED_EDGE('',*,*,#31893,.T.);
#45985=ORIENTED_EDGE('',*,*,#31894,.T.);
#45986=ORIENTED_EDGE('',*,*,#31895,.T.);
#45987=ORIENTED_EDGE('',*,*,#31896,.F.);
#45988=ORIENTED_EDGE('',*,*,#31895,.F.);
#45989=ORIENTED_EDGE('',*,*,#31897,.F.);
#45990=ORIENTED_EDGE('',*,*,#31898,.F.);
#45991=ORIENTED_EDGE('',*,*,#31897,.T.);
#45992=ORIENTED_EDGE('',*,*,#31894,.F.);
#45993=ORIENTED_EDGE('',*,*,#31899,.T.);
#45994=ORIENTED_EDGE('',*,*,#31900,.F.);
#45995=ORIENTED_EDGE('',*,*,#31899,.F.);
#45996=ORIENTED_EDGE('',*,*,#31893,.F.);
#45997=ORIENTED_EDGE('',*,*,#31901,.F.);
#45998=ORIENTED_EDGE('',*,*,#31902,.T.);
#45999=ORIENTED_EDGE('',*,*,#31903,.T.);
#46000=ORIENTED_EDGE('',*,*,#31904,.T.);
#46001=ORIENTED_EDGE('',*,*,#31905,.F.);
#46002=ORIENTED_EDGE('',*,*,#31904,.F.);
#46003=ORIENTED_EDGE('',*,*,#31906,.F.);
#46004=ORIENTED_EDGE('',*,*,#31907,.F.);
#46005=ORIENTED_EDGE('',*,*,#31906,.T.);
#46006=ORIENTED_EDGE('',*,*,#31903,.F.);
#46007=ORIENTED_EDGE('',*,*,#31908,.T.);
#46008=ORIENTED_EDGE('',*,*,#31909,.F.);
#46009=ORIENTED_EDGE('',*,*,#31908,.F.);
#46010=ORIENTED_EDGE('',*,*,#31902,.F.);
#46011=ORIENTED_EDGE('',*,*,#31910,.F.);
#46012=ORIENTED_EDGE('',*,*,#31911,.T.);
#46013=ORIENTED_EDGE('',*,*,#31912,.T.);
#46014=ORIENTED_EDGE('',*,*,#31913,.T.);
#46015=ORIENTED_EDGE('',*,*,#31914,.F.);
#46016=ORIENTED_EDGE('',*,*,#31913,.F.);
#46017=ORIENTED_EDGE('',*,*,#31915,.F.);
#46018=ORIENTED_EDGE('',*,*,#31916,.F.);
#46019=ORIENTED_EDGE('',*,*,#31915,.T.);
#46020=ORIENTED_EDGE('',*,*,#31912,.F.);
#46021=ORIENTED_EDGE('',*,*,#31917,.T.);
#46022=ORIENTED_EDGE('',*,*,#31918,.F.);
#46023=ORIENTED_EDGE('',*,*,#31917,.F.);
#46024=ORIENTED_EDGE('',*,*,#31911,.F.);
#46025=ORIENTED_EDGE('',*,*,#31919,.F.);
#46026=ORIENTED_EDGE('',*,*,#31920,.T.);
#46027=ORIENTED_EDGE('',*,*,#31921,.T.);
#46028=ORIENTED_EDGE('',*,*,#31922,.T.);
#46029=ORIENTED_EDGE('',*,*,#31923,.F.);
#46030=ORIENTED_EDGE('',*,*,#31922,.F.);
#46031=ORIENTED_EDGE('',*,*,#31924,.F.);
#46032=ORIENTED_EDGE('',*,*,#31925,.F.);
#46033=ORIENTED_EDGE('',*,*,#31924,.T.);
#46034=ORIENTED_EDGE('',*,*,#31921,.F.);
#46035=ORIENTED_EDGE('',*,*,#31926,.T.);
#46036=ORIENTED_EDGE('',*,*,#31927,.F.);
#46037=ORIENTED_EDGE('',*,*,#31926,.F.);
#46038=ORIENTED_EDGE('',*,*,#31920,.F.);
#46039=ORIENTED_EDGE('',*,*,#31928,.F.);
#46040=ORIENTED_EDGE('',*,*,#31929,.T.);
#46041=ORIENTED_EDGE('',*,*,#31930,.T.);
#46042=ORIENTED_EDGE('',*,*,#31931,.T.);
#46043=ORIENTED_EDGE('',*,*,#31932,.F.);
#46044=ORIENTED_EDGE('',*,*,#31931,.F.);
#46045=ORIENTED_EDGE('',*,*,#31933,.F.);
#46046=ORIENTED_EDGE('',*,*,#31934,.F.);
#46047=ORIENTED_EDGE('',*,*,#31933,.T.);
#46048=ORIENTED_EDGE('',*,*,#31930,.F.);
#46049=ORIENTED_EDGE('',*,*,#31935,.T.);
#46050=ORIENTED_EDGE('',*,*,#31936,.F.);
#46051=ORIENTED_EDGE('',*,*,#31935,.F.);
#46052=ORIENTED_EDGE('',*,*,#31929,.F.);
#46053=ORIENTED_EDGE('',*,*,#31937,.F.);
#46054=ORIENTED_EDGE('',*,*,#31938,.T.);
#46055=ORIENTED_EDGE('',*,*,#31939,.T.);
#46056=ORIENTED_EDGE('',*,*,#31940,.T.);
#46057=ORIENTED_EDGE('',*,*,#31941,.F.);
#46058=ORIENTED_EDGE('',*,*,#31940,.F.);
#46059=ORIENTED_EDGE('',*,*,#31942,.F.);
#46060=ORIENTED_EDGE('',*,*,#31943,.F.);
#46061=ORIENTED_EDGE('',*,*,#31942,.T.);
#46062=ORIENTED_EDGE('',*,*,#31939,.F.);
#46063=ORIENTED_EDGE('',*,*,#31944,.T.);
#46064=ORIENTED_EDGE('',*,*,#31945,.F.);
#46065=ORIENTED_EDGE('',*,*,#31944,.F.);
#46066=ORIENTED_EDGE('',*,*,#31938,.F.);
#46067=ORIENTED_EDGE('',*,*,#31946,.F.);
#46068=ORIENTED_EDGE('',*,*,#31947,.T.);
#46069=ORIENTED_EDGE('',*,*,#31948,.T.);
#46070=ORIENTED_EDGE('',*,*,#31949,.T.);
#46071=ORIENTED_EDGE('',*,*,#31950,.F.);
#46072=ORIENTED_EDGE('',*,*,#31949,.F.);
#46073=ORIENTED_EDGE('',*,*,#31951,.F.);
#46074=ORIENTED_EDGE('',*,*,#31952,.F.);
#46075=ORIENTED_EDGE('',*,*,#31951,.T.);
#46076=ORIENTED_EDGE('',*,*,#31948,.F.);
#46077=ORIENTED_EDGE('',*,*,#31953,.T.);
#46078=ORIENTED_EDGE('',*,*,#31954,.F.);
#46079=ORIENTED_EDGE('',*,*,#31953,.F.);
#46080=ORIENTED_EDGE('',*,*,#31947,.F.);
#46081=ORIENTED_EDGE('',*,*,#31955,.F.);
#46082=ORIENTED_EDGE('',*,*,#31956,.T.);
#46083=ORIENTED_EDGE('',*,*,#31957,.T.);
#46084=ORIENTED_EDGE('',*,*,#31958,.T.);
#46085=ORIENTED_EDGE('',*,*,#31959,.F.);
#46086=ORIENTED_EDGE('',*,*,#31958,.F.);
#46087=ORIENTED_EDGE('',*,*,#31960,.F.);
#46088=ORIENTED_EDGE('',*,*,#31961,.F.);
#46089=ORIENTED_EDGE('',*,*,#31960,.T.);
#46090=ORIENTED_EDGE('',*,*,#31957,.F.);
#46091=ORIENTED_EDGE('',*,*,#31962,.T.);
#46092=ORIENTED_EDGE('',*,*,#31963,.F.);
#46093=ORIENTED_EDGE('',*,*,#31962,.F.);
#46094=ORIENTED_EDGE('',*,*,#31956,.F.);
#46095=ORIENTED_EDGE('',*,*,#31964,.F.);
#46096=ORIENTED_EDGE('',*,*,#31965,.T.);
#46097=ORIENTED_EDGE('',*,*,#31966,.T.);
#46098=ORIENTED_EDGE('',*,*,#31967,.T.);
#46099=ORIENTED_EDGE('',*,*,#31968,.F.);
#46100=ORIENTED_EDGE('',*,*,#31967,.F.);
#46101=ORIENTED_EDGE('',*,*,#31969,.F.);
#46102=ORIENTED_EDGE('',*,*,#31970,.F.);
#46103=ORIENTED_EDGE('',*,*,#31969,.T.);
#46104=ORIENTED_EDGE('',*,*,#31966,.F.);
#46105=ORIENTED_EDGE('',*,*,#31971,.T.);
#46106=ORIENTED_EDGE('',*,*,#31972,.F.);
#46107=ORIENTED_EDGE('',*,*,#31971,.F.);
#46108=ORIENTED_EDGE('',*,*,#31965,.F.);
#46109=ORIENTED_EDGE('',*,*,#31973,.F.);
#46110=ORIENTED_EDGE('',*,*,#31974,.T.);
#46111=ORIENTED_EDGE('',*,*,#31975,.T.);
#46112=ORIENTED_EDGE('',*,*,#31976,.T.);
#46113=ORIENTED_EDGE('',*,*,#31977,.F.);
#46114=ORIENTED_EDGE('',*,*,#31976,.F.);
#46115=ORIENTED_EDGE('',*,*,#31978,.F.);
#46116=ORIENTED_EDGE('',*,*,#31979,.F.);
#46117=ORIENTED_EDGE('',*,*,#31978,.T.);
#46118=ORIENTED_EDGE('',*,*,#31975,.F.);
#46119=ORIENTED_EDGE('',*,*,#31980,.T.);
#46120=ORIENTED_EDGE('',*,*,#31981,.F.);
#46121=ORIENTED_EDGE('',*,*,#31980,.F.);
#46122=ORIENTED_EDGE('',*,*,#31974,.F.);
#46123=ORIENTED_EDGE('',*,*,#31982,.F.);
#46124=ORIENTED_EDGE('',*,*,#31983,.T.);
#46125=ORIENTED_EDGE('',*,*,#31984,.T.);
#46126=ORIENTED_EDGE('',*,*,#31985,.T.);
#46127=ORIENTED_EDGE('',*,*,#31986,.F.);
#46128=ORIENTED_EDGE('',*,*,#31985,.F.);
#46129=ORIENTED_EDGE('',*,*,#31987,.F.);
#46130=ORIENTED_EDGE('',*,*,#31988,.F.);
#46131=ORIENTED_EDGE('',*,*,#31987,.T.);
#46132=ORIENTED_EDGE('',*,*,#31984,.F.);
#46133=ORIENTED_EDGE('',*,*,#31989,.T.);
#46134=ORIENTED_EDGE('',*,*,#31990,.F.);
#46135=ORIENTED_EDGE('',*,*,#31989,.F.);
#46136=ORIENTED_EDGE('',*,*,#31983,.F.);
#46137=ORIENTED_EDGE('',*,*,#31991,.F.);
#46138=ORIENTED_EDGE('',*,*,#31992,.T.);
#46139=ORIENTED_EDGE('',*,*,#31993,.T.);
#46140=ORIENTED_EDGE('',*,*,#31994,.T.);
#46141=ORIENTED_EDGE('',*,*,#31995,.F.);
#46142=ORIENTED_EDGE('',*,*,#31994,.F.);
#46143=ORIENTED_EDGE('',*,*,#31996,.F.);
#46144=ORIENTED_EDGE('',*,*,#31997,.F.);
#46145=ORIENTED_EDGE('',*,*,#31996,.T.);
#46146=ORIENTED_EDGE('',*,*,#31993,.F.);
#46147=ORIENTED_EDGE('',*,*,#31998,.T.);
#46148=ORIENTED_EDGE('',*,*,#31999,.F.);
#46149=ORIENTED_EDGE('',*,*,#31998,.F.);
#46150=ORIENTED_EDGE('',*,*,#31992,.F.);
#46151=ORIENTED_EDGE('',*,*,#32000,.F.);
#46152=ORIENTED_EDGE('',*,*,#32001,.T.);
#46153=ORIENTED_EDGE('',*,*,#32002,.T.);
#46154=ORIENTED_EDGE('',*,*,#32003,.T.);
#46155=ORIENTED_EDGE('',*,*,#32004,.F.);
#46156=ORIENTED_EDGE('',*,*,#32003,.F.);
#46157=ORIENTED_EDGE('',*,*,#32005,.F.);
#46158=ORIENTED_EDGE('',*,*,#32006,.F.);
#46159=ORIENTED_EDGE('',*,*,#32005,.T.);
#46160=ORIENTED_EDGE('',*,*,#32002,.F.);
#46161=ORIENTED_EDGE('',*,*,#32007,.T.);
#46162=ORIENTED_EDGE('',*,*,#32008,.F.);
#46163=ORIENTED_EDGE('',*,*,#32007,.F.);
#46164=ORIENTED_EDGE('',*,*,#32001,.F.);
#46165=ORIENTED_EDGE('',*,*,#32009,.F.);
#46166=ORIENTED_EDGE('',*,*,#32010,.T.);
#46167=ORIENTED_EDGE('',*,*,#32011,.T.);
#46168=ORIENTED_EDGE('',*,*,#32012,.T.);
#46169=ORIENTED_EDGE('',*,*,#32013,.F.);
#46170=ORIENTED_EDGE('',*,*,#32012,.F.);
#46171=ORIENTED_EDGE('',*,*,#32014,.F.);
#46172=ORIENTED_EDGE('',*,*,#32015,.F.);
#46173=ORIENTED_EDGE('',*,*,#32014,.T.);
#46174=ORIENTED_EDGE('',*,*,#32011,.F.);
#46175=ORIENTED_EDGE('',*,*,#32016,.T.);
#46176=ORIENTED_EDGE('',*,*,#32017,.F.);
#46177=ORIENTED_EDGE('',*,*,#32016,.F.);
#46178=ORIENTED_EDGE('',*,*,#32010,.F.);
#46179=ORIENTED_EDGE('',*,*,#32018,.F.);
#46180=ORIENTED_EDGE('',*,*,#32019,.T.);
#46181=ORIENTED_EDGE('',*,*,#32020,.T.);
#46182=ORIENTED_EDGE('',*,*,#32021,.T.);
#46183=ORIENTED_EDGE('',*,*,#32022,.F.);
#46184=ORIENTED_EDGE('',*,*,#32021,.F.);
#46185=ORIENTED_EDGE('',*,*,#32023,.F.);
#46186=ORIENTED_EDGE('',*,*,#32024,.F.);
#46187=ORIENTED_EDGE('',*,*,#32023,.T.);
#46188=ORIENTED_EDGE('',*,*,#32020,.F.);
#46189=ORIENTED_EDGE('',*,*,#32025,.T.);
#46190=ORIENTED_EDGE('',*,*,#32026,.F.);
#46191=ORIENTED_EDGE('',*,*,#32025,.F.);
#46192=ORIENTED_EDGE('',*,*,#32019,.F.);
#46193=ORIENTED_EDGE('',*,*,#32027,.F.);
#46194=ORIENTED_EDGE('',*,*,#32028,.T.);
#46195=ORIENTED_EDGE('',*,*,#32029,.T.);
#46196=ORIENTED_EDGE('',*,*,#32030,.T.);
#46197=ORIENTED_EDGE('',*,*,#32031,.F.);
#46198=ORIENTED_EDGE('',*,*,#32030,.F.);
#46199=ORIENTED_EDGE('',*,*,#32032,.F.);
#46200=ORIENTED_EDGE('',*,*,#32033,.F.);
#46201=ORIENTED_EDGE('',*,*,#32032,.T.);
#46202=ORIENTED_EDGE('',*,*,#32029,.F.);
#46203=ORIENTED_EDGE('',*,*,#32034,.T.);
#46204=ORIENTED_EDGE('',*,*,#32035,.F.);
#46205=ORIENTED_EDGE('',*,*,#32034,.F.);
#46206=ORIENTED_EDGE('',*,*,#32028,.F.);
#46207=ORIENTED_EDGE('',*,*,#32036,.F.);
#46208=ORIENTED_EDGE('',*,*,#32037,.T.);
#46209=ORIENTED_EDGE('',*,*,#32038,.T.);
#46210=ORIENTED_EDGE('',*,*,#32039,.T.);
#46211=ORIENTED_EDGE('',*,*,#32040,.F.);
#46212=ORIENTED_EDGE('',*,*,#32039,.F.);
#46213=ORIENTED_EDGE('',*,*,#32041,.F.);
#46214=ORIENTED_EDGE('',*,*,#32042,.F.);
#46215=ORIENTED_EDGE('',*,*,#32041,.T.);
#46216=ORIENTED_EDGE('',*,*,#32038,.F.);
#46217=ORIENTED_EDGE('',*,*,#32043,.T.);
#46218=ORIENTED_EDGE('',*,*,#32044,.F.);
#46219=ORIENTED_EDGE('',*,*,#32043,.F.);
#46220=ORIENTED_EDGE('',*,*,#32037,.F.);
#46221=ORIENTED_EDGE('',*,*,#32045,.F.);
#46222=ORIENTED_EDGE('',*,*,#32046,.F.);
#46223=ORIENTED_EDGE('',*,*,#32047,.F.);
#46224=ORIENTED_EDGE('',*,*,#32048,.F.);
#46225=ORIENTED_EDGE('',*,*,#32049,.T.);
#46226=ORIENTED_EDGE('',*,*,#32050,.T.);
#46227=ORIENTED_EDGE('',*,*,#32046,.T.);
#46228=ORIENTED_EDGE('',*,*,#32051,.F.);
#46229=ORIENTED_EDGE('',*,*,#32047,.T.);
#46230=ORIENTED_EDGE('',*,*,#32050,.F.);
#46231=ORIENTED_EDGE('',*,*,#32052,.T.);
#46232=ORIENTED_EDGE('',*,*,#32053,.F.);
#46233=ORIENTED_EDGE('',*,*,#32052,.F.);
#46234=ORIENTED_EDGE('',*,*,#32049,.F.);
#46235=ORIENTED_EDGE('',*,*,#32054,.T.);
#46236=ORIENTED_EDGE('',*,*,#32055,.F.);
#46237=ORIENTED_EDGE('',*,*,#32054,.F.);
#46238=ORIENTED_EDGE('',*,*,#32056,.F.);
#46239=ORIENTED_EDGE('',*,*,#32057,.F.);
#46240=ORIENTED_EDGE('',*,*,#32058,.F.);
#46241=ORIENTED_EDGE('',*,*,#32059,.T.);
#46242=ORIENTED_EDGE('',*,*,#32060,.F.);
#46243=ORIENTED_EDGE('',*,*,#32059,.F.);
#46244=ORIENTED_EDGE('',*,*,#32061,.F.);
#46245=ORIENTED_EDGE('',*,*,#32062,.T.);
#46246=ORIENTED_EDGE('',*,*,#32063,.F.);
#46247=ORIENTED_EDGE('',*,*,#32062,.F.);
#46248=ORIENTED_EDGE('',*,*,#32064,.F.);
#46249=ORIENTED_EDGE('',*,*,#32065,.T.);
#46250=ORIENTED_EDGE('',*,*,#32066,.F.);
#46251=ORIENTED_EDGE('',*,*,#32065,.F.);
#46252=ORIENTED_EDGE('',*,*,#32067,.F.);
#46253=ORIENTED_EDGE('',*,*,#32068,.T.);
#46254=ORIENTED_EDGE('',*,*,#32069,.F.);
#46255=ORIENTED_EDGE('',*,*,#32068,.F.);
#46256=ORIENTED_EDGE('',*,*,#32070,.F.);
#46257=ORIENTED_EDGE('',*,*,#32071,.T.);
#46258=ORIENTED_EDGE('',*,*,#32072,.F.);
#46259=ORIENTED_EDGE('',*,*,#32071,.F.);
#46260=ORIENTED_EDGE('',*,*,#32073,.F.);
#46261=ORIENTED_EDGE('',*,*,#32057,.T.);
#46262=ORIENTED_EDGE('',*,*,#32064,.T.);
#46263=ORIENTED_EDGE('',*,*,#32061,.T.);
#46264=ORIENTED_EDGE('',*,*,#32058,.T.);
#46265=ORIENTED_EDGE('',*,*,#32073,.T.);
#46266=ORIENTED_EDGE('',*,*,#32070,.T.);
#46267=ORIENTED_EDGE('',*,*,#32067,.T.);
#46268=ORIENTED_EDGE('',*,*,#32055,.T.);
#46269=ORIENTED_EDGE('',*,*,#32074,.F.);
#46270=ORIENTED_EDGE('',*,*,#31718,.F.);
#46271=ORIENTED_EDGE('',*,*,#31615,.F.);
#46272=ORIENTED_EDGE('',*,*,#31719,.F.);
#46273=ORIENTED_EDGE('',*,*,#32075,.T.);
#46274=ORIENTED_EDGE('',*,*,#32074,.T.);
#46275=ORIENTED_EDGE('',*,*,#32075,.F.);
#46276=ORIENTED_EDGE('',*,*,#31728,.T.);
#46277=ORIENTED_EDGE('',*,*,#32076,.F.);
#46278=ORIENTED_EDGE('',*,*,#31743,.T.);
#46279=ORIENTED_EDGE('',*,*,#31745,.T.);
#46280=ORIENTED_EDGE('',*,*,#31737,.T.);
#46281=ORIENTED_EDGE('',*,*,#32077,.F.);
#46282=ORIENTED_EDGE('',*,*,#31752,.T.);
#46283=ORIENTED_EDGE('',*,*,#31754,.T.);
#46284=ORIENTED_EDGE('',*,*,#31746,.T.);
#46285=ORIENTED_EDGE('',*,*,#32078,.F.);
#46286=ORIENTED_EDGE('',*,*,#31761,.T.);
#46287=ORIENTED_EDGE('',*,*,#31763,.T.);
#46288=ORIENTED_EDGE('',*,*,#31755,.T.);
#46289=ORIENTED_EDGE('',*,*,#32079,.F.);
#46290=ORIENTED_EDGE('',*,*,#31770,.T.);
#46291=ORIENTED_EDGE('',*,*,#31772,.T.);
#46292=ORIENTED_EDGE('',*,*,#31764,.T.);
#46293=ORIENTED_EDGE('',*,*,#32080,.F.);
#46294=ORIENTED_EDGE('',*,*,#31779,.T.);
#46295=ORIENTED_EDGE('',*,*,#31781,.T.);
#46296=ORIENTED_EDGE('',*,*,#31773,.T.);
#46297=ORIENTED_EDGE('',*,*,#32081,.F.);
#46298=ORIENTED_EDGE('',*,*,#31788,.T.);
#46299=ORIENTED_EDGE('',*,*,#31790,.T.);
#46300=ORIENTED_EDGE('',*,*,#31782,.T.);
#46301=ORIENTED_EDGE('',*,*,#32082,.F.);
#46302=ORIENTED_EDGE('',*,*,#31797,.T.);
#46303=ORIENTED_EDGE('',*,*,#31799,.T.);
#46304=ORIENTED_EDGE('',*,*,#31791,.T.);
#46305=ORIENTED_EDGE('',*,*,#32083,.F.);
#46306=ORIENTED_EDGE('',*,*,#31806,.T.);
#46307=ORIENTED_EDGE('',*,*,#31808,.T.);
#46308=ORIENTED_EDGE('',*,*,#31800,.T.);
#46309=ORIENTED_EDGE('',*,*,#32084,.F.);
#46310=ORIENTED_EDGE('',*,*,#31815,.T.);
#46311=ORIENTED_EDGE('',*,*,#31817,.T.);
#46312=ORIENTED_EDGE('',*,*,#31809,.T.);
#46313=ORIENTED_EDGE('',*,*,#32085,.F.);
#46314=ORIENTED_EDGE('',*,*,#31824,.T.);
#46315=ORIENTED_EDGE('',*,*,#31826,.T.);
#46316=ORIENTED_EDGE('',*,*,#31818,.T.);
#46317=ORIENTED_EDGE('',*,*,#32086,.F.);
#46318=ORIENTED_EDGE('',*,*,#31833,.T.);
#46319=ORIENTED_EDGE('',*,*,#31835,.T.);
#46320=ORIENTED_EDGE('',*,*,#31827,.T.);
#46321=ORIENTED_EDGE('',*,*,#32087,.F.);
#46322=ORIENTED_EDGE('',*,*,#31842,.T.);
#46323=ORIENTED_EDGE('',*,*,#31844,.T.);
#46324=ORIENTED_EDGE('',*,*,#31836,.T.);
#46325=ORIENTED_EDGE('',*,*,#32088,.F.);
#46326=ORIENTED_EDGE('',*,*,#31851,.T.);
#46327=ORIENTED_EDGE('',*,*,#31853,.T.);
#46328=ORIENTED_EDGE('',*,*,#31845,.T.);
#46329=ORIENTED_EDGE('',*,*,#32089,.F.);
#46330=ORIENTED_EDGE('',*,*,#31860,.T.);
#46331=ORIENTED_EDGE('',*,*,#31862,.T.);
#46332=ORIENTED_EDGE('',*,*,#31854,.T.);
#46333=ORIENTED_EDGE('',*,*,#32090,.F.);
#46334=ORIENTED_EDGE('',*,*,#31869,.T.);
#46335=ORIENTED_EDGE('',*,*,#31871,.T.);
#46336=ORIENTED_EDGE('',*,*,#31863,.T.);
#46337=ORIENTED_EDGE('',*,*,#32091,.F.);
#46338=ORIENTED_EDGE('',*,*,#31878,.T.);
#46339=ORIENTED_EDGE('',*,*,#31880,.T.);
#46340=ORIENTED_EDGE('',*,*,#31872,.T.);
#46341=ORIENTED_EDGE('',*,*,#32092,.F.);
#46342=ORIENTED_EDGE('',*,*,#31888,.T.);
#46343=ORIENTED_EDGE('',*,*,#31890,.T.);
#46344=ORIENTED_EDGE('',*,*,#32093,.T.);
#46345=ORIENTED_EDGE('',*,*,#31727,.T.);
#46346=ORIENTED_EDGE('',*,*,#32093,.F.);
#46347=ORIENTED_EDGE('',*,*,#31891,.T.);
#46348=ORIENTED_EDGE('',*,*,#31881,.T.);
#46349=ORIENTED_EDGE('',*,*,#32094,.F.);
#46350=ORIENTED_EDGE('',*,*,#31898,.T.);
#46351=ORIENTED_EDGE('',*,*,#31900,.T.);
#46352=ORIENTED_EDGE('',*,*,#31892,.T.);
#46353=ORIENTED_EDGE('',*,*,#32095,.F.);
#46354=ORIENTED_EDGE('',*,*,#31907,.T.);
#46355=ORIENTED_EDGE('',*,*,#31909,.T.);
#46356=ORIENTED_EDGE('',*,*,#31901,.T.);
#46357=ORIENTED_EDGE('',*,*,#32096,.F.);
#46358=ORIENTED_EDGE('',*,*,#31916,.T.);
#46359=ORIENTED_EDGE('',*,*,#31918,.T.);
#46360=ORIENTED_EDGE('',*,*,#31910,.T.);
#46361=ORIENTED_EDGE('',*,*,#32097,.F.);
#46362=ORIENTED_EDGE('',*,*,#31925,.T.);
#46363=ORIENTED_EDGE('',*,*,#31927,.T.);
#46364=ORIENTED_EDGE('',*,*,#31919,.T.);
#46365=ORIENTED_EDGE('',*,*,#32098,.F.);
#46366=ORIENTED_EDGE('',*,*,#31934,.T.);
#46367=ORIENTED_EDGE('',*,*,#31936,.T.);
#46368=ORIENTED_EDGE('',*,*,#31928,.T.);
#46369=ORIENTED_EDGE('',*,*,#32099,.F.);
#46370=ORIENTED_EDGE('',*,*,#31943,.T.);
#46371=ORIENTED_EDGE('',*,*,#31945,.T.);
#46372=ORIENTED_EDGE('',*,*,#31937,.T.);
#46373=ORIENTED_EDGE('',*,*,#32100,.F.);
#46374=ORIENTED_EDGE('',*,*,#31952,.T.);
#46375=ORIENTED_EDGE('',*,*,#31954,.T.);
#46376=ORIENTED_EDGE('',*,*,#31946,.T.);
#46377=ORIENTED_EDGE('',*,*,#32101,.F.);
#46378=ORIENTED_EDGE('',*,*,#31961,.T.);
#46379=ORIENTED_EDGE('',*,*,#31963,.T.);
#46380=ORIENTED_EDGE('',*,*,#31955,.T.);
#46381=ORIENTED_EDGE('',*,*,#32102,.F.);
#46382=ORIENTED_EDGE('',*,*,#31970,.T.);
#46383=ORIENTED_EDGE('',*,*,#31972,.T.);
#46384=ORIENTED_EDGE('',*,*,#31964,.T.);
#46385=ORIENTED_EDGE('',*,*,#32103,.F.);
#46386=ORIENTED_EDGE('',*,*,#31979,.T.);
#46387=ORIENTED_EDGE('',*,*,#31981,.T.);
#46388=ORIENTED_EDGE('',*,*,#31973,.T.);
#46389=ORIENTED_EDGE('',*,*,#32104,.F.);
#46390=ORIENTED_EDGE('',*,*,#31988,.T.);
#46391=ORIENTED_EDGE('',*,*,#31990,.T.);
#46392=ORIENTED_EDGE('',*,*,#31982,.T.);
#46393=ORIENTED_EDGE('',*,*,#32105,.F.);
#46394=ORIENTED_EDGE('',*,*,#31997,.T.);
#46395=ORIENTED_EDGE('',*,*,#31999,.T.);
#46396=ORIENTED_EDGE('',*,*,#31991,.T.);
#46397=ORIENTED_EDGE('',*,*,#32106,.F.);
#46398=ORIENTED_EDGE('',*,*,#32006,.T.);
#46399=ORIENTED_EDGE('',*,*,#32008,.T.);
#46400=ORIENTED_EDGE('',*,*,#32000,.T.);
#46401=ORIENTED_EDGE('',*,*,#32107,.F.);
#46402=ORIENTED_EDGE('',*,*,#32015,.T.);
#46403=ORIENTED_EDGE('',*,*,#32017,.T.);
#46404=ORIENTED_EDGE('',*,*,#32009,.T.);
#46405=ORIENTED_EDGE('',*,*,#32108,.F.);
#46406=ORIENTED_EDGE('',*,*,#32024,.T.);
#46407=ORIENTED_EDGE('',*,*,#32026,.T.);
#46408=ORIENTED_EDGE('',*,*,#32018,.T.);
#46409=ORIENTED_EDGE('',*,*,#32109,.F.);
#46410=ORIENTED_EDGE('',*,*,#32033,.T.);
#46411=ORIENTED_EDGE('',*,*,#32035,.T.);
#46412=ORIENTED_EDGE('',*,*,#32027,.T.);
#46413=ORIENTED_EDGE('',*,*,#32110,.F.);
#46414=ORIENTED_EDGE('',*,*,#32042,.T.);
#46415=ORIENTED_EDGE('',*,*,#32044,.T.);
#46416=ORIENTED_EDGE('',*,*,#32036,.T.);
#46417=ORIENTED_EDGE('',*,*,#32111,.F.);
#46418=ORIENTED_EDGE('',*,*,#32051,.T.);
#46419=ORIENTED_EDGE('',*,*,#32053,.T.);
#46420=ORIENTED_EDGE('',*,*,#32048,.T.);
#46421=ORIENTED_EDGE('',*,*,#32112,.F.);
#46422=ORIENTED_EDGE('',*,*,#31734,.T.);
#46423=ORIENTED_EDGE('',*,*,#31736,.T.);
#46424=ORIENTED_EDGE('',*,*,#32113,.F.);
#46425=ORIENTED_EDGE('',*,*,#32114,.T.);
#46426=ORIENTED_EDGE('',*,*,#31887,.T.);
#46427=ORIENTED_EDGE('',*,*,#32092,.T.);
#46428=ORIENTED_EDGE('',*,*,#31876,.T.);
#46429=ORIENTED_EDGE('',*,*,#32091,.T.);
#46430=ORIENTED_EDGE('',*,*,#31867,.T.);
#46431=ORIENTED_EDGE('',*,*,#32090,.T.);
#46432=ORIENTED_EDGE('',*,*,#31858,.T.);
#46433=ORIENTED_EDGE('',*,*,#32089,.T.);
#46434=ORIENTED_EDGE('',*,*,#31849,.T.);
#46435=ORIENTED_EDGE('',*,*,#32088,.T.);
#46436=ORIENTED_EDGE('',*,*,#31840,.T.);
#46437=ORIENTED_EDGE('',*,*,#32087,.T.);
#46438=ORIENTED_EDGE('',*,*,#31831,.T.);
#46439=ORIENTED_EDGE('',*,*,#32086,.T.);
#46440=ORIENTED_EDGE('',*,*,#31822,.T.);
#46441=ORIENTED_EDGE('',*,*,#32085,.T.);
#46442=ORIENTED_EDGE('',*,*,#31813,.T.);
#46443=ORIENTED_EDGE('',*,*,#32084,.T.);
#46444=ORIENTED_EDGE('',*,*,#31804,.T.);
#46445=ORIENTED_EDGE('',*,*,#32083,.T.);
#46446=ORIENTED_EDGE('',*,*,#31795,.T.);
#46447=ORIENTED_EDGE('',*,*,#32082,.T.);
#46448=ORIENTED_EDGE('',*,*,#31786,.T.);
#46449=ORIENTED_EDGE('',*,*,#32081,.T.);
#46450=ORIENTED_EDGE('',*,*,#31777,.T.);
#46451=ORIENTED_EDGE('',*,*,#32080,.T.);
#46452=ORIENTED_EDGE('',*,*,#31768,.T.);
#46453=ORIENTED_EDGE('',*,*,#32079,.T.);
#46454=ORIENTED_EDGE('',*,*,#31759,.T.);
#46455=ORIENTED_EDGE('',*,*,#32078,.T.);
#46456=ORIENTED_EDGE('',*,*,#31750,.T.);
#46457=ORIENTED_EDGE('',*,*,#32077,.T.);
#46458=ORIENTED_EDGE('',*,*,#31741,.T.);
#46459=ORIENTED_EDGE('',*,*,#32076,.T.);
#46460=ORIENTED_EDGE('',*,*,#31732,.T.);
#46461=ORIENTED_EDGE('',*,*,#32112,.T.);
#46462=ORIENTED_EDGE('',*,*,#32045,.T.);
#46463=ORIENTED_EDGE('',*,*,#32111,.T.);
#46464=ORIENTED_EDGE('',*,*,#32040,.T.);
#46465=ORIENTED_EDGE('',*,*,#32110,.T.);
#46466=ORIENTED_EDGE('',*,*,#32031,.T.);
#46467=ORIENTED_EDGE('',*,*,#32109,.T.);
#46468=ORIENTED_EDGE('',*,*,#32022,.T.);
#46469=ORIENTED_EDGE('',*,*,#32108,.T.);
#46470=ORIENTED_EDGE('',*,*,#32013,.T.);
#46471=ORIENTED_EDGE('',*,*,#32107,.T.);
#46472=ORIENTED_EDGE('',*,*,#32004,.T.);
#46473=ORIENTED_EDGE('',*,*,#32106,.T.);
#46474=ORIENTED_EDGE('',*,*,#31995,.T.);
#46475=ORIENTED_EDGE('',*,*,#32105,.T.);
#46476=ORIENTED_EDGE('',*,*,#31986,.T.);
#46477=ORIENTED_EDGE('',*,*,#32104,.T.);
#46478=ORIENTED_EDGE('',*,*,#31977,.T.);
#46479=ORIENTED_EDGE('',*,*,#32103,.T.);
#46480=ORIENTED_EDGE('',*,*,#31968,.T.);
#46481=ORIENTED_EDGE('',*,*,#32102,.T.);
#46482=ORIENTED_EDGE('',*,*,#31959,.T.);
#46483=ORIENTED_EDGE('',*,*,#32101,.T.);
#46484=ORIENTED_EDGE('',*,*,#31950,.T.);
#46485=ORIENTED_EDGE('',*,*,#32100,.T.);
#46486=ORIENTED_EDGE('',*,*,#31941,.T.);
#46487=ORIENTED_EDGE('',*,*,#32099,.T.);
#46488=ORIENTED_EDGE('',*,*,#31932,.T.);
#46489=ORIENTED_EDGE('',*,*,#32098,.T.);
#46490=ORIENTED_EDGE('',*,*,#31923,.T.);
#46491=ORIENTED_EDGE('',*,*,#32097,.T.);
#46492=ORIENTED_EDGE('',*,*,#31914,.T.);
#46493=ORIENTED_EDGE('',*,*,#32096,.T.);
#46494=ORIENTED_EDGE('',*,*,#31905,.T.);
#46495=ORIENTED_EDGE('',*,*,#32095,.T.);
#46496=ORIENTED_EDGE('',*,*,#31896,.T.);
#46497=ORIENTED_EDGE('',*,*,#32094,.T.);
#46498=ORIENTED_EDGE('',*,*,#31885,.T.);
#46499=ORIENTED_EDGE('',*,*,#32114,.F.);
#46500=ORIENTED_EDGE('',*,*,#32113,.T.);
#46501=ORIENTED_EDGE('',*,*,#32066,.T.);
#46502=ORIENTED_EDGE('',*,*,#32069,.T.);
#46503=ORIENTED_EDGE('',*,*,#32072,.T.);
#46504=ORIENTED_EDGE('',*,*,#32056,.T.);
#46505=ORIENTED_EDGE('',*,*,#32060,.T.);
#46506=ORIENTED_EDGE('',*,*,#32063,.T.);
#48306=CONICAL_SURFACE('',#54760,2.,1.02790944633836);
#48307=CONICAL_SURFACE('',#54771,4.5,0.785398163397448);
#48308=CONICAL_SURFACE('',#54809,7.5,0.785398163397449);
#50501=ADVANCED_FACE('',(#15414),#1157,.T.);
#50502=ADVANCED_FACE('',(#15415),#1158,.T.);
#50503=ADVANCED_FACE('',(#15416),#1159,.T.);
#50504=ADVANCED_FACE('',(#15417),#1160,.T.);
#50505=ADVANCED_FACE('',(#15418),#1161,.T.);
#50506=ADVANCED_FACE('',(#15419),#1162,.T.);
#50507=ADVANCED_FACE('',(#15420),#1163,.T.);
#50508=ADVANCED_FACE('',(#15421),#1164,.T.);
#50509=ADVANCED_FACE('',(#15422),#1165,.T.);
#50510=ADVANCED_FACE('',(#15423),#1166,.T.);
#50511=ADVANCED_FACE('',(#15424),#1167,.T.);
#50512=ADVANCED_FACE('',(#15425),#1168,.T.);
#50513=ADVANCED_FACE('',(#15426),#1169,.T.);
#50514=ADVANCED_FACE('',(#15427),#1170,.T.);
#50515=ADVANCED_FACE('',(#15428),#1171,.T.);
#50516=ADVANCED_FACE('',(#15429),#1172,.T.);
#50517=ADVANCED_FACE('',(#15430),#1173,.T.);
#50518=ADVANCED_FACE('',(#15431),#1174,.T.);
#50519=ADVANCED_FACE('',(#15432),#1175,.T.);
#50520=ADVANCED_FACE('',(#15433),#1176,.T.);
#50521=ADVANCED_FACE('',(#15434),#1177,.T.);
#50522=ADVANCED_FACE('',(#15435),#1178,.T.);
#50523=ADVANCED_FACE('',(#15436),#1179,.T.);
#50524=ADVANCED_FACE('',(#15437),#1180,.T.);
#50525=ADVANCED_FACE('',(#15438),#1181,.T.);
#50526=ADVANCED_FACE('',(#15439),#1182,.T.);
#50527=ADVANCED_FACE('',(#15440),#1183,.T.);
#50528=ADVANCED_FACE('',(#15441),#1184,.T.);
#50529=ADVANCED_FACE('',(#15442),#1185,.T.);
#50530=ADVANCED_FACE('',(#15443),#1186,.T.);
#50531=ADVANCED_FACE('',(#15444),#1187,.T.);
#50532=ADVANCED_FACE('',(#15445),#1188,.T.);
#50533=ADVANCED_FACE('',(#15446),#12903,.F.);
#50534=ADVANCED_FACE('',(#15447),#885,.F.);
#50535=ADVANCED_FACE('',(#15448),#12904,.T.);
#50536=ADVANCED_FACE('',(#15449),#1189,.T.);
#50537=ADVANCED_FACE('',(#15450),#886,.F.);
#50538=ADVANCED_FACE('',(#15451),#955,.F.);
#50539=ADVANCED_FACE('',(#15452),#1190,.T.);
#50540=ADVANCED_FACE('',(#15453,#1030),#12905,.T.);
#50541=ADVANCED_FACE('',(#15454),#12906,.F.);
#50542=ADVANCED_FACE('',(#15455),#12907,.F.);
#50543=ADVANCED_FACE('',(#15456),#12908,.F.);
#50544=ADVANCED_FACE('',(#15457),#12909,.T.);
#50545=ADVANCED_FACE('',(#15458),#12910,.F.);
#50546=ADVANCED_FACE('',(#15459),#12911,.F.);
#50547=ADVANCED_FACE('',(#15460),#12912,.F.);
#50548=ADVANCED_FACE('',(#15461),#12913,.T.);
#50549=ADVANCED_FACE('',(#15462),#12914,.F.);
#50550=ADVANCED_FACE('',(#15463),#12915,.F.);
#50551=ADVANCED_FACE('',(#15464),#12916,.F.);
#50552=ADVANCED_FACE('',(#15465),#12917,.T.);
#50553=ADVANCED_FACE('',(#15466),#12918,.F.);
#50554=ADVANCED_FACE('',(#15467),#12919,.F.);
#50555=ADVANCED_FACE('',(#15468),#12920,.F.);
#50556=ADVANCED_FACE('',(#15469),#12921,.T.);
#50557=ADVANCED_FACE('',(#15470),#12922,.F.);
#50558=ADVANCED_FACE('',(#15471),#12923,.F.);
#50559=ADVANCED_FACE('',(#15472),#12924,.F.);
#50560=ADVANCED_FACE('',(#15473),#12925,.T.);
#50561=ADVANCED_FACE('',(#15474),#12926,.F.);
#50562=ADVANCED_FACE('',(#15475),#12927,.F.);
#50563=ADVANCED_FACE('',(#15476),#12928,.F.);
#50564=ADVANCED_FACE('',(#15477),#12929,.T.);
#50565=ADVANCED_FACE('',(#15478),#12930,.F.);
#50566=ADVANCED_FACE('',(#15479),#12931,.F.);
#50567=ADVANCED_FACE('',(#15480),#12932,.F.);
#50568=ADVANCED_FACE('',(#15481),#12933,.T.);
#50569=ADVANCED_FACE('',(#15482),#12934,.F.);
#50570=ADVANCED_FACE('',(#15483),#12935,.F.);
#50571=ADVANCED_FACE('',(#15484),#12936,.F.);
#50572=ADVANCED_FACE('',(#15485),#12937,.T.);
#50573=ADVANCED_FACE('',(#15486),#12938,.F.);
#50574=ADVANCED_FACE('',(#15487),#12939,.F.);
#50575=ADVANCED_FACE('',(#15488),#12940,.F.);
#50576=ADVANCED_FACE('',(#15489),#12941,.T.);
#50577=ADVANCED_FACE('',(#15490),#12942,.F.);
#50578=ADVANCED_FACE('',(#15491),#12943,.F.);
#50579=ADVANCED_FACE('',(#15492),#12944,.F.);
#50580=ADVANCED_FACE('',(#15493),#12945,.T.);
#50581=ADVANCED_FACE('',(#15494),#12946,.F.);
#50582=ADVANCED_FACE('',(#15495),#12947,.F.);
#50583=ADVANCED_FACE('',(#15496),#12948,.F.);
#50584=ADVANCED_FACE('',(#15497),#12949,.T.);
#50585=ADVANCED_FACE('',(#15498),#12950,.F.);
#50586=ADVANCED_FACE('',(#15499),#12951,.F.);
#50587=ADVANCED_FACE('',(#15500),#12952,.F.);
#50588=ADVANCED_FACE('',(#15501),#12953,.T.);
#50589=ADVANCED_FACE('',(#15502),#12954,.F.);
#50590=ADVANCED_FACE('',(#15503),#12955,.F.);
#50591=ADVANCED_FACE('',(#15504),#12956,.F.);
#50592=ADVANCED_FACE('',(#15505),#12957,.T.);
#50593=ADVANCED_FACE('',(#15506),#12958,.F.);
#50594=ADVANCED_FACE('',(#15507),#12959,.F.);
#50595=ADVANCED_FACE('',(#15508),#12960,.F.);
#50596=ADVANCED_FACE('',(#15509),#12961,.T.);
#50597=ADVANCED_FACE('',(#15510),#12962,.F.);
#50598=ADVANCED_FACE('',(#15511),#12963,.F.);
#50599=ADVANCED_FACE('',(#15512),#12964,.F.);
#50600=ADVANCED_FACE('',(#15513),#12965,.T.);
#50601=ADVANCED_FACE('',(#15514),#12966,.F.);
#50602=ADVANCED_FACE('',(#15515),#12967,.F.);
#50603=ADVANCED_FACE('',(#15516),#12968,.F.);
#50604=ADVANCED_FACE('',(#15517),#12969,.T.);
#50605=ADVANCED_FACE('',(#15518),#12970,.F.);
#50606=ADVANCED_FACE('',(#15519),#12971,.F.);
#50607=ADVANCED_FACE('',(#15520),#12972,.F.);
#50608=ADVANCED_FACE('',(#15521),#12973,.T.);
#50609=ADVANCED_FACE('',(#15522),#12974,.F.);
#50610=ADVANCED_FACE('',(#15523),#12975,.F.);
#50611=ADVANCED_FACE('',(#15524),#12976,.F.);
#50612=ADVANCED_FACE('',(#15525),#12977,.T.);
#50613=ADVANCED_FACE('',(#15526),#12978,.F.);
#50614=ADVANCED_FACE('',(#15527),#12979,.F.);
#50615=ADVANCED_FACE('',(#15528),#12980,.F.);
#50616=ADVANCED_FACE('',(#15529),#12981,.T.);
#50617=ADVANCED_FACE('',(#15530),#12982,.F.);
#50618=ADVANCED_FACE('',(#15531),#12983,.F.);
#50619=ADVANCED_FACE('',(#15532),#12984,.F.);
#50620=ADVANCED_FACE('',(#15533),#12985,.T.);
#50621=ADVANCED_FACE('',(#15534),#12986,.F.);
#50622=ADVANCED_FACE('',(#15535),#12987,.F.);
#50623=ADVANCED_FACE('',(#15536),#12988,.F.);
#50624=ADVANCED_FACE('',(#15537),#12989,.T.);
#50625=ADVANCED_FACE('',(#15538),#12990,.F.);
#50626=ADVANCED_FACE('',(#15539),#12991,.F.);
#50627=ADVANCED_FACE('',(#15540),#12992,.F.);
#50628=ADVANCED_FACE('',(#15541),#12993,.T.);
#50629=ADVANCED_FACE('',(#15542),#12994,.F.);
#50630=ADVANCED_FACE('',(#15543),#12995,.F.);
#50631=ADVANCED_FACE('',(#15544),#12996,.F.);
#50632=ADVANCED_FACE('',(#15545),#12997,.T.);
#50633=ADVANCED_FACE('',(#15546),#12998,.F.);
#50634=ADVANCED_FACE('',(#15547),#12999,.F.);
#50635=ADVANCED_FACE('',(#15548),#13000,.F.);
#50636=ADVANCED_FACE('',(#15549),#13001,.T.);
#50637=ADVANCED_FACE('',(#15550),#13002,.F.);
#50638=ADVANCED_FACE('',(#15551),#13003,.F.);
#50639=ADVANCED_FACE('',(#15552),#13004,.F.);
#50640=ADVANCED_FACE('',(#15553),#13005,.T.);
#50641=ADVANCED_FACE('',(#15554),#13006,.F.);
#50642=ADVANCED_FACE('',(#15555),#13007,.F.);
#50643=ADVANCED_FACE('',(#15556),#13008,.F.);
#50644=ADVANCED_FACE('',(#15557),#13009,.T.);
#50645=ADVANCED_FACE('',(#15558),#13010,.F.);
#50646=ADVANCED_FACE('',(#15559),#13011,.F.);
#50647=ADVANCED_FACE('',(#15560),#13012,.F.);
#50648=ADVANCED_FACE('',(#15561),#13013,.T.);
#50649=ADVANCED_FACE('',(#15562),#13014,.F.);
#50650=ADVANCED_FACE('',(#15563),#13015,.F.);
#50651=ADVANCED_FACE('',(#15564),#13016,.F.);
#50652=ADVANCED_FACE('',(#15565),#13017,.T.);
#50653=ADVANCED_FACE('',(#15566),#13018,.F.);
#50654=ADVANCED_FACE('',(#15567),#13019,.F.);
#50655=ADVANCED_FACE('',(#15568),#13020,.F.);
#50656=ADVANCED_FACE('',(#15569),#13021,.T.);
#50657=ADVANCED_FACE('',(#15570),#13022,.F.);
#50658=ADVANCED_FACE('',(#15571),#13023,.F.);
#50659=ADVANCED_FACE('',(#15572),#13024,.F.);
#50660=ADVANCED_FACE('',(#15573),#13025,.T.);
#50661=ADVANCED_FACE('',(#15574),#13026,.F.);
#50662=ADVANCED_FACE('',(#15575),#13027,.F.);
#50663=ADVANCED_FACE('',(#15576),#13028,.F.);
#50664=ADVANCED_FACE('',(#15577),#13029,.T.);
#50665=ADVANCED_FACE('',(#15578),#13030,.F.);
#50666=ADVANCED_FACE('',(#15579),#13031,.F.);
#50667=ADVANCED_FACE('',(#15580),#13032,.F.);
#50668=ADVANCED_FACE('',(#15581),#13033,.T.);
#50669=ADVANCED_FACE('',(#15582),#13034,.F.);
#50670=ADVANCED_FACE('',(#15583),#13035,.F.);
#50671=ADVANCED_FACE('',(#15584),#13036,.F.);
#50672=ADVANCED_FACE('',(#15585),#13037,.T.);
#50673=ADVANCED_FACE('',(#15586),#13038,.F.);
#50674=ADVANCED_FACE('',(#15587),#13039,.F.);
#50675=ADVANCED_FACE('',(#15588),#13040,.F.);
#50676=ADVANCED_FACE('',(#15589),#13041,.T.);
#50677=ADVANCED_FACE('',(#15590),#13042,.F.);
#50678=ADVANCED_FACE('',(#15591),#13043,.F.);
#50679=ADVANCED_FACE('',(#15592),#13044,.F.);
#50680=ADVANCED_FACE('',(#15593),#13045,.T.);
#50681=ADVANCED_FACE('',(#15594),#13046,.F.);
#50682=ADVANCED_FACE('',(#15595),#13047,.F.);
#50683=ADVANCED_FACE('',(#15596),#13048,.F.);
#50684=ADVANCED_FACE('',(#15597),#13049,.T.);
#50685=ADVANCED_FACE('',(#15598),#48306,.F.);
#50686=ADVANCED_FACE('',(#15599),#13050,.F.);
#50687=ADVANCED_FACE('',(#15600),#13051,.F.);
#50688=ADVANCED_FACE('',(#15601),#13052,.F.);
#50689=ADVANCED_FACE('',(#15602),#13053,.F.);
#50690=ADVANCED_FACE('',(#15603),#13054,.F.);
#50691=ADVANCED_FACE('',(#15604),#13055,.F.);
#50692=ADVANCED_FACE('',(#15605,#1031),#13056,.T.);
#50693=ADVANCED_FACE('',(#15606),#13057,.T.);
#50694=ADVANCED_FACE('',(#15607),#48307,.T.);
#50695=ADVANCED_FACE('',(#15608),#1191,.T.);
#50696=ADVANCED_FACE('',(#15609),#48308,.T.);
#50697=ADVANCED_FACE('',(#15610,#1032),#13058,.T.);
#51023=CLOSED_SHELL('',(#50501,#50502,#50503,#50504,#50505,#50506,#50507,
#50508,#50509,#50510,#50511,#50512,#50513,#50514,#50515,#50516,#50517,#50518,
#50519,#50520,#50521,#50522,#50523,#50524,#50525,#50526,#50527,#50528,#50529,
#50530,#50531,#50532,#50533,#50534,#50535,#50536,#50537,#50538,#50539,#50540,
#50541,#50542,#50543,#50544,#50545,#50546,#50547,#50548,#50549,#50550,#50551,
#50552,#50553,#50554,#50555,#50556,#50557,#50558,#50559,#50560,#50561,#50562,
#50563,#50564,#50565,#50566,#50567,#50568,#50569,#50570,#50571,#50572,#50573,
#50574,#50575,#50576,#50577,#50578,#50579,#50580,#50581,#50582,#50583,#50584,
#50585,#50586,#50587,#50588,#50589,#50590,#50591,#50592,#50593,#50594,#50595,
#50596,#50597,#50598,#50599,#50600,#50601,#50602,#50603,#50604,#50605,#50606,
#50607,#50608,#50609,#50610,#50611,#50612,#50613,#50614,#50615,#50616,#50617,
#50618,#50619,#50620,#50621,#50622,#50623,#50624,#50625,#50626,#50627,#50628,
#50629,#50630,#50631,#50632,#50633,#50634,#50635,#50636,#50637,#50638,#50639,
#50640,#50641,#50642,#50643,#50644,#50645,#50646,#50647,#50648,#50649,#50650,
#50651,#50652,#50653,#50654,#50655,#50656,#50657,#50658,#50659,#50660,#50661,
#50662,#50663,#50664,#50665,#50666,#50667,#50668,#50669,#50670,#50671,#50672,
#50673,#50674,#50675,#50676,#50677,#50678,#50679,#50680,#50681,#50682,#50683,
#50684,#50685,#50686,#50687,#50688,#50689,#50690,#50691,#50692,#50693,#50694,
#50695,#50696,#50697));
#54491=AXIS2_PLACEMENT_3D('',#84081,#65795,#65796);
#54492=AXIS2_PLACEMENT_3D('',#84082,#65797,#65798);
#54493=AXIS2_PLACEMENT_3D('',#84098,#65800,#65801);
#54494=AXIS2_PLACEMENT_3D('',#84109,#65802,#65803);
#54495=AXIS2_PLACEMENT_3D('',#84157,#65805,#65806);
#54496=AXIS2_PLACEMENT_3D('',#84205,#65808,#65809);
#54497=AXIS2_PLACEMENT_3D('',#84259,#65811,#65812);
#54498=AXIS2_PLACEMENT_3D('',#84307,#65814,#65815);
#54499=AXIS2_PLACEMENT_3D('',#84355,#65817,#65818);
#54500=AXIS2_PLACEMENT_3D('',#84409,#65820,#65821);
#54501=AXIS2_PLACEMENT_3D('',#84457,#65823,#65824);
#54502=AXIS2_PLACEMENT_3D('',#84505,#65826,#65827);
#54503=AXIS2_PLACEMENT_3D('',#84559,#65829,#65830);
#54504=AXIS2_PLACEMENT_3D('',#84607,#65832,#65833);
#54505=AXIS2_PLACEMENT_3D('',#84655,#65835,#65836);
#54506=AXIS2_PLACEMENT_3D('',#84709,#65838,#65839);
#54507=AXIS2_PLACEMENT_3D('',#84757,#65841,#65842);
#54508=AXIS2_PLACEMENT_3D('',#84805,#65844,#65845);
#54509=AXIS2_PLACEMENT_3D('',#84859,#65847,#65848);
#54510=AXIS2_PLACEMENT_3D('',#84868,#65850,#65851);
#54511=AXIS2_PLACEMENT_3D('',#84869,#65852,#65853);
#54512=AXIS2_PLACEMENT_3D('',#84885,#65855,#65856);
#54513=AXIS2_PLACEMENT_3D('',#84896,#65857,#65858);
#54514=AXIS2_PLACEMENT_3D('',#84921,#65860,#65861);
#54515=AXIS2_PLACEMENT_3D('',#84945,#65863,#65864);
#54516=AXIS2_PLACEMENT_3D('',#84970,#65866,#65867);
#54517=AXIS2_PLACEMENT_3D('',#84995,#65869,#65870);
#54518=AXIS2_PLACEMENT_3D('',#85019,#65872,#65873);
#54519=AXIS2_PLACEMENT_3D('',#85044,#65875,#65876);
#54520=AXIS2_PLACEMENT_3D('',#85069,#65878,#65879);
#54521=AXIS2_PLACEMENT_3D('',#85093,#65881,#65882);
#54522=AXIS2_PLACEMENT_3D('',#85118,#65884,#65885);
#54523=AXIS2_PLACEMENT_3D('',#85143,#65887,#65888);
#54524=AXIS2_PLACEMENT_3D('',#85167,#65890,#65891);
#54525=AXIS2_PLACEMENT_3D('',#85192,#65893,#65894);
#54526=AXIS2_PLACEMENT_3D('',#85217,#65896,#65897);
#54527=AXIS2_PLACEMENT_3D('',#85241,#65899,#65900);
#54528=AXIS2_PLACEMENT_3D('',#85350,#65901,#65902);
#54529=AXIS2_PLACEMENT_3D('',#85352,#65903,#65904);
#54530=AXIS2_PLACEMENT_3D('',#86016,#65905,#65906);
#54531=AXIS2_PLACEMENT_3D('',#86018,#65907,#65908);
#54532=AXIS2_PLACEMENT_3D('',#86019,#65909,#65910);
#54533=AXIS2_PLACEMENT_3D('',#86127,#65911,#65912);
#54534=AXIS2_PLACEMENT_3D('',#86128,#65913,#65914);
#54535=AXIS2_PLACEMENT_3D('',#86579,#65915,#65916);
#54536=AXIS2_PLACEMENT_3D('',#86581,#65917,#65918);
#54537=AXIS2_PLACEMENT_3D('',#86582,#65919,#65920);
#54538=AXIS2_PLACEMENT_3D('',#86583,#65921,#65922);
#54539=AXIS2_PLACEMENT_3D('',#86584,#65923,#65924);
#54540=AXIS2_PLACEMENT_3D('',#86585,#65925,#65926);
#54541=AXIS2_PLACEMENT_3D('',#86587,#65927,#65928);
#54542=AXIS2_PLACEMENT_3D('',#86588,#65929,#65930);
#54543=AXIS2_PLACEMENT_3D('',#86597,#65935,#65936);
#54544=AXIS2_PLACEMENT_3D('',#86599,#65937,#65938);
#54545=AXIS2_PLACEMENT_3D('',#86601,#65940,#65941);
#54546=AXIS2_PLACEMENT_3D('',#86605,#65944,#65945);
#54547=AXIS2_PLACEMENT_3D('',#86606,#65946,#65947);
#54548=AXIS2_PLACEMENT_3D('',#86607,#65948,#65949);
#54549=AXIS2_PLACEMENT_3D('',#86616,#65954,#65955);
#54550=AXIS2_PLACEMENT_3D('',#86618,#65956,#65957);
#54551=AXIS2_PLACEMENT_3D('',#86620,#65959,#65960);
#54552=AXIS2_PLACEMENT_3D('',#86624,#65963,#65964);
#54553=AXIS2_PLACEMENT_3D('',#86625,#65965,#65966);
#54554=AXIS2_PLACEMENT_3D('',#86626,#65967,#65968);
#54555=AXIS2_PLACEMENT_3D('',#86635,#65973,#65974);
#54556=AXIS2_PLACEMENT_3D('',#86637,#65975,#65976);
#54557=AXIS2_PLACEMENT_3D('',#86639,#65978,#65979);
#54558=AXIS2_PLACEMENT_3D('',#86643,#65982,#65983);
#54559=AXIS2_PLACEMENT_3D('',#86644,#65984,#65985);
#54560=AXIS2_PLACEMENT_3D('',#86645,#65986,#65987);
#54561=AXIS2_PLACEMENT_3D('',#86654,#65992,#65993);
#54562=AXIS2_PLACEMENT_3D('',#86656,#65994,#65995);
#54563=AXIS2_PLACEMENT_3D('',#86658,#65997,#65998);
#54564=AXIS2_PLACEMENT_3D('',#86662,#66001,#66002);
#54565=AXIS2_PLACEMENT_3D('',#86663,#66003,#66004);
#54566=AXIS2_PLACEMENT_3D('',#86664,#66005,#66006);
#54567=AXIS2_PLACEMENT_3D('',#86673,#66011,#66012);
#54568=AXIS2_PLACEMENT_3D('',#86675,#66013,#66014);
#54569=AXIS2_PLACEMENT_3D('',#86677,#66016,#66017);
#54570=AXIS2_PLACEMENT_3D('',#86681,#66020,#66021);
#54571=AXIS2_PLACEMENT_3D('',#86682,#66022,#66023);
#54572=AXIS2_PLACEMENT_3D('',#86683,#66024,#66025);
#54573=AXIS2_PLACEMENT_3D('',#86692,#66030,#66031);
#54574=AXIS2_PLACEMENT_3D('',#86694,#66032,#66033);
#54575=AXIS2_PLACEMENT_3D('',#86696,#66035,#66036);
#54576=AXIS2_PLACEMENT_3D('',#86700,#66039,#66040);
#54577=AXIS2_PLACEMENT_3D('',#86701,#66041,#66042);
#54578=AXIS2_PLACEMENT_3D('',#86702,#66043,#66044);
#54579=AXIS2_PLACEMENT_3D('',#86711,#66049,#66050);
#54580=AXIS2_PLACEMENT_3D('',#86713,#66051,#66052);
#54581=AXIS2_PLACEMENT_3D('',#86715,#66054,#66055);
#54582=AXIS2_PLACEMENT_3D('',#86719,#66058,#66059);
#54583=AXIS2_PLACEMENT_3D('',#86720,#66060,#66061);
#54584=AXIS2_PLACEMENT_3D('',#86721,#66062,#66063);
#54585=AXIS2_PLACEMENT_3D('',#86730,#66068,#66069);
#54586=AXIS2_PLACEMENT_3D('',#86732,#66070,#66071);
#54587=AXIS2_PLACEMENT_3D('',#86734,#66073,#66074);
#54588=AXIS2_PLACEMENT_3D('',#86738,#66077,#66078);
#54589=AXIS2_PLACEMENT_3D('',#86739,#66079,#66080);
#54590=AXIS2_PLACEMENT_3D('',#86740,#66081,#66082);
#54591=AXIS2_PLACEMENT_3D('',#86749,#66087,#66088);
#54592=AXIS2_PLACEMENT_3D('',#86751,#66089,#66090);
#54593=AXIS2_PLACEMENT_3D('',#86753,#66092,#66093);
#54594=AXIS2_PLACEMENT_3D('',#86757,#66096,#66097);
#54595=AXIS2_PLACEMENT_3D('',#86758,#66098,#66099);
#54596=AXIS2_PLACEMENT_3D('',#86759,#66100,#66101);
#54597=AXIS2_PLACEMENT_3D('',#86768,#66106,#66107);
#54598=AXIS2_PLACEMENT_3D('',#86770,#66108,#66109);
#54599=AXIS2_PLACEMENT_3D('',#86772,#66111,#66112);
#54600=AXIS2_PLACEMENT_3D('',#86776,#66115,#66116);
#54601=AXIS2_PLACEMENT_3D('',#86777,#66117,#66118);
#54602=AXIS2_PLACEMENT_3D('',#86778,#66119,#66120);
#54603=AXIS2_PLACEMENT_3D('',#86787,#66125,#66126);
#54604=AXIS2_PLACEMENT_3D('',#86789,#66127,#66128);
#54605=AXIS2_PLACEMENT_3D('',#86791,#66130,#66131);
#54606=AXIS2_PLACEMENT_3D('',#86795,#66134,#66135);
#54607=AXIS2_PLACEMENT_3D('',#86796,#66136,#66137);
#54608=AXIS2_PLACEMENT_3D('',#86797,#66138,#66139);
#54609=AXIS2_PLACEMENT_3D('',#86806,#66144,#66145);
#54610=AXIS2_PLACEMENT_3D('',#86808,#66146,#66147);
#54611=AXIS2_PLACEMENT_3D('',#86810,#66149,#66150);
#54612=AXIS2_PLACEMENT_3D('',#86814,#66153,#66154);
#54613=AXIS2_PLACEMENT_3D('',#86815,#66155,#66156);
#54614=AXIS2_PLACEMENT_3D('',#86816,#66157,#66158);
#54615=AXIS2_PLACEMENT_3D('',#86825,#66163,#66164);
#54616=AXIS2_PLACEMENT_3D('',#86827,#66165,#66166);
#54617=AXIS2_PLACEMENT_3D('',#86829,#66168,#66169);
#54618=AXIS2_PLACEMENT_3D('',#86833,#66172,#66173);
#54619=AXIS2_PLACEMENT_3D('',#86834,#66174,#66175);
#54620=AXIS2_PLACEMENT_3D('',#86835,#66176,#66177);
#54621=AXIS2_PLACEMENT_3D('',#86844,#66182,#66183);
#54622=AXIS2_PLACEMENT_3D('',#86846,#66184,#66185);
#54623=AXIS2_PLACEMENT_3D('',#86848,#66187,#66188);
#54624=AXIS2_PLACEMENT_3D('',#86852,#66191,#66192);
#54625=AXIS2_PLACEMENT_3D('',#86853,#66193,#66194);
#54626=AXIS2_PLACEMENT_3D('',#86854,#66195,#66196);
#54627=AXIS2_PLACEMENT_3D('',#86863,#66201,#66202);
#54628=AXIS2_PLACEMENT_3D('',#86865,#66203,#66204);
#54629=AXIS2_PLACEMENT_3D('',#86867,#66206,#66207);
#54630=AXIS2_PLACEMENT_3D('',#86871,#66210,#66211);
#54631=AXIS2_PLACEMENT_3D('',#86872,#66212,#66213);
#54632=AXIS2_PLACEMENT_3D('',#86873,#66214,#66215);
#54633=AXIS2_PLACEMENT_3D('',#86882,#66220,#66221);
#54634=AXIS2_PLACEMENT_3D('',#86884,#66222,#66223);
#54635=AXIS2_PLACEMENT_3D('',#86886,#66225,#66226);
#54636=AXIS2_PLACEMENT_3D('',#86890,#66229,#66230);
#54637=AXIS2_PLACEMENT_3D('',#86891,#66231,#66232);
#54638=AXIS2_PLACEMENT_3D('',#86892,#66233,#66234);
#54639=AXIS2_PLACEMENT_3D('',#86901,#66239,#66240);
#54640=AXIS2_PLACEMENT_3D('',#86903,#66241,#66242);
#54641=AXIS2_PLACEMENT_3D('',#86905,#66244,#66245);
#54642=AXIS2_PLACEMENT_3D('',#86909,#66248,#66249);
#54643=AXIS2_PLACEMENT_3D('',#86910,#66250,#66251);
#54644=AXIS2_PLACEMENT_3D('',#86911,#66252,#66253);
#54645=AXIS2_PLACEMENT_3D('',#86920,#66258,#66259);
#54646=AXIS2_PLACEMENT_3D('',#86922,#66260,#66261);
#54647=AXIS2_PLACEMENT_3D('',#86925,#66263,#66264);
#54648=AXIS2_PLACEMENT_3D('',#86926,#66265,#66266);
#54649=AXIS2_PLACEMENT_3D('',#86930,#66269,#66270);
#54650=AXIS2_PLACEMENT_3D('',#86932,#66271,#66272);
#54651=AXIS2_PLACEMENT_3D('',#86933,#66273,#66274);
#54652=AXIS2_PLACEMENT_3D('',#86934,#66275,#66276);
#54653=AXIS2_PLACEMENT_3D('',#86943,#66281,#66282);
#54654=AXIS2_PLACEMENT_3D('',#86945,#66283,#66284);
#54655=AXIS2_PLACEMENT_3D('',#86947,#66286,#66287);
#54656=AXIS2_PLACEMENT_3D('',#86951,#66290,#66291);
#54657=AXIS2_PLACEMENT_3D('',#86952,#66292,#66293);
#54658=AXIS2_PLACEMENT_3D('',#86953,#66294,#66295);
#54659=AXIS2_PLACEMENT_3D('',#86962,#66300,#66301);
#54660=AXIS2_PLACEMENT_3D('',#86964,#66302,#66303);
#54661=AXIS2_PLACEMENT_3D('',#86966,#66305,#66306);
#54662=AXIS2_PLACEMENT_3D('',#86970,#66309,#66310);
#54663=AXIS2_PLACEMENT_3D('',#86971,#66311,#66312);
#54664=AXIS2_PLACEMENT_3D('',#86972,#66313,#66314);
#54665=AXIS2_PLACEMENT_3D('',#86981,#66319,#66320);
#54666=AXIS2_PLACEMENT_3D('',#86983,#66321,#66322);
#54667=AXIS2_PLACEMENT_3D('',#86985,#66324,#66325);
#54668=AXIS2_PLACEMENT_3D('',#86989,#66328,#66329);
#54669=AXIS2_PLACEMENT_3D('',#86990,#66330,#66331);
#54670=AXIS2_PLACEMENT_3D('',#86991,#66332,#66333);
#54671=AXIS2_PLACEMENT_3D('',#87000,#66338,#66339);
#54672=AXIS2_PLACEMENT_3D('',#87002,#66340,#66341);
#54673=AXIS2_PLACEMENT_3D('',#87004,#66343,#66344);
#54674=AXIS2_PLACEMENT_3D('',#87008,#66347,#66348);
#54675=AXIS2_PLACEMENT_3D('',#87009,#66349,#66350);
#54676=AXIS2_PLACEMENT_3D('',#87010,#66351,#66352);
#54677=AXIS2_PLACEMENT_3D('',#87019,#66357,#66358);
#54678=AXIS2_PLACEMENT_3D('',#87021,#66359,#66360);
#54679=AXIS2_PLACEMENT_3D('',#87023,#66362,#66363);
#54680=AXIS2_PLACEMENT_3D('',#87027,#66366,#66367);
#54681=AXIS2_PLACEMENT_3D('',#87028,#66368,#66369);
#54682=AXIS2_PLACEMENT_3D('',#87029,#66370,#66371);
#54683=AXIS2_PLACEMENT_3D('',#87038,#66376,#66377);
#54684=AXIS2_PLACEMENT_3D('',#87040,#66378,#66379);
#54685=AXIS2_PLACEMENT_3D('',#87042,#66381,#66382);
#54686=AXIS2_PLACEMENT_3D('',#87046,#66385,#66386);
#54687=AXIS2_PLACEMENT_3D('',#87047,#66387,#66388);
#54688=AXIS2_PLACEMENT_3D('',#87048,#66389,#66390);
#54689=AXIS2_PLACEMENT_3D('',#87057,#66395,#66396);
#54690=AXIS2_PLACEMENT_3D('',#87059,#66397,#66398);
#54691=AXIS2_PLACEMENT_3D('',#87061,#66400,#66401);
#54692=AXIS2_PLACEMENT_3D('',#87065,#66404,#66405);
#54693=AXIS2_PLACEMENT_3D('',#87066,#66406,#66407);
#54694=AXIS2_PLACEMENT_3D('',#87067,#66408,#66409);
#54695=AXIS2_PLACEMENT_3D('',#87076,#66414,#66415);
#54696=AXIS2_PLACEMENT_3D('',#87078,#66416,#66417);
#54697=AXIS2_PLACEMENT_3D('',#87080,#66419,#66420);
#54698=AXIS2_PLACEMENT_3D('',#87084,#66423,#66424);
#54699=AXIS2_PLACEMENT_3D('',#87085,#66425,#66426);
#54700=AXIS2_PLACEMENT_3D('',#87086,#66427,#66428);
#54701=AXIS2_PLACEMENT_3D('',#87095,#66433,#66434);
#54702=AXIS2_PLACEMENT_3D('',#87097,#66435,#66436);
#54703=AXIS2_PLACEMENT_3D('',#87099,#66438,#66439);
#54704=AXIS2_PLACEMENT_3D('',#87103,#66442,#66443);
#54705=AXIS2_PLACEMENT_3D('',#87104,#66444,#66445);
#54706=AXIS2_PLACEMENT_3D('',#87105,#66446,#66447);
#54707=AXIS2_PLACEMENT_3D('',#87114,#66452,#66453);
#54708=AXIS2_PLACEMENT_3D('',#87116,#66454,#66455);
#54709=AXIS2_PLACEMENT_3D('',#87118,#66457,#66458);
#54710=AXIS2_PLACEMENT_3D('',#87122,#66461,#66462);
#54711=AXIS2_PLACEMENT_3D('',#87123,#66463,#66464);
#54712=AXIS2_PLACEMENT_3D('',#87124,#66465,#66466);
#54713=AXIS2_PLACEMENT_3D('',#87133,#66471,#66472);
#54714=AXIS2_PLACEMENT_3D('',#87135,#66473,#66474);
#54715=AXIS2_PLACEMENT_3D('',#87137,#66476,#66477);
#54716=AXIS2_PLACEMENT_3D('',#87141,#66480,#66481);
#54717=AXIS2_PLACEMENT_3D('',#87142,#66482,#66483);
#54718=AXIS2_PLACEMENT_3D('',#87143,#66484,#66485);
#54719=AXIS2_PLACEMENT_3D('',#87152,#66490,#66491);
#54720=AXIS2_PLACEMENT_3D('',#87154,#66492,#66493);
#54721=AXIS2_PLACEMENT_3D('',#87156,#66495,#66496);
#54722=AXIS2_PLACEMENT_3D('',#87160,#66499,#66500);
#54723=AXIS2_PLACEMENT_3D('',#87161,#66501,#66502);
#54724=AXIS2_PLACEMENT_3D('',#87162,#66503,#66504);
#54725=AXIS2_PLACEMENT_3D('',#87171,#66509,#66510);
#54726=AXIS2_PLACEMENT_3D('',#87173,#66511,#66512);
#54727=AXIS2_PLACEMENT_3D('',#87175,#66514,#66515);
#54728=AXIS2_PLACEMENT_3D('',#87179,#66518,#66519);
#54729=AXIS2_PLACEMENT_3D('',#87180,#66520,#66521);
#54730=AXIS2_PLACEMENT_3D('',#87181,#66522,#66523);
#54731=AXIS2_PLACEMENT_3D('',#87190,#66528,#66529);
#54732=AXIS2_PLACEMENT_3D('',#87192,#66530,#66531);
#54733=AXIS2_PLACEMENT_3D('',#87194,#66533,#66534);
#54734=AXIS2_PLACEMENT_3D('',#87198,#66537,#66538);
#54735=AXIS2_PLACEMENT_3D('',#87199,#66539,#66540);
#54736=AXIS2_PLACEMENT_3D('',#87200,#66541,#66542);
#54737=AXIS2_PLACEMENT_3D('',#87209,#66547,#66548);
#54738=AXIS2_PLACEMENT_3D('',#87211,#66549,#66550);
#54739=AXIS2_PLACEMENT_3D('',#87213,#66552,#66553);
#54740=AXIS2_PLACEMENT_3D('',#87217,#66556,#66557);
#54741=AXIS2_PLACEMENT_3D('',#87218,#66558,#66559);
#54742=AXIS2_PLACEMENT_3D('',#87219,#66560,#66561);
#54743=AXIS2_PLACEMENT_3D('',#87228,#66566,#66567);
#54744=AXIS2_PLACEMENT_3D('',#87230,#66568,#66569);
#54745=AXIS2_PLACEMENT_3D('',#87232,#66571,#66572);
#54746=AXIS2_PLACEMENT_3D('',#87236,#66575,#66576);
#54747=AXIS2_PLACEMENT_3D('',#87237,#66577,#66578);
#54748=AXIS2_PLACEMENT_3D('',#87238,#66579,#66580);
#54749=AXIS2_PLACEMENT_3D('',#87247,#66585,#66586);
#54750=AXIS2_PLACEMENT_3D('',#87249,#66587,#66588);
#54751=AXIS2_PLACEMENT_3D('',#87251,#66590,#66591);
#54752=AXIS2_PLACEMENT_3D('',#87255,#66594,#66595);
#54753=AXIS2_PLACEMENT_3D('',#87256,#66596,#66597);
#54754=AXIS2_PLACEMENT_3D('',#87257,#66598,#66599);
#54755=AXIS2_PLACEMENT_3D('',#87260,#66600,#66601);
#54756=AXIS2_PLACEMENT_3D('',#87264,#66604,#66605);
#54757=AXIS2_PLACEMENT_3D('',#87270,#66609,#66610);
#54758=AXIS2_PLACEMENT_3D('',#87274,#66613,#66614);
#54759=AXIS2_PLACEMENT_3D('',#87275,#66615,#66616);
#54760=AXIS2_PLACEMENT_3D('',#87276,#66617,#66618);
#54761=AXIS2_PLACEMENT_3D('',#87280,#66620,#66621);
#54762=AXIS2_PLACEMENT_3D('',#87281,#66622,#66623);
#54763=AXIS2_PLACEMENT_3D('',#87290,#66628,#66629);
#54764=AXIS2_PLACEMENT_3D('',#87296,#66633,#66634);
#54765=AXIS2_PLACEMENT_3D('',#87302,#66638,#66639);
#54766=AXIS2_PLACEMENT_3D('',#87308,#66643,#66644);
#54767=AXIS2_PLACEMENT_3D('',#87314,#66648,#66649);
#54768=AXIS2_PLACEMENT_3D('',#87317,#66652,#66653);
#54769=AXIS2_PLACEMENT_3D('',#87318,#66654,#66655);
#54770=AXIS2_PLACEMENT_3D('',#87320,#66656,#66657);
#54771=AXIS2_PLACEMENT_3D('',#87321,#66658,#66659);
#54772=AXIS2_PLACEMENT_3D('',#87323,#66661,#66662);
#54773=AXIS2_PLACEMENT_3D('',#87324,#66663,#66664);
#54774=AXIS2_PLACEMENT_3D('',#87325,#66665,#66666);
#54775=AXIS2_PLACEMENT_3D('',#87326,#66667,#66668);
#54776=AXIS2_PLACEMENT_3D('',#87327,#66669,#66670);
#54777=AXIS2_PLACEMENT_3D('',#87328,#66671,#66672);
#54778=AXIS2_PLACEMENT_3D('',#87329,#66673,#66674);
#54779=AXIS2_PLACEMENT_3D('',#87330,#66675,#66676);
#54780=AXIS2_PLACEMENT_3D('',#87331,#66677,#66678);
#54781=AXIS2_PLACEMENT_3D('',#87332,#66679,#66680);
#54782=AXIS2_PLACEMENT_3D('',#87333,#66681,#66682);
#54783=AXIS2_PLACEMENT_3D('',#87334,#66683,#66684);
#54784=AXIS2_PLACEMENT_3D('',#87335,#66685,#66686);
#54785=AXIS2_PLACEMENT_3D('',#87336,#66687,#66688);
#54786=AXIS2_PLACEMENT_3D('',#87337,#66689,#66690);
#54787=AXIS2_PLACEMENT_3D('',#87338,#66691,#66692);
#54788=AXIS2_PLACEMENT_3D('',#87339,#66693,#66694);
#54789=AXIS2_PLACEMENT_3D('',#87340,#66695,#66696);
#54790=AXIS2_PLACEMENT_3D('',#87342,#66698,#66699);
#54791=AXIS2_PLACEMENT_3D('',#87343,#66700,#66701);
#54792=AXIS2_PLACEMENT_3D('',#87344,#66702,#66703);
#54793=AXIS2_PLACEMENT_3D('',#87345,#66704,#66705);
#54794=AXIS2_PLACEMENT_3D('',#87346,#66706,#66707);
#54795=AXIS2_PLACEMENT_3D('',#87347,#66708,#66709);
#54796=AXIS2_PLACEMENT_3D('',#87348,#66710,#66711);
#54797=AXIS2_PLACEMENT_3D('',#87349,#66712,#66713);
#54798=AXIS2_PLACEMENT_3D('',#87350,#66714,#66715);
#54799=AXIS2_PLACEMENT_3D('',#87351,#66716,#66717);
#54800=AXIS2_PLACEMENT_3D('',#87352,#66718,#66719);
#54801=AXIS2_PLACEMENT_3D('',#87353,#66720,#66721);
#54802=AXIS2_PLACEMENT_3D('',#87354,#66722,#66723);
#54803=AXIS2_PLACEMENT_3D('',#87355,#66724,#66725);
#54804=AXIS2_PLACEMENT_3D('',#87356,#66726,#66727);
#54805=AXIS2_PLACEMENT_3D('',#87357,#66728,#66729);
#54806=AXIS2_PLACEMENT_3D('',#87358,#66730,#66731);
#54807=AXIS2_PLACEMENT_3D('',#87359,#66732,#66733);
#54808=AXIS2_PLACEMENT_3D('',#87360,#66734,#66735);
#54809=AXIS2_PLACEMENT_3D('',#87361,#66736,#66737);
#54810=AXIS2_PLACEMENT_3D('',#87363,#66738,#66739);
#54811=AXIS2_PLACEMENT_3D('',#87365,#66741,#66742);
#65795=DIRECTION('axis',(0.,0.,1.));
#65796=DIRECTION('refdir',(1.,0.,0.));
#65797=DIRECTION('center_axis',(1.,0.,0.));
#65798=DIRECTION('ref_axis',(0.,1.,0.));
#65799=DIRECTION('',(-1.,0.,0.));
#65800=DIRECTION('center_axis',(1.,0.,0.));
#65801=DIRECTION('ref_axis',(0.,1.,0.));
#65802=DIRECTION('center_axis',(1.,0.,0.));
#65803=DIRECTION('ref_axis',(0.,1.,0.));
#65804=DIRECTION('',(-1.,0.,0.));
#65805=DIRECTION('center_axis',(1.,0.,0.));
#65806=DIRECTION('ref_axis',(0.,1.,0.));
#65807=DIRECTION('',(-1.,0.,0.));
#65808=DIRECTION('center_axis',(1.,0.,0.));
#65809=DIRECTION('ref_axis',(0.,1.,0.));
#65810=DIRECTION('',(-1.,0.,0.));
#65811=DIRECTION('center_axis',(1.,0.,0.));
#65812=DIRECTION('ref_axis',(0.,1.,0.));
#65813=DIRECTION('',(-1.,0.,0.));
#65814=DIRECTION('center_axis',(1.,0.,0.));
#65815=DIRECTION('ref_axis',(0.,1.,0.));
#65816=DIRECTION('',(-1.,0.,0.));
#65817=DIRECTION('center_axis',(1.,0.,0.));
#65818=DIRECTION('ref_axis',(0.,1.,0.));
#65819=DIRECTION('',(-1.,0.,0.));
#65820=DIRECTION('center_axis',(1.,0.,0.));
#65821=DIRECTION('ref_axis',(0.,1.,0.));
#65822=DIRECTION('',(-1.,0.,0.));
#65823=DIRECTION('center_axis',(1.,0.,0.));
#65824=DIRECTION('ref_axis',(0.,1.,0.));
#65825=DIRECTION('',(-1.,0.,0.));
#65826=DIRECTION('center_axis',(1.,0.,0.));
#65827=DIRECTION('ref_axis',(0.,1.,0.));
#65828=DIRECTION('',(-1.,0.,0.));
#65829=DIRECTION('center_axis',(1.,0.,0.));
#65830=DIRECTION('ref_axis',(0.,1.,0.));
#65831=DIRECTION('',(-1.,0.,0.));
#65832=DIRECTION('center_axis',(1.,0.,0.));
#65833=DIRECTION('ref_axis',(0.,1.,0.));
#65834=DIRECTION('',(-1.,0.,0.));
#65835=DIRECTION('center_axis',(1.,0.,0.));
#65836=DIRECTION('ref_axis',(0.,1.,0.));
#65837=DIRECTION('',(-1.,0.,0.));
#65838=DIRECTION('center_axis',(1.,0.,0.));
#65839=DIRECTION('ref_axis',(0.,1.,0.));
#65840=DIRECTION('',(-1.,0.,0.));
#65841=DIRECTION('center_axis',(1.,0.,0.));
#65842=DIRECTION('ref_axis',(0.,1.,0.));
#65843=DIRECTION('',(-1.,0.,0.));
#65844=DIRECTION('center_axis',(1.,0.,0.));
#65845=DIRECTION('ref_axis',(0.,1.,0.));
#65846=DIRECTION('',(-1.,0.,0.));
#65847=DIRECTION('center_axis',(1.,0.,0.));
#65848=DIRECTION('ref_axis',(0.,-0.915339016570139,-0.402684100436572));
#65849=DIRECTION('',(1.,0.,0.));
#65850=DIRECTION('center_axis',(1.,0.,0.));
#65851=DIRECTION('ref_axis',(0.,1.,9.48637278455213E-14));
#65852=DIRECTION('center_axis',(1.,0.,0.));
#65853=DIRECTION('ref_axis',(0.,1.,9.48637278455213E-14));
#65854=DIRECTION('',(1.,0.,0.));
#65855=DIRECTION('center_axis',(1.,0.,0.));
#65856=DIRECTION('ref_axis',(0.,1.,9.48637278455213E-14));
#65857=DIRECTION('center_axis',(1.,0.,0.));
#65858=DIRECTION('ref_axis',(0.,1.,9.48637278455213E-14));
#65859=DIRECTION('',(1.,0.,0.));
#65860=DIRECTION('center_axis',(1.,0.,0.));
#65861=DIRECTION('ref_axis',(0.,1.,9.48637278455213E-14));
#65862=DIRECTION('',(1.,0.,0.));
#65863=DIRECTION('center_axis',(1.,0.,0.));
#65864=DIRECTION('ref_axis',(0.,1.,9.48637278455213E-14));
#65865=DIRECTION('',(1.,0.,0.));
#65866=DIRECTION('center_axis',(1.,0.,0.));
#65867=DIRECTION('ref_axis',(0.,1.,9.48637278455213E-14));
#65868=DIRECTION('',(1.,0.,0.));
#65869=DIRECTION('center_axis',(1.,0.,0.));
#65870=DIRECTION('ref_axis',(0.,1.,9.48637278455213E-14));
#65871=DIRECTION('',(1.,0.,0.));
#65872=DIRECTION('center_axis',(1.,0.,0.));
#65873=DIRECTION('ref_axis',(0.,1.,9.48637278455213E-14));
#65874=DIRECTION('',(1.,0.,0.));
#65875=DIRECTION('center_axis',(1.,0.,0.));
#65876=DIRECTION('ref_axis',(0.,1.,9.48637278455213E-14));
#65877=DIRECTION('',(1.,0.,0.));
#65878=DIRECTION('center_axis',(1.,0.,0.));
#65879=DIRECTION('ref_axis',(0.,1.,9.48637278455213E-14));
#65880=DIRECTION('',(1.,0.,0.));
#65881=DIRECTION('center_axis',(1.,0.,0.));
#65882=DIRECTION('ref_axis',(0.,1.,9.48637278455213E-14));
#65883=DIRECTION('',(1.,0.,0.));
#65884=DIRECTION('center_axis',(1.,0.,0.));
#65885=DIRECTION('ref_axis',(0.,1.,9.48637278455213E-14));
#65886=DIRECTION('',(1.,0.,0.));
#65887=DIRECTION('center_axis',(1.,0.,0.));
#65888=DIRECTION('ref_axis',(0.,1.,9.48637278455213E-14));
#65889=DIRECTION('',(1.,0.,0.));
#65890=DIRECTION('center_axis',(1.,0.,0.));
#65891=DIRECTION('ref_axis',(0.,1.,9.48637278455213E-14));
#65892=DIRECTION('',(1.,0.,0.));
#65893=DIRECTION('center_axis',(1.,0.,0.));
#65894=DIRECTION('ref_axis',(0.,1.,9.48637278455213E-14));
#65895=DIRECTION('',(1.,0.,0.));
#65896=DIRECTION('center_axis',(1.,0.,0.));
#65897=DIRECTION('ref_axis',(0.,1.,9.48637278455213E-14));
#65898=DIRECTION('',(1.,0.,0.));
#65899=DIRECTION('center_axis',(1.,0.,0.));
#65900=DIRECTION('ref_axis',(0.,0.,-1.));
#65901=DIRECTION('center_axis',(1.,0.,0.));
#65902=DIRECTION('ref_axis',(0.,1.,0.));
#65903=DIRECTION('center_axis',(1.,0.,0.));
#65904=DIRECTION('ref_axis',(0.,1.,0.));
#65905=DIRECTION('center_axis',(1.,0.,0.));
#65906=DIRECTION('ref_axis',(0.,0.,-1.));
#65907=DIRECTION('center_axis',(1.,0.,0.));
#65908=DIRECTION('ref_axis',(0.,1.,0.));
#65909=DIRECTION('center_axis',(1.,0.,0.));
#65910=DIRECTION('ref_axis',(0.,1.,0.));
#65911=DIRECTION('center_axis',(-1.,0.,0.));
#65912=DIRECTION('ref_axis',(0.,1.,9.48637278455213E-14));
#65913=DIRECTION('center_axis',(1.,0.,0.));
#65914=DIRECTION('ref_axis',(0.,1.,9.48637278455213E-14));
#65915=DIRECTION('center_axis',(1.,0.,0.));
#65916=DIRECTION('ref_axis',(0.,0.,-1.));
#65917=DIRECTION('center_axis',(0.,-1.,-1.22464679914735E-16));
#65918=DIRECTION('ref_axis',(0.,-1.22464679914735E-16,1.));
#65919=DIRECTION('center_axis',(-1.,0.,0.));
#65920=DIRECTION('ref_axis',(0.,1.,0.));
#65921=DIRECTION('center_axis',(1.,0.,0.));
#65922=DIRECTION('ref_axis',(0.,1.,0.));
#65923=DIRECTION('center_axis',(1.,0.,0.));
#65924=DIRECTION('ref_axis',(0.,0.326715465838084,-0.945122745669685));
#65925=DIRECTION('center_axis',(-1.,0.,0.));
#65926=DIRECTION('ref_axis',(0.,0.,1.));
#65927=DIRECTION('center_axis',(1.,0.,0.));
#65928=DIRECTION('ref_axis',(0.,0.,-1.));
#65929=DIRECTION('center_axis',(0.,-0.601539426890005,-0.798843112192153));
#65930=DIRECTION('ref_axis',(0.,0.798843112192152,-0.601539426890005));
#65931=DIRECTION('',(1.,0.,0.));
#65932=DIRECTION('',(0.,-0.798843112192152,0.601539426890005));
#65933=DIRECTION('',(1.,0.,0.));
#65934=DIRECTION('',(0.,0.798843112192152,-0.601539426890005));
#65935=DIRECTION('center_axis',(1.,0.,0.));
#65936=DIRECTION('ref_axis',(0.,-0.17364817766693,-0.984807753012208));
#65937=DIRECTION('center_axis',(1.,0.,0.));
#65938=DIRECTION('ref_axis',(0.,0.,-1.));
#65939=DIRECTION('',(0.,-0.956405578693576,-0.292041724833639));
#65940=DIRECTION('center_axis',(0.,-0.292041724833639,0.956405578693576));
#65941=DIRECTION('ref_axis',(0.,-0.956405578693576,-0.292041724833639));
#65942=DIRECTION('',(-1.,0.,0.));
#65943=DIRECTION('',(0.,0.956405578693576,0.292041724833639));
#65944=DIRECTION('center_axis',(1.,0.,0.));
#65945=DIRECTION('ref_axis',(0.,-0.17364817766693,-0.984807753012208));
#65946=DIRECTION('center_axis',(-1.,0.,0.));
#65947=DIRECTION('ref_axis',(0.,1.,0.));
#65948=DIRECTION('center_axis',(0.,-0.731118342017745,-0.682250665052973));
#65949=DIRECTION('ref_axis',(0.,0.682250665052973,-0.731118342017745));
#65950=DIRECTION('',(1.,0.,0.));
#65951=DIRECTION('',(0.,-0.682250665052973,0.731118342017745));
#65952=DIRECTION('',(1.,0.,0.));
#65953=DIRECTION('',(0.,0.682250665052973,-0.731118342017745));
#65954=DIRECTION('center_axis',(1.,0.,0.));
#65955=DIRECTION('ref_axis',(0.,-0.342020143325669,-0.939692620785908));
#65956=DIRECTION('center_axis',(1.,0.,0.));
#65957=DIRECTION('ref_axis',(0.,0.,-1.));
#65958=DIRECTION('',(0.,-0.992588142241629,-0.1215268689686));
#65959=DIRECTION('center_axis',(0.,-0.1215268689686,0.992588142241629));
#65960=DIRECTION('ref_axis',(0.,-0.992588142241629,-0.1215268689686));
#65961=DIRECTION('',(-1.,0.,0.));
#65962=DIRECTION('',(0.,0.992588142241629,0.1215268689686));
#65963=DIRECTION('center_axis',(1.,0.,0.));
#65964=DIRECTION('ref_axis',(0.,-0.342020143325669,-0.939692620785908));
#65965=DIRECTION('center_axis',(-1.,0.,0.));
#65966=DIRECTION('ref_axis',(0.,1.,0.));
#65967=DIRECTION('center_axis',(0.,-0.838482596287006,-0.544928376691655));
#65968=DIRECTION('ref_axis',(0.,0.544928376691655,-0.838482596287006));
#65969=DIRECTION('',(1.,0.,0.));
#65970=DIRECTION('',(0.,-0.544928376691655,0.838482596287006));
#65971=DIRECTION('',(1.,0.,0.));
#65972=DIRECTION('',(0.,0.544928376691655,-0.838482596287006));
#65973=DIRECTION('center_axis',(1.,0.,0.));
#65974=DIRECTION('ref_axis',(0.,-0.5,-0.866025403784438));
#65975=DIRECTION('center_axis',(1.,0.,0.));
#65976=DIRECTION('ref_axis',(0.,0.,-1.));
#65977=DIRECTION('',(0.,-0.998611417361506,0.052680519314487));
#65978=DIRECTION('center_axis',(0.,0.052680519314487,0.998611417361506));
#65979=DIRECTION('ref_axis',(0.,-0.998611417361506,0.052680519314487));
#65980=DIRECTION('',(-1.,0.,0.));
#65981=DIRECTION('',(0.,0.998611417361506,-0.052680519314487));
#65982=DIRECTION('center_axis',(1.,0.,0.));
#65983=DIRECTION('ref_axis',(0.,-0.5,-0.866025403784438));
#65984=DIRECTION('center_axis',(-1.,0.,0.));
#65985=DIRECTION('ref_axis',(0.,1.,0.));
#65986=DIRECTION('center_axis',(0.,-0.920369981160753,-0.391048715351624));
#65987=DIRECTION('ref_axis',(0.,0.391048715351624,-0.920369981160753));
#65988=DIRECTION('',(1.,0.,0.));
#65989=DIRECTION('',(0.,-0.391048715351624,0.920369981160753));
#65990=DIRECTION('',(1.,0.,0.));
#65991=DIRECTION('',(0.,0.391048715351624,-0.920369981160753));
#65992=DIRECTION('center_axis',(1.,0.,0.));
#65993=DIRECTION('ref_axis',(0.,-0.64278760968654,-0.766044443118978));
#65994=DIRECTION('center_axis',(1.,0.,0.));
#65995=DIRECTION('ref_axis',(0.,0.,-1.));
#65996=DIRECTION('',(0.,-0.974292389886613,0.225287236675832));
#65997=DIRECTION('center_axis',(0.,0.225287236675832,0.974292389886613));
#65998=DIRECTION('ref_axis',(0.,-0.974292389886613,0.225287236675832));
#65999=DIRECTION('',(-1.,0.,0.));
#66000=DIRECTION('',(0.,0.974292389886613,-0.225287236675832));
#66001=DIRECTION('center_axis',(1.,0.,0.));
#66002=DIRECTION('ref_axis',(0.,-0.64278760968654,-0.766044443118978));
#66003=DIRECTION('center_axis',(-1.,0.,0.));
#66004=DIRECTION('ref_axis',(0.,1.,0.));
#66005=DIRECTION('center_axis',(0.,-0.974292389886613,-0.225287236675831));
#66006=DIRECTION('ref_axis',(0.,0.225287236675831,-0.974292389886613));
#66007=DIRECTION('',(1.,0.,0.));
#66008=DIRECTION('',(0.,-0.225287236675831,0.974292389886613));
#66009=DIRECTION('',(1.,0.,0.));
#66010=DIRECTION('',(0.,0.225287236675831,-0.974292389886613));
#66011=DIRECTION('center_axis',(1.,0.,0.));
#66012=DIRECTION('ref_axis',(0.,-0.766044443118978,-0.642787609686539));
#66013=DIRECTION('center_axis',(1.,0.,0.));
#66014=DIRECTION('ref_axis',(0.,0.,-1.));
#66015=DIRECTION('',(0.,-0.920369981160753,0.391048715351624));
#66016=DIRECTION('center_axis',(0.,0.391048715351624,0.920369981160753));
#66017=DIRECTION('ref_axis',(0.,-0.920369981160753,0.391048715351624));
#66018=DIRECTION('',(-1.,0.,0.));
#66019=DIRECTION('',(0.,0.920369981160753,-0.391048715351624));
#66020=DIRECTION('center_axis',(1.,0.,0.));
#66021=DIRECTION('ref_axis',(0.,-0.766044443118978,-0.642787609686539));
#66022=DIRECTION('center_axis',(-1.,0.,0.));
#66023=DIRECTION('ref_axis',(0.,1.,0.));
#66024=DIRECTION('center_axis',(0.,-0.998611417361506,-0.0526805193144866));
#66025=DIRECTION('ref_axis',(0.,0.0526805193144866,-0.998611417361506));
#66026=DIRECTION('',(1.,0.,0.));
#66027=DIRECTION('',(0.,-0.0526805193144866,0.998611417361506));
#66028=DIRECTION('',(1.,0.,0.));
#66029=DIRECTION('',(0.,0.0526805193144866,-0.998611417361506));
#66030=DIRECTION('center_axis',(1.,0.,0.));
#66031=DIRECTION('ref_axis',(0.,-0.866025403784439,-0.5));
#66032=DIRECTION('center_axis',(1.,0.,0.));
#66033=DIRECTION('ref_axis',(0.,0.,-1.));
#66034=DIRECTION('',(0.,-0.838482596287006,0.544928376691655));
#66035=DIRECTION('center_axis',(0.,0.544928376691655,0.838482596287006));
#66036=DIRECTION('ref_axis',(0.,-0.838482596287006,0.544928376691655));
#66037=DIRECTION('',(-1.,0.,0.));
#66038=DIRECTION('',(0.,0.838482596287006,-0.544928376691655));
#66039=DIRECTION('center_axis',(1.,0.,0.));
#66040=DIRECTION('ref_axis',(0.,-0.866025403784439,-0.5));
#66041=DIRECTION('center_axis',(-1.,0.,0.));
#66042=DIRECTION('ref_axis',(0.,1.,0.));
#66043=DIRECTION('center_axis',(0.,-0.992588142241629,0.121526868968601));
#66044=DIRECTION('ref_axis',(0.,-0.121526868968601,-0.992588142241629));
#66045=DIRECTION('',(1.,0.,0.));
#66046=DIRECTION('',(0.,0.121526868968601,0.992588142241629));
#66047=DIRECTION('',(1.,0.,0.));
#66048=DIRECTION('',(0.,-0.121526868968601,-0.992588142241629));
#66049=DIRECTION('center_axis',(1.,0.,0.));
#66050=DIRECTION('ref_axis',(0.,-0.939692620785909,-0.342020143325668));
#66051=DIRECTION('center_axis',(1.,0.,0.));
#66052=DIRECTION('ref_axis',(0.,0.,-1.));
#66053=DIRECTION('',(0.,-0.731118342017744,0.682250665052974));
#66054=DIRECTION('center_axis',(0.,0.682250665052974,0.731118342017744));
#66055=DIRECTION('ref_axis',(0.,-0.731118342017744,0.682250665052974));
#66056=DIRECTION('',(-1.,0.,0.));
#66057=DIRECTION('',(0.,0.731118342017744,-0.682250665052974));
#66058=DIRECTION('center_axis',(1.,0.,0.));
#66059=DIRECTION('ref_axis',(0.,-0.939692620785909,-0.342020143325668));
#66060=DIRECTION('center_axis',(-1.,0.,0.));
#66061=DIRECTION('ref_axis',(0.,1.,0.));
#66062=DIRECTION('center_axis',(0.,-0.956405578693575,0.292041724833639));
#66063=DIRECTION('ref_axis',(0.,-0.292041724833639,-0.956405578693575));
#66064=DIRECTION('',(1.,0.,0.));
#66065=DIRECTION('',(0.,0.292041724833639,0.956405578693575));
#66066=DIRECTION('',(1.,0.,0.));
#66067=DIRECTION('',(0.,-0.292041724833639,-0.956405578693575));
#66068=DIRECTION('center_axis',(1.,0.,0.));
#66069=DIRECTION('ref_axis',(0.,-0.984807753012208,-0.17364817766693));
#66070=DIRECTION('center_axis',(1.,0.,0.));
#66071=DIRECTION('ref_axis',(0.,0.,-1.));
#66072=DIRECTION('',(0.,-0.601539426890005,0.798843112192153));
#66073=DIRECTION('center_axis',(0.,0.798843112192153,0.601539426890005));
#66074=DIRECTION('ref_axis',(0.,-0.601539426890005,0.798843112192153));
#66075=DIRECTION('',(-1.,0.,0.));
#66076=DIRECTION('',(0.,0.601539426890005,-0.798843112192153));
#66077=DIRECTION('center_axis',(1.,0.,0.));
#66078=DIRECTION('ref_axis',(0.,-0.984807753012208,-0.17364817766693));
#66079=DIRECTION('center_axis',(-1.,0.,0.));
#66080=DIRECTION('ref_axis',(0.,1.,0.));
#66081=DIRECTION('center_axis',(0.,-0.891163115601492,0.453683040669851));
#66082=DIRECTION('ref_axis',(0.,-0.453683040669851,-0.891163115601492));
#66083=DIRECTION('',(1.,0.,0.));
#66084=DIRECTION('',(0.,0.453683040669851,0.891163115601492));
#66085=DIRECTION('',(1.,0.,0.));
#66086=DIRECTION('',(0.,-0.453683040669851,-0.891163115601492));
#66087=DIRECTION('center_axis',(1.,0.,0.));
#66088=DIRECTION('ref_axis',(0.,-1.,1.83697019872103E-16));
#66089=DIRECTION('center_axis',(1.,0.,0.));
#66090=DIRECTION('ref_axis',(0.,0.,-1.));
#66091=DIRECTION('',(0.,-0.453683040669851,0.891163115601492));
#66092=DIRECTION('center_axis',(0.,0.891163115601492,0.453683040669851));
#66093=DIRECTION('ref_axis',(0.,-0.453683040669851,0.891163115601492));
#66094=DIRECTION('',(-1.,0.,0.));
#66095=DIRECTION('',(0.,0.453683040669851,-0.891163115601492));
#66096=DIRECTION('center_axis',(1.,0.,0.));
#66097=DIRECTION('ref_axis',(0.,-1.,1.83697019872103E-16));
#66098=DIRECTION('center_axis',(-1.,0.,0.));
#66099=DIRECTION('ref_axis',(0.,1.,0.));
#66100=DIRECTION('center_axis',(0.,-0.798843112192153,0.601539426890005));
#66101=DIRECTION('ref_axis',(0.,-0.601539426890005,-0.798843112192153));
#66102=DIRECTION('',(1.,0.,0.));
#66103=DIRECTION('',(0.,0.601539426890005,0.798843112192153));
#66104=DIRECTION('',(1.,0.,0.));
#66105=DIRECTION('',(0.,-0.601539426890005,-0.798843112192153));
#66106=DIRECTION('center_axis',(1.,0.,0.));
#66107=DIRECTION('ref_axis',(0.,-0.984807753012208,0.17364817766693));
#66108=DIRECTION('center_axis',(1.,0.,0.));
#66109=DIRECTION('ref_axis',(0.,0.,-1.));
#66110=DIRECTION('',(0.,-0.292041724833639,0.956405578693576));
#66111=DIRECTION('center_axis',(0.,0.956405578693576,0.292041724833639));
#66112=DIRECTION('ref_axis',(0.,-0.292041724833639,0.956405578693576));
#66113=DIRECTION('',(-1.,0.,0.));
#66114=DIRECTION('',(0.,0.292041724833639,-0.956405578693576));
#66115=DIRECTION('center_axis',(1.,0.,0.));
#66116=DIRECTION('ref_axis',(0.,-0.984807753012208,0.17364817766693));
#66117=DIRECTION('center_axis',(-1.,0.,0.));
#66118=DIRECTION('ref_axis',(0.,1.,0.));
#66119=DIRECTION('center_axis',(0.,-0.682250665052973,0.731118342017745));
#66120=DIRECTION('ref_axis',(0.,-0.731118342017745,-0.682250665052973));
#66121=DIRECTION('',(1.,0.,0.));
#66122=DIRECTION('',(0.,0.731118342017745,0.682250665052973));
#66123=DIRECTION('',(1.,0.,0.));
#66124=DIRECTION('',(0.,-0.731118342017745,-0.682250665052973));
#66125=DIRECTION('center_axis',(1.,0.,0.));
#66126=DIRECTION('ref_axis',(0.,-0.939692620785908,0.342020143325669));
#66127=DIRECTION('center_axis',(1.,0.,0.));
#66128=DIRECTION('ref_axis',(0.,0.,-1.));
#66129=DIRECTION('',(0.,-0.1215268689686,0.992588142241629));
#66130=DIRECTION('center_axis',(0.,0.992588142241629,0.1215268689686));
#66131=DIRECTION('ref_axis',(0.,-0.1215268689686,0.992588142241629));
#66132=DIRECTION('',(-1.,0.,0.));
#66133=DIRECTION('',(0.,0.1215268689686,-0.992588142241629));
#66134=DIRECTION('center_axis',(1.,0.,0.));
#66135=DIRECTION('ref_axis',(0.,-0.939692620785908,0.342020143325669));
#66136=DIRECTION('center_axis',(-1.,0.,0.));
#66137=DIRECTION('ref_axis',(0.,1.,0.));
#66138=DIRECTION('center_axis',(0.,-0.544928376691655,0.838482596287006));
#66139=DIRECTION('ref_axis',(0.,-0.838482596287006,-0.544928376691655));
#66140=DIRECTION('',(1.,0.,0.));
#66141=DIRECTION('',(0.,0.838482596287006,0.544928376691655));
#66142=DIRECTION('',(1.,0.,0.));
#66143=DIRECTION('',(0.,-0.838482596287006,-0.544928376691655));
#66144=DIRECTION('center_axis',(1.,0.,0.));
#66145=DIRECTION('ref_axis',(0.,-0.866025403784438,0.5));
#66146=DIRECTION('center_axis',(1.,0.,0.));
#66147=DIRECTION('ref_axis',(0.,0.,-1.));
#66148=DIRECTION('',(0.,0.052680519314487,0.998611417361506));
#66149=DIRECTION('center_axis',(0.,0.998611417361506,-0.052680519314487));
#66150=DIRECTION('ref_axis',(0.,0.052680519314487,0.998611417361506));
#66151=DIRECTION('',(-1.,0.,0.));
#66152=DIRECTION('',(0.,-0.052680519314487,-0.998611417361506));
#66153=DIRECTION('center_axis',(1.,0.,0.));
#66154=DIRECTION('ref_axis',(0.,-0.866025403784438,0.5));
#66155=DIRECTION('center_axis',(-1.,0.,0.));
#66156=DIRECTION('ref_axis',(0.,1.,0.));
#66157=DIRECTION('center_axis',(0.,-0.391048715351624,0.920369981160753));
#66158=DIRECTION('ref_axis',(0.,-0.920369981160753,-0.391048715351624));
#66159=DIRECTION('',(1.,0.,0.));
#66160=DIRECTION('',(0.,0.920369981160753,0.391048715351624));
#66161=DIRECTION('',(1.,0.,0.));
#66162=DIRECTION('',(0.,-0.920369981160753,-0.391048715351624));
#66163=DIRECTION('center_axis',(1.,0.,0.));
#66164=DIRECTION('ref_axis',(0.,-0.766044443118978,0.642787609686539));
#66165=DIRECTION('center_axis',(1.,0.,0.));
#66166=DIRECTION('ref_axis',(0.,0.,-1.));
#66167=DIRECTION('',(0.,0.225287236675832,0.974292389886613));
#66168=DIRECTION('center_axis',(0.,0.974292389886613,-0.225287236675832));
#66169=DIRECTION('ref_axis',(0.,0.225287236675832,0.974292389886613));
#66170=DIRECTION('',(-1.,0.,0.));
#66171=DIRECTION('',(0.,-0.225287236675832,-0.974292389886613));
#66172=DIRECTION('center_axis',(1.,0.,0.));
#66173=DIRECTION('ref_axis',(0.,-0.766044443118978,0.642787609686539));
#66174=DIRECTION('center_axis',(-1.,0.,0.));
#66175=DIRECTION('ref_axis',(0.,1.,0.));
#66176=DIRECTION('center_axis',(0.,-0.225287236675832,0.974292389886613));
#66177=DIRECTION('ref_axis',(0.,-0.974292389886613,-0.225287236675832));
#66178=DIRECTION('',(1.,0.,0.));
#66179=DIRECTION('',(0.,0.974292389886613,0.225287236675832));
#66180=DIRECTION('',(1.,0.,0.));
#66181=DIRECTION('',(0.,-0.974292389886613,-0.225287236675832));
#66182=DIRECTION('center_axis',(1.,0.,0.));
#66183=DIRECTION('ref_axis',(0.,-0.642787609686539,0.766044443118978));
#66184=DIRECTION('center_axis',(1.,0.,0.));
#66185=DIRECTION('ref_axis',(0.,0.,-1.));
#66186=DIRECTION('',(0.,0.391048715351624,0.920369981160753));
#66187=DIRECTION('center_axis',(0.,0.920369981160753,-0.391048715351624));
#66188=DIRECTION('ref_axis',(0.,0.391048715351624,0.920369981160753));
#66189=DIRECTION('',(-1.,0.,0.));
#66190=DIRECTION('',(0.,-0.391048715351624,-0.920369981160753));
#66191=DIRECTION('center_axis',(1.,0.,0.));
#66192=DIRECTION('ref_axis',(0.,-0.642787609686539,0.766044443118978));
#66193=DIRECTION('center_axis',(-1.,0.,0.));
#66194=DIRECTION('ref_axis',(0.,1.,0.));
#66195=DIRECTION('center_axis',(0.,-0.0526805193144861,0.998611417361506));
#66196=DIRECTION('ref_axis',(0.,-0.998611417361506,-0.0526805193144861));
#66197=DIRECTION('',(1.,0.,0.));
#66198=DIRECTION('',(0.,0.998611417361506,0.0526805193144861));
#66199=DIRECTION('',(1.,0.,0.));
#66200=DIRECTION('',(0.,-0.998611417361506,-0.0526805193144861));
#66201=DIRECTION('center_axis',(1.,0.,0.));
#66202=DIRECTION('ref_axis',(0.,-0.5,0.866025403784439));
#66203=DIRECTION('center_axis',(1.,0.,0.));
#66204=DIRECTION('ref_axis',(0.,0.,-1.));
#66205=DIRECTION('',(0.,0.544928376691655,0.838482596287005));
#66206=DIRECTION('center_axis',(0.,0.838482596287005,-0.544928376691655));
#66207=DIRECTION('ref_axis',(0.,0.544928376691655,0.838482596287005));
#66208=DIRECTION('',(-1.,0.,0.));
#66209=DIRECTION('',(0.,-0.544928376691655,-0.838482596287005));
#66210=DIRECTION('center_axis',(1.,0.,0.));
#66211=DIRECTION('ref_axis',(0.,-0.5,0.866025403784439));
#66212=DIRECTION('center_axis',(-1.,0.,0.));
#66213=DIRECTION('ref_axis',(0.,1.,0.));
#66214=DIRECTION('center_axis',(0.,0.1215268689686,0.992588142241629));
#66215=DIRECTION('ref_axis',(0.,-0.992588142241629,0.1215268689686));
#66216=DIRECTION('',(1.,0.,0.));
#66217=DIRECTION('',(0.,0.992588142241629,-0.1215268689686));
#66218=DIRECTION('',(1.,0.,0.));
#66219=DIRECTION('',(0.,-0.992588142241629,0.1215268689686));
#66220=DIRECTION('center_axis',(1.,0.,0.));
#66221=DIRECTION('ref_axis',(0.,-0.342020143325669,0.939692620785909));
#66222=DIRECTION('center_axis',(1.,0.,0.));
#66223=DIRECTION('ref_axis',(0.,0.,-1.));
#66224=DIRECTION('',(0.,0.682250665052974,0.731118342017744));
#66225=DIRECTION('center_axis',(0.,0.731118342017744,-0.682250665052974));
#66226=DIRECTION('ref_axis',(0.,0.682250665052974,0.731118342017744));
#66227=DIRECTION('',(-1.,0.,0.));
#66228=DIRECTION('',(0.,-0.682250665052974,-0.731118342017744));
#66229=DIRECTION('center_axis',(1.,0.,0.));
#66230=DIRECTION('ref_axis',(0.,-0.342020143325669,0.939692620785909));
#66231=DIRECTION('center_axis',(-1.,0.,0.));
#66232=DIRECTION('ref_axis',(0.,1.,0.));
#66233=DIRECTION('center_axis',(0.,0.292041724833639,0.956405578693575));
#66234=DIRECTION('ref_axis',(0.,-0.956405578693575,0.292041724833639));
#66235=DIRECTION('',(1.,0.,0.));
#66236=DIRECTION('',(0.,0.956405578693575,-0.292041724833639));
#66237=DIRECTION('',(1.,0.,0.));
#66238=DIRECTION('',(0.,-0.956405578693575,0.292041724833639));
#66239=DIRECTION('center_axis',(1.,0.,0.));
#66240=DIRECTION('ref_axis',(0.,-0.17364817766693,0.984807753012208));
#66241=DIRECTION('center_axis',(1.,0.,0.));
#66242=DIRECTION('ref_axis',(0.,0.,-1.));
#66243=DIRECTION('',(0.,0.798843112192153,0.601539426890005));
#66244=DIRECTION('center_axis',(0.,0.601539426890005,-0.798843112192153));
#66245=DIRECTION('ref_axis',(0.,0.798843112192153,0.601539426890005));
#66246=DIRECTION('',(-1.,0.,0.));
#66247=DIRECTION('',(0.,-0.798843112192153,-0.601539426890005));
#66248=DIRECTION('center_axis',(1.,0.,0.));
#66249=DIRECTION('ref_axis',(0.,-0.17364817766693,0.984807753012208));
#66250=DIRECTION('center_axis',(-1.,0.,0.));
#66251=DIRECTION('ref_axis',(0.,1.,0.));
#66252=DIRECTION('center_axis',(0.,0.453683040669851,0.891163115601492));
#66253=DIRECTION('ref_axis',(0.,-0.891163115601492,0.453683040669851));
#66254=DIRECTION('',(1.,0.,0.));
#66255=DIRECTION('',(0.,0.891163115601492,-0.453683040669851));
#66256=DIRECTION('',(1.,0.,0.));
#66257=DIRECTION('',(0.,-0.891163115601492,0.453683040669851));
#66258=DIRECTION('center_axis',(1.,0.,0.));
#66259=DIRECTION('ref_axis',(0.,1.22464679914735E-16,1.));
#66260=DIRECTION('center_axis',(1.,0.,0.));
#66261=DIRECTION('ref_axis',(0.,0.,-1.));
#66262=DIRECTION('',(0.,0.891163115601492,0.453683040669851));
#66263=DIRECTION('center_axis',(1.,0.,0.));
#66264=DIRECTION('ref_axis',(0.,0.,-1.));
#66265=DIRECTION('center_axis',(0.,0.453683040669851,-0.891163115601492));
#66266=DIRECTION('ref_axis',(0.,0.891163115601492,0.453683040669851));
#66267=DIRECTION('',(-1.,0.,0.));
#66268=DIRECTION('',(0.,-0.891163115601492,-0.453683040669851));
#66269=DIRECTION('center_axis',(1.,0.,0.));
#66270=DIRECTION('ref_axis',(0.,1.22464679914735E-16,1.));
#66271=DIRECTION('center_axis',(-1.,0.,0.));
#66272=DIRECTION('ref_axis',(0.,1.,0.));
#66273=DIRECTION('center_axis',(-1.,0.,0.));
#66274=DIRECTION('ref_axis',(0.,1.,0.));
#66275=DIRECTION('center_axis',(0.,0.601539426890006,0.798843112192152));
#66276=DIRECTION('ref_axis',(0.,-0.798843112192152,0.601539426890006));
#66277=DIRECTION('',(1.,0.,0.));
#66278=DIRECTION('',(0.,0.798843112192152,-0.601539426890006));
#66279=DIRECTION('',(1.,0.,0.));
#66280=DIRECTION('',(0.,-0.798843112192152,0.601539426890006));
#66281=DIRECTION('center_axis',(1.,0.,0.));
#66282=DIRECTION('ref_axis',(0.,0.173648177666931,0.984807753012208));
#66283=DIRECTION('center_axis',(1.,0.,0.));
#66284=DIRECTION('ref_axis',(0.,0.,-1.));
#66285=DIRECTION('',(0.,0.956405578693576,0.292041724833639));
#66286=DIRECTION('center_axis',(0.,0.292041724833639,-0.956405578693576));
#66287=DIRECTION('ref_axis',(0.,0.956405578693576,0.292041724833639));
#66288=DIRECTION('',(-1.,0.,0.));
#66289=DIRECTION('',(0.,-0.956405578693576,-0.292041724833639));
#66290=DIRECTION('center_axis',(1.,0.,0.));
#66291=DIRECTION('ref_axis',(0.,0.173648177666931,0.984807753012208));
#66292=DIRECTION('center_axis',(-1.,0.,0.));
#66293=DIRECTION('ref_axis',(0.,1.,0.));
#66294=DIRECTION('center_axis',(0.,0.731118342017744,0.682250665052974));
#66295=DIRECTION('ref_axis',(0.,-0.682250665052974,0.731118342017744));
#66296=DIRECTION('',(1.,0.,0.));
#66297=DIRECTION('',(0.,0.682250665052974,-0.731118342017744));
#66298=DIRECTION('',(1.,0.,0.));
#66299=DIRECTION('',(0.,-0.682250665052974,0.731118342017744));
#66300=DIRECTION('center_axis',(1.,0.,0.));
#66301=DIRECTION('ref_axis',(0.,0.342020143325669,0.939692620785908));
#66302=DIRECTION('center_axis',(1.,0.,0.));
#66303=DIRECTION('ref_axis',(0.,0.,-1.));
#66304=DIRECTION('',(0.,0.992588142241629,0.1215268689686));
#66305=DIRECTION('center_axis',(0.,0.1215268689686,-0.992588142241629));
#66306=DIRECTION('ref_axis',(0.,0.992588142241629,0.1215268689686));
#66307=DIRECTION('',(-1.,0.,0.));
#66308=DIRECTION('',(0.,-0.992588142241629,-0.1215268689686));
#66309=DIRECTION('center_axis',(1.,0.,0.));
#66310=DIRECTION('ref_axis',(0.,0.342020143325669,0.939692620785908));
#66311=DIRECTION('center_axis',(-1.,0.,0.));
#66312=DIRECTION('ref_axis',(0.,1.,0.));
#66313=DIRECTION('center_axis',(0.,0.838482596287006,0.544928376691655));
#66314=DIRECTION('ref_axis',(0.,-0.544928376691655,0.838482596287006));
#66315=DIRECTION('',(1.,0.,0.));
#66316=DIRECTION('',(0.,0.544928376691655,-0.838482596287006));
#66317=DIRECTION('',(1.,0.,0.));
#66318=DIRECTION('',(0.,-0.544928376691655,0.838482596287006));
#66319=DIRECTION('center_axis',(1.,0.,0.));
#66320=DIRECTION('ref_axis',(0.,0.5,0.866025403784439));
#66321=DIRECTION('center_axis',(1.,0.,0.));
#66322=DIRECTION('ref_axis',(0.,0.,-1.));
#66323=DIRECTION('',(0.,0.998611417361506,-0.0526805193144864));
#66324=DIRECTION('center_axis',(0.,-0.0526805193144864,-0.998611417361506));
#66325=DIRECTION('ref_axis',(0.,0.998611417361506,-0.0526805193144864));
#66326=DIRECTION('',(-1.,0.,0.));
#66327=DIRECTION('',(0.,-0.998611417361506,0.0526805193144864));
#66328=DIRECTION('center_axis',(1.,0.,0.));
#66329=DIRECTION('ref_axis',(0.,0.5,0.866025403784439));
#66330=DIRECTION('center_axis',(-1.,0.,0.));
#66331=DIRECTION('ref_axis',(0.,1.,0.));
#66332=DIRECTION('center_axis',(0.,0.920369981160753,0.391048715351624));
#66333=DIRECTION('ref_axis',(0.,-0.391048715351624,0.920369981160753));
#66334=DIRECTION('',(1.,0.,0.));
#66335=DIRECTION('',(0.,0.391048715351624,-0.920369981160753));
#66336=DIRECTION('',(1.,0.,0.));
#66337=DIRECTION('',(0.,-0.391048715351624,0.920369981160753));
#66338=DIRECTION('center_axis',(1.,0.,0.));
#66339=DIRECTION('ref_axis',(0.,0.642787609686539,0.766044443118978));
#66340=DIRECTION('center_axis',(1.,0.,0.));
#66341=DIRECTION('ref_axis',(0.,0.,-1.));
#66342=DIRECTION('',(0.,0.974292389886613,-0.225287236675832));
#66343=DIRECTION('center_axis',(0.,-0.225287236675832,-0.974292389886613));
#66344=DIRECTION('ref_axis',(0.,0.974292389886613,-0.225287236675832));
#66345=DIRECTION('',(-1.,0.,0.));
#66346=DIRECTION('',(0.,-0.974292389886613,0.225287236675832));
#66347=DIRECTION('center_axis',(1.,0.,0.));
#66348=DIRECTION('ref_axis',(0.,0.642787609686539,0.766044443118978));
#66349=DIRECTION('center_axis',(-1.,0.,0.));
#66350=DIRECTION('ref_axis',(0.,1.,0.));
#66351=DIRECTION('center_axis',(0.,0.974292389886613,0.225287236675832));
#66352=DIRECTION('ref_axis',(0.,-0.225287236675832,0.974292389886613));
#66353=DIRECTION('',(1.,0.,0.));
#66354=DIRECTION('',(0.,0.225287236675832,-0.974292389886613));
#66355=DIRECTION('',(1.,0.,0.));
#66356=DIRECTION('',(0.,-0.225287236675832,0.974292389886613));
#66357=DIRECTION('center_axis',(1.,0.,0.));
#66358=DIRECTION('ref_axis',(0.,0.766044443118978,0.642787609686539));
#66359=DIRECTION('center_axis',(1.,0.,0.));
#66360=DIRECTION('ref_axis',(0.,0.,-1.));
#66361=DIRECTION('',(0.,0.920369981160753,-0.391048715351624));
#66362=DIRECTION('center_axis',(0.,-0.391048715351624,-0.920369981160753));
#66363=DIRECTION('ref_axis',(0.,0.920369981160753,-0.391048715351624));
#66364=DIRECTION('',(-1.,0.,0.));
#66365=DIRECTION('',(0.,-0.920369981160753,0.391048715351624));
#66366=DIRECTION('center_axis',(1.,0.,0.));
#66367=DIRECTION('ref_axis',(0.,0.766044443118978,0.642787609686539));
#66368=DIRECTION('center_axis',(-1.,0.,0.));
#66369=DIRECTION('ref_axis',(0.,1.,0.));
#66370=DIRECTION('center_axis',(0.,0.998611417361506,0.0526805193144862));
#66371=DIRECTION('ref_axis',(0.,-0.0526805193144862,0.998611417361506));
#66372=DIRECTION('',(1.,0.,0.));
#66373=DIRECTION('',(0.,0.0526805193144862,-0.998611417361506));
#66374=DIRECTION('',(1.,0.,0.));
#66375=DIRECTION('',(0.,-0.0526805193144862,0.998611417361506));
#66376=DIRECTION('center_axis',(1.,0.,0.));
#66377=DIRECTION('ref_axis',(0.,0.866025403784439,0.5));
#66378=DIRECTION('center_axis',(1.,0.,0.));
#66379=DIRECTION('ref_axis',(0.,0.,-1.));
#66380=DIRECTION('',(0.,0.838482596287005,-0.544928376691655));
#66381=DIRECTION('center_axis',(0.,-0.544928376691655,-0.838482596287005));
#66382=DIRECTION('ref_axis',(0.,0.838482596287005,-0.544928376691655));
#66383=DIRECTION('',(-1.,0.,0.));
#66384=DIRECTION('',(0.,-0.838482596287005,0.544928376691655));
#66385=DIRECTION('center_axis',(1.,0.,0.));
#66386=DIRECTION('ref_axis',(0.,0.866025403784439,0.5));
#66387=DIRECTION('center_axis',(-1.,0.,0.));
#66388=DIRECTION('ref_axis',(0.,1.,0.));
#66389=DIRECTION('center_axis',(0.,0.992588142241629,-0.1215268689686));
#66390=DIRECTION('ref_axis',(0.,0.1215268689686,0.992588142241629));
#66391=DIRECTION('',(1.,0.,0.));
#66392=DIRECTION('',(0.,-0.1215268689686,-0.992588142241629));
#66393=DIRECTION('',(1.,0.,0.));
#66394=DIRECTION('',(0.,0.1215268689686,0.992588142241629));
#66395=DIRECTION('center_axis',(1.,0.,0.));
#66396=DIRECTION('ref_axis',(0.,0.939692620785908,0.342020143325669));
#66397=DIRECTION('center_axis',(1.,0.,0.));
#66398=DIRECTION('ref_axis',(0.,0.,-1.));
#66399=DIRECTION('',(0.,0.731118342017744,-0.682250665052974));
#66400=DIRECTION('center_axis',(0.,-0.682250665052974,-0.731118342017744));
#66401=DIRECTION('ref_axis',(0.,0.731118342017744,-0.682250665052974));
#66402=DIRECTION('',(-1.,0.,0.));
#66403=DIRECTION('',(0.,-0.731118342017744,0.682250665052974));
#66404=DIRECTION('center_axis',(1.,0.,0.));
#66405=DIRECTION('ref_axis',(0.,0.939692620785908,0.342020143325669));
#66406=DIRECTION('center_axis',(-1.,0.,0.));
#66407=DIRECTION('ref_axis',(0.,1.,0.));
#66408=DIRECTION('center_axis',(0.,0.956405578693576,-0.292041724833639));
#66409=DIRECTION('ref_axis',(0.,0.292041724833639,0.956405578693576));
#66410=DIRECTION('',(1.,0.,0.));
#66411=DIRECTION('',(0.,-0.292041724833639,-0.956405578693576));
#66412=DIRECTION('',(1.,0.,0.));
#66413=DIRECTION('',(0.,0.292041724833639,0.956405578693576));
#66414=DIRECTION('center_axis',(1.,0.,0.));
#66415=DIRECTION('ref_axis',(0.,0.984807753012208,0.17364817766693));
#66416=DIRECTION('center_axis',(1.,0.,0.));
#66417=DIRECTION('ref_axis',(0.,0.,-1.));
#66418=DIRECTION('',(0.,0.601539426890005,-0.798843112192153));
#66419=DIRECTION('center_axis',(0.,-0.798843112192153,-0.601539426890005));
#66420=DIRECTION('ref_axis',(0.,0.601539426890005,-0.798843112192153));
#66421=DIRECTION('',(-1.,0.,0.));
#66422=DIRECTION('',(0.,-0.601539426890005,0.798843112192153));
#66423=DIRECTION('center_axis',(1.,0.,0.));
#66424=DIRECTION('ref_axis',(0.,0.984807753012208,0.17364817766693));
#66425=DIRECTION('center_axis',(-1.,0.,0.));
#66426=DIRECTION('ref_axis',(0.,1.,0.));
#66427=DIRECTION('center_axis',(0.,0.891163115601492,-0.453683040669851));
#66428=DIRECTION('ref_axis',(0.,0.453683040669851,0.891163115601492));
#66429=DIRECTION('',(1.,0.,0.));
#66430=DIRECTION('',(0.,-0.453683040669851,-0.891163115601492));
#66431=DIRECTION('',(1.,0.,0.));
#66432=DIRECTION('',(0.,0.453683040669851,0.891163115601492));
#66433=DIRECTION('center_axis',(1.,0.,0.));
#66434=DIRECTION('ref_axis',(0.,1.,-6.12323399573677E-17));
#66435=DIRECTION('center_axis',(1.,0.,0.));
#66436=DIRECTION('ref_axis',(0.,0.,-1.));
#66437=DIRECTION('',(0.,0.453683040669851,-0.891163115601492));
#66438=DIRECTION('center_axis',(0.,-0.891163115601492,-0.453683040669851));
#66439=DIRECTION('ref_axis',(0.,0.453683040669851,-0.891163115601492));
#66440=DIRECTION('',(-1.,0.,0.));
#66441=DIRECTION('',(0.,-0.453683040669851,0.891163115601492));
#66442=DIRECTION('center_axis',(1.,0.,0.));
#66443=DIRECTION('ref_axis',(0.,1.,-6.12323399573677E-17));
#66444=DIRECTION('center_axis',(-1.,0.,0.));
#66445=DIRECTION('ref_axis',(0.,1.,0.));
#66446=DIRECTION('center_axis',(0.,0.798843112192153,-0.601539426890005));
#66447=DIRECTION('ref_axis',(0.,0.601539426890005,0.798843112192152));
#66448=DIRECTION('',(1.,0.,0.));
#66449=DIRECTION('',(0.,-0.601539426890005,-0.798843112192152));
#66450=DIRECTION('',(1.,0.,0.));
#66451=DIRECTION('',(0.,0.601539426890005,0.798843112192152));
#66452=DIRECTION('center_axis',(1.,0.,0.));
#66453=DIRECTION('ref_axis',(0.,0.984807753012208,-0.17364817766693));
#66454=DIRECTION('center_axis',(1.,0.,0.));
#66455=DIRECTION('ref_axis',(0.,0.,-1.));
#66456=DIRECTION('',(0.,0.292041724833639,-0.956405578693576));
#66457=DIRECTION('center_axis',(0.,-0.956405578693576,-0.292041724833639));
#66458=DIRECTION('ref_axis',(0.,0.292041724833639,-0.956405578693576));
#66459=DIRECTION('',(-1.,0.,0.));
#66460=DIRECTION('',(0.,-0.292041724833639,0.956405578693576));
#66461=DIRECTION('center_axis',(1.,0.,0.));
#66462=DIRECTION('ref_axis',(0.,0.984807753012208,-0.17364817766693));
#66463=DIRECTION('center_axis',(-1.,0.,0.));
#66464=DIRECTION('ref_axis',(0.,1.,0.));
#66465=DIRECTION('center_axis',(0.,0.682250665052974,-0.731118342017744));
#66466=DIRECTION('ref_axis',(0.,0.731118342017744,0.682250665052974));
#66467=DIRECTION('',(1.,0.,0.));
#66468=DIRECTION('',(0.,-0.731118342017744,-0.682250665052974));
#66469=DIRECTION('',(1.,0.,0.));
#66470=DIRECTION('',(0.,0.731118342017744,0.682250665052974));
#66471=DIRECTION('center_axis',(1.,0.,0.));
#66472=DIRECTION('ref_axis',(0.,0.939692620785908,-0.342020143325669));
#66473=DIRECTION('center_axis',(1.,0.,0.));
#66474=DIRECTION('ref_axis',(0.,0.,-1.));
#66475=DIRECTION('',(0.,0.1215268689686,-0.992588142241629));
#66476=DIRECTION('center_axis',(0.,-0.992588142241629,-0.1215268689686));
#66477=DIRECTION('ref_axis',(0.,0.1215268689686,-0.992588142241629));
#66478=DIRECTION('',(-1.,0.,0.));
#66479=DIRECTION('',(0.,-0.1215268689686,0.992588142241629));
#66480=DIRECTION('center_axis',(1.,0.,0.));
#66481=DIRECTION('ref_axis',(0.,0.939692620785908,-0.342020143325669));
#66482=DIRECTION('center_axis',(-1.,0.,0.));
#66483=DIRECTION('ref_axis',(0.,1.,0.));
#66484=DIRECTION('center_axis',(0.,0.544928376691655,-0.838482596287006));
#66485=DIRECTION('ref_axis',(0.,0.838482596287006,0.544928376691655));
#66486=DIRECTION('',(1.,0.,0.));
#66487=DIRECTION('',(0.,-0.838482596287006,-0.544928376691655));
#66488=DIRECTION('',(1.,0.,0.));
#66489=DIRECTION('',(0.,0.838482596287006,0.544928376691655));
#66490=DIRECTION('center_axis',(1.,0.,0.));
#66491=DIRECTION('ref_axis',(0.,0.866025403784439,-0.5));
#66492=DIRECTION('center_axis',(1.,0.,0.));
#66493=DIRECTION('ref_axis',(0.,0.,-1.));
#66494=DIRECTION('',(0.,-0.0526805193144866,-0.998611417361506));
#66495=DIRECTION('center_axis',(0.,-0.998611417361506,0.0526805193144866));
#66496=DIRECTION('ref_axis',(0.,-0.0526805193144866,-0.998611417361506));
#66497=DIRECTION('',(-1.,0.,0.));
#66498=DIRECTION('',(0.,0.0526805193144866,0.998611417361506));
#66499=DIRECTION('center_axis',(1.,0.,0.));
#66500=DIRECTION('ref_axis',(0.,0.866025403784439,-0.5));
#66501=DIRECTION('center_axis',(-1.,0.,0.));
#66502=DIRECTION('ref_axis',(0.,1.,0.));
#66503=DIRECTION('center_axis',(0.,0.391048715351624,-0.920369981160753));
#66504=DIRECTION('ref_axis',(0.,0.920369981160753,0.391048715351624));
#66505=DIRECTION('',(1.,0.,0.));
#66506=DIRECTION('',(0.,-0.920369981160753,-0.391048715351624));
#66507=DIRECTION('',(1.,0.,0.));
#66508=DIRECTION('',(0.,0.920369981160753,0.391048715351624));
#66509=DIRECTION('center_axis',(1.,0.,0.));
#66510=DIRECTION('ref_axis',(0.,0.766044443118978,-0.642787609686539));
#66511=DIRECTION('center_axis',(1.,0.,0.));
#66512=DIRECTION('ref_axis',(0.,0.,-1.));
#66513=DIRECTION('',(0.,-0.225287236675832,-0.974292389886613));
#66514=DIRECTION('center_axis',(0.,-0.974292389886613,0.225287236675832));
#66515=DIRECTION('ref_axis',(0.,-0.225287236675832,-0.974292389886613));
#66516=DIRECTION('',(-1.,0.,0.));
#66517=DIRECTION('',(0.,0.225287236675832,0.974292389886613));
#66518=DIRECTION('center_axis',(1.,0.,0.));
#66519=DIRECTION('ref_axis',(0.,0.766044443118978,-0.642787609686539));
#66520=DIRECTION('center_axis',(-1.,0.,0.));
#66521=DIRECTION('ref_axis',(0.,1.,0.));
#66522=DIRECTION('center_axis',(0.,0.225287236675832,-0.974292389886613));
#66523=DIRECTION('ref_axis',(0.,0.974292389886613,0.225287236675832));
#66524=DIRECTION('',(1.,0.,0.));
#66525=DIRECTION('',(0.,-0.974292389886613,-0.225287236675832));
#66526=DIRECTION('',(1.,0.,0.));
#66527=DIRECTION('',(0.,0.974292389886613,0.225287236675832));
#66528=DIRECTION('center_axis',(1.,0.,0.));
#66529=DIRECTION('ref_axis',(0.,0.642787609686539,-0.766044443118978));
#66530=DIRECTION('center_axis',(1.,0.,0.));
#66531=DIRECTION('ref_axis',(0.,0.,-1.));
#66532=DIRECTION('',(0.,-0.391048715351624,-0.920369981160753));
#66533=DIRECTION('center_axis',(0.,-0.920369981160753,0.391048715351624));
#66534=DIRECTION('ref_axis',(0.,-0.391048715351624,-0.920369981160753));
#66535=DIRECTION('',(-1.,0.,0.));
#66536=DIRECTION('',(0.,0.391048715351624,0.920369981160753));
#66537=DIRECTION('center_axis',(1.,0.,0.));
#66538=DIRECTION('ref_axis',(0.,0.642787609686539,-0.766044443118978));
#66539=DIRECTION('center_axis',(-1.,0.,0.));
#66540=DIRECTION('ref_axis',(0.,1.,0.));
#66541=DIRECTION('center_axis',(0.,0.0526805193144864,-0.998611417361506));
#66542=DIRECTION('ref_axis',(0.,0.998611417361506,0.0526805193144864));
#66543=DIRECTION('',(1.,0.,0.));
#66544=DIRECTION('',(0.,-0.998611417361506,-0.0526805193144864));
#66545=DIRECTION('',(1.,0.,0.));
#66546=DIRECTION('',(0.,0.998611417361506,0.0526805193144864));
#66547=DIRECTION('center_axis',(1.,0.,0.));
#66548=DIRECTION('ref_axis',(0.,0.5,-0.866025403784439));
#66549=DIRECTION('center_axis',(1.,0.,0.));
#66550=DIRECTION('ref_axis',(0.,0.,-1.));
#66551=DIRECTION('',(0.,-0.544928376691655,-0.838482596287006));
#66552=DIRECTION('center_axis',(0.,-0.838482596287006,0.544928376691655));
#66553=DIRECTION('ref_axis',(0.,-0.544928376691655,-0.838482596287006));
#66554=DIRECTION('',(-1.,0.,0.));
#66555=DIRECTION('',(0.,0.544928376691655,0.838482596287006));
#66556=DIRECTION('center_axis',(1.,0.,0.));
#66557=DIRECTION('ref_axis',(0.,0.5,-0.866025403784439));
#66558=DIRECTION('center_axis',(-1.,0.,0.));
#66559=DIRECTION('ref_axis',(0.,1.,0.));
#66560=DIRECTION('center_axis',(0.,-0.1215268689686,-0.992588142241629));
#66561=DIRECTION('ref_axis',(0.,0.992588142241629,-0.1215268689686));
#66562=DIRECTION('',(1.,0.,0.));
#66563=DIRECTION('',(0.,-0.992588142241629,0.1215268689686));
#66564=DIRECTION('',(1.,0.,0.));
#66565=DIRECTION('',(0.,0.992588142241629,-0.1215268689686));
#66566=DIRECTION('center_axis',(1.,0.,0.));
#66567=DIRECTION('ref_axis',(0.,0.342020143325669,-0.939692620785908));
#66568=DIRECTION('center_axis',(1.,0.,0.));
#66569=DIRECTION('ref_axis',(0.,0.,-1.));
#66570=DIRECTION('',(0.,-0.682250665052974,-0.731118342017744));
#66571=DIRECTION('center_axis',(0.,-0.731118342017744,0.682250665052974));
#66572=DIRECTION('ref_axis',(0.,-0.682250665052974,-0.731118342017744));
#66573=DIRECTION('',(-1.,0.,0.));
#66574=DIRECTION('',(0.,0.682250665052974,0.731118342017744));
#66575=DIRECTION('center_axis',(1.,0.,0.));
#66576=DIRECTION('ref_axis',(0.,0.342020143325669,-0.939692620785908));
#66577=DIRECTION('center_axis',(-1.,0.,0.));
#66578=DIRECTION('ref_axis',(0.,1.,0.));
#66579=DIRECTION('center_axis',(0.,-0.292041724833639,-0.956405578693576));
#66580=DIRECTION('ref_axis',(0.,0.956405578693576,-0.292041724833639));
#66581=DIRECTION('',(1.,0.,0.));
#66582=DIRECTION('',(0.,-0.956405578693576,0.292041724833639));
#66583=DIRECTION('',(1.,0.,0.));
#66584=DIRECTION('',(0.,0.956405578693576,-0.292041724833639));
#66585=DIRECTION('center_axis',(1.,0.,0.));
#66586=DIRECTION('ref_axis',(0.,0.17364817766693,-0.984807753012208));
#66587=DIRECTION('center_axis',(1.,0.,0.));
#66588=DIRECTION('ref_axis',(0.,0.,-1.));
#66589=DIRECTION('',(0.,-0.798843112192153,-0.601539426890005));
#66590=DIRECTION('center_axis',(0.,-0.601539426890005,0.798843112192153));
#66591=DIRECTION('ref_axis',(0.,-0.798843112192153,-0.601539426890005));
#66592=DIRECTION('',(-1.,0.,0.));
#66593=DIRECTION('',(0.,0.798843112192153,0.601539426890005));
#66594=DIRECTION('center_axis',(1.,0.,0.));
#66595=DIRECTION('ref_axis',(0.,0.17364817766693,-0.984807753012208));
#66596=DIRECTION('center_axis',(-1.,0.,0.));
#66597=DIRECTION('ref_axis',(0.,1.,0.));
#66598=DIRECTION('center_axis',(1.,0.,0.));
#66599=DIRECTION('ref_axis',(0.,0.,-1.));
#66600=DIRECTION('center_axis',(1.,0.,0.));
#66601=DIRECTION('ref_axis',(0.,0.,-1.));
#66602=DIRECTION('',(0.,0.891163115601492,-0.453683040669851));
#66603=DIRECTION('',(0.,-0.891163115601492,-0.453683040669851));
#66604=DIRECTION('center_axis',(0.,-0.453683040669851,-0.891163115601492));
#66605=DIRECTION('ref_axis',(0.,0.891163115601492,-0.453683040669851));
#66606=DIRECTION('',(1.,0.,0.));
#66607=DIRECTION('',(0.,-0.891163115601492,0.453683040669851));
#66608=DIRECTION('',(1.,0.,0.));
#66609=DIRECTION('center_axis',(0.,-0.453683040669851,0.891163115601492));
#66610=DIRECTION('ref_axis',(0.,-0.891163115601492,-0.453683040669851));
#66611=DIRECTION('',(-1.,0.,0.));
#66612=DIRECTION('',(0.,0.891163115601492,0.453683040669851));
#66613=DIRECTION('center_axis',(1.,0.,0.));
#66614=DIRECTION('ref_axis',(0.,0.,-1.));
#66615=DIRECTION('center_axis',(-1.,0.,0.));
#66616=DIRECTION('ref_axis',(0.,1.,0.));
#66617=DIRECTION('center_axis',(1.,0.,0.));
#66618=DIRECTION('ref_axis',(0.,1.,0.));
#66619=DIRECTION('',(0.516609948219971,-0.856220860175784,-1.04856813577747E-16));
#66620=DIRECTION('center_axis',(-1.,0.,0.));
#66621=DIRECTION('ref_axis',(0.,1.,0.));
#66622=DIRECTION('center_axis',(0.,-0.5,0.866025403784439));
#66623=DIRECTION('ref_axis',(0.,-0.866025403784439,-0.5));
#66624=DIRECTION('',(0.,0.866025403784439,0.5));
#66625=DIRECTION('',(1.,0.,0.));
#66626=DIRECTION('',(0.,-0.866025403784439,-0.5));
#66627=DIRECTION('',(1.,0.,0.));
#66628=DIRECTION('center_axis',(0.,0.5,0.866025403784439));
#66629=DIRECTION('ref_axis',(0.,-0.866025403784439,0.5));
#66630=DIRECTION('',(0.,0.866025403784439,-0.5));
#66631=DIRECTION('',(0.,-0.866025403784439,0.5));
#66632=DIRECTION('',(1.,0.,0.));
#66633=DIRECTION('center_axis',(0.,1.,-3.60555503696918E-16));
#66634=DIRECTION('ref_axis',(0.,3.60555503696918E-16,1.));
#66635=DIRECTION('',(0.,-3.60555503696918E-16,-1.));
#66636=DIRECTION('',(0.,3.60555503696918E-16,1.));
#66637=DIRECTION('',(1.,0.,0.));
#66638=DIRECTION('center_axis',(0.,0.5,-0.866025403784439));
#66639=DIRECTION('ref_axis',(0.,0.866025403784439,0.5));
#66640=DIRECTION('',(0.,-0.866025403784439,-0.5));
#66641=DIRECTION('',(0.,0.866025403784439,0.5));
#66642=DIRECTION('',(1.,0.,0.));
#66643=DIRECTION('center_axis',(0.,-0.5,-0.866025403784439));
#66644=DIRECTION('ref_axis',(0.,0.866025403784439,-0.5));
#66645=DIRECTION('',(0.,-0.866025403784439,0.5));
#66646=DIRECTION('',(0.,0.866025403784439,-0.5));
#66647=DIRECTION('',(1.,0.,0.));
#66648=DIRECTION('center_axis',(0.,-1.,-1.20185167898973E-16));
#66649=DIRECTION('ref_axis',(0.,1.20185167898973E-16,-1.));
#66650=DIRECTION('',(0.,-1.20185167898973E-16,1.));
#66651=DIRECTION('',(0.,1.20185167898973E-16,-1.));
#66652=DIRECTION('center_axis',(1.,0.,0.));
#66653=DIRECTION('ref_axis',(0.,0.,-1.));
#66654=DIRECTION('center_axis',(-1.,0.,0.));
#66655=DIRECTION('ref_axis',(0.,0.,1.));
#66656=DIRECTION('center_axis',(1.,0.,0.));
#66657=DIRECTION('ref_axis',(0.,0.,-1.));
#66658=DIRECTION('center_axis',(1.,0.,0.));
#66659=DIRECTION('ref_axis',(0.,1.,0.));
#66660=DIRECTION('',(-0.707106781186548,0.707106781186547,8.65956056235493E-17));
#66661=DIRECTION('center_axis',(1.,0.,0.));
#66662=DIRECTION('ref_axis',(0.,1.,0.));
#66663=DIRECTION('center_axis',(1.,0.,0.));
#66664=DIRECTION('ref_axis',(0.,0.,-1.));
#66665=DIRECTION('center_axis',(1.,0.,0.));
#66666=DIRECTION('ref_axis',(0.,0.,-1.));
#66667=DIRECTION('center_axis',(1.,0.,0.));
#66668=DIRECTION('ref_axis',(0.,0.,-1.));
#66669=DIRECTION('center_axis',(1.,0.,0.));
#66670=DIRECTION('ref_axis',(0.,0.,-1.));
#66671=DIRECTION('center_axis',(1.,0.,0.));
#66672=DIRECTION('ref_axis',(0.,0.,-1.));
#66673=DIRECTION('center_axis',(1.,0.,0.));
#66674=DIRECTION('ref_axis',(0.,0.,-1.));
#66675=DIRECTION('center_axis',(1.,0.,0.));
#66676=DIRECTION('ref_axis',(0.,0.,-1.));
#66677=DIRECTION('center_axis',(1.,0.,0.));
#66678=DIRECTION('ref_axis',(0.,0.,-1.));
#66679=DIRECTION('center_axis',(1.,0.,0.));
#66680=DIRECTION('ref_axis',(0.,0.,-1.));
#66681=DIRECTION('center_axis',(1.,0.,0.));
#66682=DIRECTION('ref_axis',(0.,0.,-1.));
#66683=DIRECTION('center_axis',(1.,0.,0.));
#66684=DIRECTION('ref_axis',(0.,0.,-1.));
#66685=DIRECTION('center_axis',(1.,0.,0.));
#66686=DIRECTION('ref_axis',(0.,0.,-1.));
#66687=DIRECTION('center_axis',(1.,0.,0.));
#66688=DIRECTION('ref_axis',(0.,0.,-1.));
#66689=DIRECTION('center_axis',(1.,0.,0.));
#66690=DIRECTION('ref_axis',(0.,0.,-1.));
#66691=DIRECTION('center_axis',(1.,0.,0.));
#66692=DIRECTION('ref_axis',(0.,0.,-1.));
#66693=DIRECTION('center_axis',(1.,0.,0.));
#66694=DIRECTION('ref_axis',(0.,0.,-1.));
#66695=DIRECTION('center_axis',(1.,0.,0.));
#66696=DIRECTION('ref_axis',(0.,0.,-1.));
#66697=DIRECTION('',(-1.,0.,0.));
#66698=DIRECTION('center_axis',(1.,0.,0.));
#66699=DIRECTION('ref_axis',(0.,0.,-1.));
#66700=DIRECTION('center_axis',(1.,0.,0.));
#66701=DIRECTION('ref_axis',(0.,0.,-1.));
#66702=DIRECTION('center_axis',(1.,0.,0.));
#66703=DIRECTION('ref_axis',(0.,0.,-1.));
#66704=DIRECTION('center_axis',(1.,0.,0.));
#66705=DIRECTION('ref_axis',(0.,0.,-1.));
#66706=DIRECTION('center_axis',(1.,0.,0.));
#66707=DIRECTION('ref_axis',(0.,0.,-1.));
#66708=DIRECTION('center_axis',(1.,0.,0.));
#66709=DIRECTION('ref_axis',(0.,0.,-1.));
#66710=DIRECTION('center_axis',(1.,0.,0.));
#66711=DIRECTION('ref_axis',(0.,0.,-1.));
#66712=DIRECTION('center_axis',(1.,0.,0.));
#66713=DIRECTION('ref_axis',(0.,0.,-1.));
#66714=DIRECTION('center_axis',(1.,0.,0.));
#66715=DIRECTION('ref_axis',(0.,0.,-1.));
#66716=DIRECTION('center_axis',(1.,0.,0.));
#66717=DIRECTION('ref_axis',(0.,0.,-1.));
#66718=DIRECTION('center_axis',(1.,0.,0.));
#66719=DIRECTION('ref_axis',(0.,0.,-1.));
#66720=DIRECTION('center_axis',(1.,0.,0.));
#66721=DIRECTION('ref_axis',(0.,0.,-1.));
#66722=DIRECTION('center_axis',(1.,0.,0.));
#66723=DIRECTION('ref_axis',(0.,0.,-1.));
#66724=DIRECTION('center_axis',(1.,0.,0.));
#66725=DIRECTION('ref_axis',(0.,0.,-1.));
#66726=DIRECTION('center_axis',(1.,0.,0.));
#66727=DIRECTION('ref_axis',(0.,0.,-1.));
#66728=DIRECTION('center_axis',(1.,0.,0.));
#66729=DIRECTION('ref_axis',(0.,0.,-1.));
#66730=DIRECTION('center_axis',(1.,0.,0.));
#66731=DIRECTION('ref_axis',(0.,0.,-1.));
#66732=DIRECTION('center_axis',(1.,0.,0.));
#66733=DIRECTION('ref_axis',(0.,0.,-1.));
#66734=DIRECTION('center_axis',(1.,0.,0.));
#66735=DIRECTION('ref_axis',(0.,0.,-1.));
#66736=DIRECTION('center_axis',(-1.,0.,0.));
#66737=DIRECTION('ref_axis',(0.,1.,0.));
#66738=DIRECTION('center_axis',(1.,0.,0.));
#66739=DIRECTION('ref_axis',(0.,0.,-1.));
#66740=DIRECTION('',(-0.707106781186547,-0.707106781186548,-8.65956056235494E-17));
#66741=DIRECTION('center_axis',(1.,0.,0.));
#66742=DIRECTION('ref_axis',(0.,0.,-1.));
#84081=CARTESIAN_POINT('',(0.,0.,0.));
#84082=CARTESIAN_POINT('Origin',(-12.,0.,0.));
#84083=CARTESIAN_POINT('',(-23.5911584740964,-4.92956674790982,0.00292070512225823));
#84084=CARTESIAN_POINT('',(-23.8088415259036,-4.92702269843929,0.00145594308024882));
#84085=CARTESIAN_POINT('',(-12.,-4.925,-6.03138548580071E-16));
#84086=CARTESIAN_POINT('',(-24.075,2.17166274343819,4.42389655029935));
#84087=CARTESIAN_POINT('Ctrl Pts',(-23.5911584740964,-4.92956674790982,
0.00292070512225823));
#84088=CARTESIAN_POINT('Ctrl Pts',(-23.6009614954506,-4.93111317644749,
0.204570992366802));
#84089=CARTESIAN_POINT('Ctrl Pts',(-23.6107645168047,-4.91982886340447,
0.406056936676851));
#84090=CARTESIAN_POINT('Ctrl Pts',(-23.6205675381589,-4.89513422052396,
0.605891441984341));
#84091=CARTESIAN_POINT('Ctrl Pts',(-23.6995490603975,-4.69617306198144,
2.21592908800913));
#84092=CARTESIAN_POINT('Ctrl Pts',(-23.7785305826362,-3.62670832241862,
3.71876701687665));
#84093=CARTESIAN_POINT('Ctrl Pts',(-23.8575121048748,-2.16899469412727,
4.4312955762216));
#84094=CARTESIAN_POINT('Ctrl Pts',(-23.9300080699165,-0.830981026599293,
5.08531494765676));
#84095=CARTESIAN_POINT('Ctrl Pts',(-24.0025040349583,0.834137422466123,
5.07348830853079));
#84096=CARTESIAN_POINT('Ctrl Pts',(-24.075,2.1749296145658,4.42583829068189));
#84097=CARTESIAN_POINT('',(-24.075,-2.16839587231057,4.42195480991682));
#84098=CARTESIAN_POINT('Origin',(-24.075,0.,0.));
#84099=CARTESIAN_POINT('Ctrl Pts',(-24.075,-2.16839587231055,4.42195480991682));
#84100=CARTESIAN_POINT('Ctrl Pts',(-24.0355092388807,-2.89986906309508,
4.0632619883516));
#84101=CARTESIAN_POINT('Ctrl Pts',(-23.9960184777614,-3.53523507248361,
3.51964117664448));
#84102=CARTESIAN_POINT('Ctrl Pts',(-23.956527716642,-4.00941683121766,2.85617839596279));
#84103=CARTESIAN_POINT('Ctrl Pts',(-23.9170369555227,-4.48359858995173,
2.19271561528108));
#84104=CARTESIAN_POINT('Ctrl Pts',(-23.8775461944034,-4.79659609803131,
1.40941086562478));
#84105=CARTESIAN_POINT('Ctrl Pts',(-23.8380554332841,-4.89386793853736,
0.60185165851297));
#84106=CARTESIAN_POINT('Ctrl Pts',(-23.8283174641573,-4.91785405966823,
0.402716812689607));
#84107=CARTESIAN_POINT('Ctrl Pts',(-23.8185794950304,-4.92872278569346,
0.202107152556501));
#84108=CARTESIAN_POINT('Ctrl Pts',(-23.8088415259036,-4.92702269843929,
0.00145594308024882));
#84109=CARTESIAN_POINT('Origin',(-12.,0.,0.));
#84110=CARTESIAN_POINT('',(-22.0911584740964,-4.91737544826784,0.00117139545793843));
#84111=CARTESIAN_POINT('',(-22.3088415259036,-4.91734906814233,0.00115834211832263));
#84112=CARTESIAN_POINT('',(-12.,-4.925,-6.03138548580071E-16));
#84113=CARTESIAN_POINT('Ctrl Pts',(-22.0911584740964,-4.91737544826784,
0.00117139545793843));
#84114=CARTESIAN_POINT('Ctrl Pts',(-22.1270723620188,-4.91897685522205,
0.744760528145342));
#84115=CARTESIAN_POINT('Ctrl Pts',(-22.1629862499411,-4.76069723452924,
1.48770236188821));
#84116=CARTESIAN_POINT('Ctrl Pts',(-22.1989001378635,-4.43900651799258,
2.1514447222654));
#84117=CARTESIAN_POINT('Ctrl Pts',(-22.2778816601021,-3.7315469820872,3.61114137527611));
#84118=CARTESIAN_POINT('Ctrl Pts',(-22.3568631823407,-2.23375885028816,
4.68779421931301));
#84119=CARTESIAN_POINT('Ctrl Pts',(-22.4358447045794,-0.624704128296198,
4.8932036453613));
#84120=CARTESIAN_POINT('Ctrl Pts',(-22.514826226818,0.984350593695766,5.09861307140959));
#84121=CARTESIAN_POINT('Ctrl Pts',(-22.5938077490566,2.70467190588065,4.43277907946927));
#84122=CARTESIAN_POINT('Ctrl Pts',(-22.6727892712953,3.75614713958277,3.19766196357196));
#84123=CARTESIAN_POINT('Ctrl Pts',(-22.7517707935339,4.80762237328489,1.96254484767464));
#84124=CARTESIAN_POINT('Ctrl Pts',(-22.8307523157726,5.19025152850426,0.158144607820335));
#84125=CARTESIAN_POINT('Ctrl Pts',(-22.9097338380112,4.7307378850514,-1.39752590139163));
#84126=CARTESIAN_POINT('Ctrl Pts',(-22.9887153602498,4.27122424159855,-2.95319641060359));
#84127=CARTESIAN_POINT('Ctrl Pts',(-23.0676968824885,2.96956779947348,-4.26013718917321));
#84128=CARTESIAN_POINT('Ctrl Pts',(-23.1466784047271,1.41558592983439,-4.72553140556831));
#84129=CARTESIAN_POINT('Ctrl Pts',(-23.2256599269657,-0.138395939804694,
-5.19092562196341));
#84130=CARTESIAN_POINT('Ctrl Pts',(-23.3046414492044,-1.9447032369578,-4.81477327618398));
#84131=CARTESIAN_POINT('Ctrl Pts',(-23.383622971443,-3.18362809677325,-3.76807842170324));
#84132=CARTESIAN_POINT('Ctrl Pts',(-23.4528014723275,-4.26878019414078,
-2.85129714344818));
#84133=CARTESIAN_POINT('Ctrl Pts',(-23.5219799732119,-4.91865382585283,
-1.42009614555244));
#84134=CARTESIAN_POINT('Ctrl Pts',(-23.5911584740964,-4.92956674790982,
0.00292070512225823));
#84135=CARTESIAN_POINT('Ctrl Pts',(-23.8088415259036,-4.92702269843929,
0.00145594308024882));
#84136=CARTESIAN_POINT('Ctrl Pts',(-23.7395979727918,-4.91493392710047,
-1.42530999747258));
#84137=CARTESIAN_POINT('Ctrl Pts',(-23.67035441968,-4.26734424473369,-2.85417674458798));
#84138=CARTESIAN_POINT('Ctrl Pts',(-23.6011108665682,-3.18148423977708,
-3.76984525036356));
#84139=CARTESIAN_POINT('Ctrl Pts',(-23.5221293443296,-1.94291584928667,
-4.81428750097075));
#84140=CARTESIAN_POINT('Ctrl Pts',(-23.4431478220909,-0.134138057587843,
-5.19103575813942));
#84141=CARTESIAN_POINT('Ctrl Pts',(-23.3641662998523,1.41999380222758,-4.72488423722609));
#84142=CARTESIAN_POINT('Ctrl Pts',(-23.2851847776136,2.974125662043,-4.25873271631276));
#84143=CARTESIAN_POINT('Ctrl Pts',(-23.206203255375,4.27361158997502,-2.94968141731743));
#84144=CARTESIAN_POINT('Ctrl Pts',(-23.1272217331364,4.7315879300895,-1.39338320500447));
#84145=CARTESIAN_POINT('Ctrl Pts',(-23.0482402108977,5.18956427020398,0.162915007308491));
#84146=CARTESIAN_POINT('Ctrl Pts',(-22.9692586886591,4.80603102250092,1.96646013293908));
#84147=CARTESIAN_POINT('Ctrl Pts',(-22.8902771664205,3.75368351489473,3.20058718340981));
#84148=CARTESIAN_POINT('Ctrl Pts',(-22.8112956441818,2.70133600728855,4.43471423388053));
#84149=CARTESIAN_POINT('Ctrl Pts',(-22.7323141219432,0.980174239779238,
5.0994232091914));
#84150=CARTESIAN_POINT('Ctrl Pts',(-22.6533325997046,-0.628783080097548,
4.89276602692514));
#84151=CARTESIAN_POINT('Ctrl Pts',(-22.5743510774659,-2.23774039997434,
4.68610884465887));
#84152=CARTESIAN_POINT('Ctrl Pts',(-22.4953695552273,-3.73449327221861,
3.60808550481548));
#84153=CARTESIAN_POINT('Ctrl Pts',(-22.4163880329886,-4.44072222040884,
2.147775994752));
#84154=CARTESIAN_POINT('Ctrl Pts',(-22.3805391972936,-4.76127169589553,
1.48495772781659));
#84155=CARTESIAN_POINT('Ctrl Pts',(-22.3446903615986,-4.91896128463458,
0.743382726906644));
#84156=CARTESIAN_POINT('Ctrl Pts',(-22.3088415259036,-4.91734906814233,
0.00115834211832263));
#84157=CARTESIAN_POINT('Origin',(-12.,0.,0.));
#84158=CARTESIAN_POINT('',(-20.5911584740964,-4.92589392880443,-0.00432496190080733));
#84159=CARTESIAN_POINT('',(-20.8088415259036,-4.92585352153195,-0.00432860929833674));
#84160=CARTESIAN_POINT('',(-12.,-4.925,-6.03138548580071E-16));
#84161=CARTESIAN_POINT('Ctrl Pts',(-20.5911584740964,-4.92589392880443,
-0.00432496190080733));
#84162=CARTESIAN_POINT('Ctrl Pts',(-20.6531832285869,-4.91428084654241,
1.27427360734497));
#84163=CARTESIAN_POINT('Ctrl Pts',(-20.7152079830775,-4.40421217229855,
2.56109016084293));
#84164=CARTESIAN_POINT('Ctrl Pts',(-20.777232737568,-3.50886170650261,3.46719945285304));
#84165=CARTESIAN_POINT('Ctrl Pts',(-20.8562142598067,-2.36873397352748,
4.62102733633866));
#84166=CARTESIAN_POINT('Ctrl Pts',(-20.9351957820453,-0.603866149587261,
5.1575327966315));
#84167=CARTESIAN_POINT('Ctrl Pts',(-21.0141773042839,0.985531967041327,
4.83345759281197));
#84168=CARTESIAN_POINT('Ctrl Pts',(-21.0931588265226,2.57493008366992,4.50938238899243));
#84169=CARTESIAN_POINT('Ctrl Pts',(-21.1721403487612,3.98885849298689,3.3247265210605));
#84170=CARTESIAN_POINT('Ctrl Pts',(-21.2511218709998,4.58622424309187,1.81662748812464));
#84171=CARTESIAN_POINT('Ctrl Pts',(-21.3301033932385,5.18358999319685,0.308528455188798));
#84172=CARTESIAN_POINT('Ctrl Pts',(-21.4090849154771,4.96439308408986,-1.52301374275097));
#84173=CARTESIAN_POINT('Ctrl Pts',(-21.4880664377157,4.0280236561071,-2.84755980093255));
#84174=CARTESIAN_POINT('Ctrl Pts',(-21.5670479599544,3.09165422812432,-4.17210585911414));
#84175=CARTESIAN_POINT('Ctrl Pts',(-21.646029482193,1.43811228126576,-4.98965577753752));
#84176=CARTESIAN_POINT('Ctrl Pts',(-21.7250110044317,-0.18287507021828,
-4.92951859654145));
#84177=CARTESIAN_POINT('Ctrl Pts',(-21.8039925266703,-1.80386242170232,
-4.86938141554538));
#84178=CARTESIAN_POINT('Ctrl Pts',(-21.8829740489089,-3.39229517781185,
-3.93155713512985));
#84179=CARTESIAN_POINT('Ctrl Pts',(-21.9619555711476,-4.22794608586075,
-2.54127476392983));
#84180=CARTESIAN_POINT('Ctrl Pts',(-22.0050232054638,-4.68361605402348,
-1.78317120929954));
#84181=CARTESIAN_POINT('Ctrl Pts',(-22.0480908397801,-4.91545505442897,
-0.89053447936648));
#84182=CARTESIAN_POINT('Ctrl Pts',(-22.0911584740964,-4.91737544826784,
0.00117139545793843));
#84183=CARTESIAN_POINT('Ctrl Pts',(-22.3088415259036,-4.91734906814233,
0.00115834211832263));
#84184=CARTESIAN_POINT('Ctrl Pts',(-22.26570883936,-4.91540927770695,-0.891872940863008));
#84185=CARTESIAN_POINT('Ctrl Pts',(-22.2225761528164,-4.68285658280413,
-1.78584430297331));
#84186=CARTESIAN_POINT('Ctrl Pts',(-22.1794434662727,-4.22588839382535,
-2.54470959099318));
#84187=CARTESIAN_POINT('Ctrl Pts',(-22.1004619440341,-3.38912059491543,
-3.93428998639135));
#84188=CARTESIAN_POINT('Ctrl Pts',(-22.0214804217955,-1.79987997295941,
-4.87085509690416));
#84189=CARTESIAN_POINT('Ctrl Pts',(-21.9424988995568,-0.178834088830268,
-4.92967666338373));
#84190=CARTESIAN_POINT('Ctrl Pts',(-21.8635173773182,1.44221179529888,-4.98849822986331));
#84191=CARTESIAN_POINT('Ctrl Pts',(-21.7845358550796,3.09506294160113,-4.16957625230965));
#84192=CARTESIAN_POINT('Ctrl Pts',(-21.7055543328409,4.03034398306194,-2.84426032790294));
#84193=CARTESIAN_POINT('Ctrl Pts',(-21.6265728106023,4.96562502452275,-1.51894440349625));
#84194=CARTESIAN_POINT('Ctrl Pts',(-21.5475912883637,5.18333596114214,0.312765467763498));
#84195=CARTESIAN_POINT('Ctrl Pts',(-21.468609766125,4.5847403503353,1.82037297348421));
#84196=CARTESIAN_POINT('Ctrl Pts',(-21.3896282438864,3.98614473952846,3.32798047920493));
#84197=CARTESIAN_POINT('Ctrl Pts',(-21.3106467216477,2.57124258129539,4.51148561938661));
#84198=CARTESIAN_POINT('Ctrl Pts',(-21.2316651994091,0.981578778726861,
4.83426274757768));
#84199=CARTESIAN_POINT('Ctrl Pts',(-21.1526836771705,-0.608085023841661,
5.15703987576876));
#84200=CARTESIAN_POINT('Ctrl Pts',(-21.0737021549319,-2.37251047074563,
4.61908899196923));
#84201=CARTESIAN_POINT('Ctrl Pts',(-20.9947206326932,-3.51169377874649,
3.46432886221565));
#84202=CARTESIAN_POINT('Ctrl Pts',(-20.93276093043,-4.40536430555249,2.55843857551328));
#84203=CARTESIAN_POINT('Ctrl Pts',(-20.8708012281668,-4.91425182481639,
1.27295500491239));
#84204=CARTESIAN_POINT('Ctrl Pts',(-20.8088415259036,-4.92585352153195,
-0.00432860929833674));
#84205=CARTESIAN_POINT('Origin',(-12.,0.,0.));
#84206=CARTESIAN_POINT('',(-19.0911584740964,-4.93036753939865,0.00306120389312589));
#84207=CARTESIAN_POINT('',(-19.3088415259036,-4.93039896058852,0.00304429332654976));
#84208=CARTESIAN_POINT('',(-12.,-4.925,-6.03138548580071E-16));
#84209=CARTESIAN_POINT('Ctrl Pts',(-19.0911584740964,-4.93036753939865,
0.00306120389312589));
#84210=CARTESIAN_POINT('Ctrl Pts',(-19.1003125729165,-4.93174437091004,
0.191322718640612));
#84211=CARTESIAN_POINT('Ctrl Pts',(-19.1094666717366,-4.92188543239957,
0.379438718776696));
#84212=CARTESIAN_POINT('Ctrl Pts',(-19.1186207705567,-4.90030624508457,
0.56620051557689));
#84213=CARTESIAN_POINT('Ctrl Pts',(-19.1976022927953,-4.71412111683668,
2.17758043371112));
#84214=CARTESIAN_POINT('Ctrl Pts',(-19.2765838150339,-3.65545366284497,
3.68815033528921));
#84215=CARTESIAN_POINT('Ctrl Pts',(-19.3555653372726,-2.20431556954579,
4.41300092242343));
#84216=CARTESIAN_POINT('Ctrl Pts',(-19.4345468595112,-0.753177476246607,
5.13785150955766));
#84217=CARTESIAN_POINT('Ctrl Pts',(-19.5135283817499,1.09043125636005,5.07698278224803));
#84218=CARTESIAN_POINT('Ctrl Pts',(-19.5925099039885,2.49059780960012,4.25799328980927));
#84219=CARTESIAN_POINT('Ctrl Pts',(-19.6714914262271,3.89076436284019,3.43900379737051));
#84220=CARTESIAN_POINT('Ctrl Pts',(-19.7504729484657,4.84748873671366,1.86189353980263));
#84221=CARTESIAN_POINT('Ctrl Pts',(-19.8294544707044,4.92698134988234,0.241741989311494));
#84222=CARTESIAN_POINT('Ctrl Pts',(-19.908435992943,5.00647396305102,-1.37840956117965));
#84223=CARTESIAN_POINT('Ctrl Pts',(-19.9874175151817,4.20873481551489,-3.04160240459405));
#84224=CARTESIAN_POINT('Ctrl Pts',(-20.0663990374203,2.89546784338567,-3.99372633407541));
#84225=CARTESIAN_POINT('Ctrl Pts',(-20.1453805596589,1.58220087125645,-4.94585026355678));
#84226=CARTESIAN_POINT('Ctrl Pts',(-20.2243620818976,-0.246593925465854,
-5.18690527910513));
#84227=CARTESIAN_POINT('Ctrl Pts',(-20.3033436041362,-1.76172065737862,
-4.60759424510195));
#84228=CARTESIAN_POINT('Ctrl Pts',(-20.3823251263748,-3.27684738929139,
-4.02828321109877));
#84229=CARTESIAN_POINT('Ctrl Pts',(-20.4613066486135,-4.47830605639462,
-2.62860612754407));
#84230=CARTESIAN_POINT('Ctrl Pts',(-20.5402881708521,-4.82134156894121,
-1.04319243242752));
#84231=CARTESIAN_POINT('Ctrl Pts',(-20.5572449386002,-4.89498883922333,
-0.702815454993217));
#84232=CARTESIAN_POINT('Ctrl Pts',(-20.5742017063483,-4.92906879568418,
-0.353877316599127));
#84233=CARTESIAN_POINT('Ctrl Pts',(-20.5911584740964,-4.92589392880443,
-0.00432496190080733));
#84234=CARTESIAN_POINT('Ctrl Pts',(-20.8088415259036,-4.92585352153195,
-0.00432860929833674));
#84235=CARTESIAN_POINT('Ctrl Pts',(-20.7918197059282,-4.92904078657178,
-0.355229129225151));
#84236=CARTESIAN_POINT('Ctrl Pts',(-20.7747978859527,-4.89469624934525,
-0.705510771380119));
#84237=CARTESIAN_POINT('Ctrl Pts',(-20.7577760659773,-4.82048723932594,
-1.04713290262958));
#84238=CARTESIAN_POINT('Ctrl Pts',(-20.6787945437387,-4.4761562228068,-2.63226516201363));
#84239=CARTESIAN_POINT('Ctrl Pts',(-20.5998130215,-3.27355302067076,-4.03096030507408));
#84240=CARTESIAN_POINT('Ctrl Pts',(-20.5208314992614,-1.75795314101832,
-4.60903271986277));
#84241=CARTESIAN_POINT('Ctrl Pts',(-20.4418499770228,-0.242353261365892,
-5.18710513465145));
#84242=CARTESIAN_POINT('Ctrl Pts',(-20.3628684547841,1.58624329580292,-4.94455482116838));
#84243=CARTESIAN_POINT('Ctrl Pts',(-20.2838869325455,2.89873129214139,-3.99135762699838));
#84244=CARTESIAN_POINT('Ctrl Pts',(-20.2049054103069,4.21121928847986,-3.03816043282837));
#84245=CARTESIAN_POINT('Ctrl Pts',(-20.1259238880682,5.00759872398798,-1.37431635797142));
#84246=CARTESIAN_POINT('Ctrl Pts',(-20.0469423658296,4.92678177190102,0.24576949363086));
#84247=CARTESIAN_POINT('Ctrl Pts',(-19.9679608435909,4.84596481981407,1.86585534523313));
#84248=CARTESIAN_POINT('Ctrl Pts',(-19.8889793213523,3.88795148013202,3.44218297358073));
#84249=CARTESIAN_POINT('Ctrl Pts',(-19.8099977991137,2.48711597359967,4.26002756225397));
#84250=CARTESIAN_POINT('Ctrl Pts',(-19.731016276875,1.08628046706732,5.0778721509272));
#84251=CARTESIAN_POINT('Ctrl Pts',(-19.6520347546364,-0.757377206315341,
5.13723369992608));
#84252=CARTESIAN_POINT('Ctrl Pts',(-19.5730532323978,-2.20792214579921,
4.41119713404449));
#84253=CARTESIAN_POINT('Ctrl Pts',(-19.4940717101591,-3.65846708528308,
3.6851605681629));
#84254=CARTESIAN_POINT('Ctrl Pts',(-19.4150901879205,-4.71589929086815,
2.17372588740081));
#84255=CARTESIAN_POINT('Ctrl Pts',(-19.3361086656819,-4.90076709523542,
0.562194436802809));
#84256=CARTESIAN_POINT('Ctrl Pts',(-19.3270196190891,-4.92204133811868,
0.376742396565921));
#84257=CARTESIAN_POINT('Ctrl Pts',(-19.3179305724964,-4.93176022977169,
0.18996477700119));
#84258=CARTESIAN_POINT('Ctrl Pts',(-19.3088415259036,-4.93039896058852,
0.00304429332654976));
#84259=CARTESIAN_POINT('Origin',(-12.,0.,0.));
#84260=CARTESIAN_POINT('',(-17.5911584740964,-4.91748734336217,0.00138246325145752));
#84261=CARTESIAN_POINT('',(-17.8088415259036,-4.91749844770123,0.00140301643559147));
#84262=CARTESIAN_POINT('',(-12.,-4.925,-6.03138548580071E-16));
#84263=CARTESIAN_POINT('Ctrl Pts',(-17.5911584740964,-4.91748734336217,
0.00138246325145752));
#84264=CARTESIAN_POINT('Ctrl Pts',(-17.6264234394847,-4.9193418852286,0.731498546199545));
#84265=CARTESIAN_POINT('Ctrl Pts',(-17.661688404873,-4.76696687445272,1.46087872121623));
#84266=CARTESIAN_POINT('Ctrl Pts',(-17.6969533702612,-4.45641077730308,
2.11518020197493));
#84267=CARTESIAN_POINT('Ctrl Pts',(-17.7759348924999,-3.76087079808261,
3.58059286818176));
#84268=CARTESIAN_POINT('Ctrl Pts',(-17.8549164147385,-2.27188252680849,
4.66940512599426));
#84269=CARTESIAN_POINT('Ctrl Pts',(-17.9338979369771,-0.664569915601229,
4.88793730824473));
#84270=CARTESIAN_POINT('Ctrl Pts',(-18.0128794592158,0.942742695606023,
5.1064694904952));
#84271=CARTESIAN_POINT('Ctrl Pts',(-18.0918609814544,2.66837964674642,4.45472159718366));
#84272=CARTESIAN_POINT('Ctrl Pts',(-18.170842503693,3.72991782550763,3.22820341940916));
#84273=CARTESIAN_POINT('Ctrl Pts',(-18.2498240259317,4.79145600426884,2.00168524163466));
#84274=CARTESIAN_POINT('Ctrl Pts',(-18.3288055481703,5.18889541065087,0.200396779397185));
#84275=CARTESIAN_POINT('Ctrl Pts',(-18.407787070409,4.74203256755282,-1.3589376120088));
#84276=CARTESIAN_POINT('Ctrl Pts',(-18.4867685926476,4.29516972445477,-2.91827200341478));
#84277=CARTESIAN_POINT('Ctrl Pts',(-18.5657501148862,3.00400463187666,-4.23565232398927));
#84278=CARTESIAN_POINT('Ctrl Pts',(-18.6447316371249,1.45396599931439,-4.7137635888389));
#84279=CARTESIAN_POINT('Ctrl Pts',(-18.7237131593635,-0.096072633247862,
-5.19187485368853));
#84280=CARTESIAN_POINT('Ctrl Pts',(-18.8026946816021,-1.90498480579426,
-4.8307170628133));
#84281=CARTESIAN_POINT('Ctrl Pts',(-18.8816762038408,-3.15258949081541,
-3.79404320003051));
#84282=CARTESIAN_POINT('Ctrl Pts',(-18.9515036272593,-4.25559457517833,
-2.87752168067103));
#84283=CARTESIAN_POINT('Ctrl Pts',(-19.0213310506779,-4.91986507500412,
-1.43299675899955));
#84284=CARTESIAN_POINT('Ctrl Pts',(-19.0911584740964,-4.93036753939865,
0.00306120389312589));
#84285=CARTESIAN_POINT('Ctrl Pts',(-19.3088415259036,-4.93039896058852,
0.00304429332654976));
#84286=CARTESIAN_POINT('Ctrl Pts',(-19.2389490502577,-4.91993114394113,
-1.43432707666567));
#84287=CARTESIAN_POINT('Ctrl Pts',(-19.1690565746118,-4.2542688128935,-2.88014631871502));
#84288=CARTESIAN_POINT('Ctrl Pts',(-19.099164098966,-3.14948667556652,-3.79661879576485));
#84289=CARTESIAN_POINT('Ctrl Pts',(-19.0201825767273,-1.90103504838086,
-4.83227235730055));
#84290=CARTESIAN_POINT('Ctrl Pts',(-18.9412010544887,-0.0918283908600531,
-5.19195125993805));
#84291=CARTESIAN_POINT('Ctrl Pts',(-18.86221953225,1.45781876197131,-4.71257307881752));
#84292=CARTESIAN_POINT('Ctrl Pts',(-18.7832380100114,3.00746591480269,-4.23319489769699));
#84293=CARTESIAN_POINT('Ctrl Pts',(-18.7042564877728,4.29755356294462,-2.91475963281842));
#84294=CARTESIAN_POINT('Ctrl Pts',(-18.6252749655341,4.74314151432189,-1.35506058509819));
#84295=CARTESIAN_POINT('Ctrl Pts',(-18.5462934432955,5.18872946569916,0.204638462622037));
#84296=CARTESIAN_POINT('Ctrl Pts',(-18.4673119210569,4.78981772031176,2.00560129318392));
#84297=CARTESIAN_POINT('Ctrl Pts',(-18.3883303988182,3.72727733438716,3.23125119241768));
#84298=CARTESIAN_POINT('Ctrl Pts',(-18.3093488765796,2.66473694846256,4.45690109165143));
#84299=CARTESIAN_POINT('Ctrl Pts',(-18.230367354341,0.93856792200078,5.10723805955708));
#84300=CARTESIAN_POINT('Ctrl Pts',(-18.1513858321023,-0.668565385932749,
4.88739203645243));
#84301=CARTESIAN_POINT('Ctrl Pts',(-18.0724043098637,-2.27569869386628,
4.66754601334778));
#84302=CARTESIAN_POINT('Ctrl Pts',(-17.9934227876251,-3.76379628327154,
3.57751699923284));
#84303=CARTESIAN_POINT('Ctrl Pts',(-17.9144412653864,-4.45813804603734,
2.11153635114173));
#84304=CARTESIAN_POINT('Ctrl Pts',(-17.8792413522255,-4.76758725720248,
1.45818870670777));
#84305=CARTESIAN_POINT('Ctrl Pts',(-17.8440414390645,-4.91937734376141,
0.73016796568955));
#84306=CARTESIAN_POINT('Ctrl Pts',(-17.8088415259036,-4.91749844770123,
0.00140301643559147));
#84307=CARTESIAN_POINT('Origin',(-12.,0.,0.));
#84308=CARTESIAN_POINT('',(-16.0911584740964,-4.92549411112511,-0.00435654742202807));
#84309=CARTESIAN_POINT('',(-16.3088415259036,-4.92545367141813,-0.00435907189217228));
#84310=CARTESIAN_POINT('',(-12.,-4.925,-6.03138548580071E-16));
#84311=CARTESIAN_POINT('Ctrl Pts',(-16.0911584740964,-4.92549411112511,
-0.00435654742202807));
#84312=CARTESIAN_POINT('Ctrl Pts',(-16.1525343060529,-4.91401305180791,
1.26112872196585));
#84313=CARTESIAN_POINT('Ctrl Pts',(-16.2139101380093,-4.41566061870666,
2.53464705245624));
#84314=CARTESIAN_POINT('Ctrl Pts',(-16.2752859699658,-3.53701851325257,
3.43847122126015));
#84315=CARTESIAN_POINT('Ctrl Pts',(-16.3542674922044,-2.40633744906825,
4.60155783715884));
#84316=CARTESIAN_POINT('Ctrl Pts',(-16.4332490144431,-0.64590265744457,
5.15243672494805));
#84317=CARTESIAN_POINT('Ctrl Pts',(-16.5122305366817,0.946085018446281,
4.84133322963671));
#84318=CARTESIAN_POINT('Ctrl Pts',(-16.5912120589203,2.53807269433713,4.53022973432537));
#84319=CARTESIAN_POINT('Ctrl Pts',(-16.670193581159,3.96161325449515,3.3571438559135));
#84320=CARTESIAN_POINT('Ctrl Pts',(-16.7491751033976,4.57125747194857,1.85396586474963));
#84321=CARTESIAN_POINT('Ctrl Pts',(-16.8281566256362,5.18090168940199,0.350787873585757));
#84322=CARTESIAN_POINT('Ctrl Pts',(-16.9071381478749,4.97664956415081,-1.4824822303301));
#84323=CARTESIAN_POINT('Ctrl Pts',(-16.9861196701135,4.05111129643801,-2.81461925781151));
#84324=CARTESIAN_POINT('Ctrl Pts',(-17.0651011923521,3.12557302872522,-4.14675628529291));
#84325=CARTESIAN_POINT('Ctrl Pts',(-17.1440827145908,1.47874861855081,-4.97776023633987));
#84326=CARTESIAN_POINT('Ctrl Pts',(-17.2230642368294,-0.142673309742003,
-4.93084461620456));
#84327=CARTESIAN_POINT('Ctrl Pts',(-17.3020457590681,-1.76409523803482,
-4.88392899606925));
#84328=CARTESIAN_POINT('Ctrl Pts',(-17.3810272813067,-3.36011468444605,
-3.95909380475167));
#84329=CARTESIAN_POINT('Ctrl Pts',(-17.4600088035453,-4.20707856406823,
-2.57566967179231));
#84330=CARTESIAN_POINT('Ctrl Pts',(-17.5037253603957,-4.67587612005653,
-1.8099394346116));
#84331=CARTESIAN_POINT('Ctrl Pts',(-17.5474419172461,-4.91518834252542,
-0.903713030141044));
#84332=CARTESIAN_POINT('Ctrl Pts',(-17.5911584740964,-4.91748734336217,
0.00138246325145752));
#84333=CARTESIAN_POINT('Ctrl Pts',(-17.8088415259036,-4.91749844770123,
0.00140301643559147));
#84334=CARTESIAN_POINT('Ctrl Pts',(-17.7650599168259,-4.91516147907213,
-0.905033939016169));
#84335=CARTESIAN_POINT('Ctrl Pts',(-17.7212783077482,-4.67509315331331,
-1.81262221095911));
#84336=CARTESIAN_POINT('Ctrl Pts',(-17.6774966986705,-4.20497130464389,
-2.57910777670998));
#84337=CARTESIAN_POINT('Ctrl Pts',(-17.5985151764319,-3.35687686435833,
-3.96183897440324));
#84338=CARTESIAN_POINT('Ctrl Pts',(-17.5195336541932,-1.76010204766094,
-4.88536908772247));
#84339=CARTESIAN_POINT('Ctrl Pts',(-17.4405521319546,-0.138642432499522,
-4.93095922439053));
#84340=CARTESIAN_POINT('Ctrl Pts',(-17.361570609716,1.48281718266189,-4.9765493610586));
#84341=CARTESIAN_POINT('Ctrl Pts',(-17.2825890874773,3.1289615962873,-4.14419952107549));
#84342=CARTESIAN_POINT('Ctrl Pts',(-17.2036075652387,4.05341050192337,-2.81130644015036));
#84343=CARTESIAN_POINT('Ctrl Pts',(-17.1246260430001,4.97785940755944,-1.47841335922522));
#84344=CARTESIAN_POINT('Ctrl Pts',(-17.0456445207614,5.18061280520616,0.355022962641952));
#84345=CARTESIAN_POINT('Ctrl Pts',(-16.9666629985228,4.56974003457753,1.85770197110664));
#84346=CARTESIAN_POINT('Ctrl Pts',(-16.8876814762842,3.9588672639489,3.36038097957132));
#84347=CARTESIAN_POINT('Ctrl Pts',(-16.8086999540455,2.53436832504492,4.53230267463353));
#84348=CARTESIAN_POINT('Ctrl Pts',(-16.7297184318069,0.942126984447272,
4.8421046397495));
#84349=CARTESIAN_POINT('Ctrl Pts',(-16.6507369095683,-0.65011435615038,
5.15190660486548));
#84350=CARTESIAN_POINT('Ctrl Pts',(-16.5717553873296,-2.41009809844172,
4.59958884003522));
#84351=CARTESIAN_POINT('Ctrl Pts',(-16.492773865091,-3.53982791004914,3.43557840318775));
#84352=CARTESIAN_POINT('Ctrl Pts',(-16.4314630853618,-4.41680031662811,
2.53199506529855));
#84353=CARTESIAN_POINT('Ctrl Pts',(-16.3701523056327,-4.91398734347909,
1.25981119608574));
#84354=CARTESIAN_POINT('Ctrl Pts',(-16.3088415259036,-4.92545367141813,
-0.00435907189217227));
#84355=CARTESIAN_POINT('Origin',(-12.,0.,0.));
#84356=CARTESIAN_POINT('',(-14.5911584740964,-4.93067827447104,0.00288827060414214));
#84357=CARTESIAN_POINT('',(-14.8088415259036,-4.93070824935115,0.00287043364757822));
#84358=CARTESIAN_POINT('',(-12.,-4.925,-6.03138548580071E-16));
#84359=CARTESIAN_POINT('Ctrl Pts',(-14.5911584740964,-4.93067827447104,
0.00288827060414214));
#84360=CARTESIAN_POINT('Ctrl Pts',(-14.5996636503824,-4.93190134523225,
0.177775193398353));
#84361=CARTESIAN_POINT('Ctrl Pts',(-14.6081688266684,-4.92339421157364,
0.352541876964962));
#84362=CARTESIAN_POINT('Ctrl Pts',(-14.6166740029544,-4.90476040342235,
0.526222089557762));
#84363=CARTESIAN_POINT('Ctrl Pts',(-14.6956555251931,-4.731721481782,2.1390666811365));
#84364=CARTESIAN_POINT('Ctrl Pts',(-14.7746370474317,-3.68540719144605,
3.65821927729102));
#84365=CARTESIAN_POINT('Ctrl Pts',(-14.8536185696703,-2.24022814548496,
4.39487908351248));
#84366=CARTESIAN_POINT('Ctrl Pts',(-14.932600091909,-0.795049099523871,
5.13153888973394));
#84367=CARTESIAN_POINT('Ctrl Pts',(-15.0115816141476,1.04899470206234,5.08570590602234));
#84368=CARTESIAN_POINT('Ctrl Pts',(-15.0905631363863,2.45579315495828,4.27816132030787));
#84369=CARTESIAN_POINT('Ctrl Pts',(-15.1695446586249,3.86259160785421,3.47061673459341));
#84370=CARTESIAN_POINT('Ctrl Pts',(-15.2485261808635,4.83214471205985,1.90136054687609));
#84371=CARTESIAN_POINT('Ctrl Pts',(-15.3275077031022,4.92484623566303,0.281911081005368));
#84372=CARTESIAN_POINT('Ctrl Pts',(-15.4064892253408,5.0175477592662,-1.33753838486535));
#84373=CARTESIAN_POINT('Ctrl Pts',(-15.4854707475794,4.23339770226691,-3.00718112888947));
#84374=CARTESIAN_POINT('Ctrl Pts',(-15.5644522698181,2.9279384793258,-3.96998243872724));
#84375=CARTESIAN_POINT('Ctrl Pts',(-15.6434337920567,1.62247925638469,-4.93278374856501));
#84376=CARTESIAN_POINT('Ctrl Pts',(-15.7224153142953,-0.204289132498227,
-5.18874362421643));
#84377=CARTESIAN_POINT('Ctrl Pts',(-15.801396836534,-1.72408944853063,-4.62180699250664));
#84378=CARTESIAN_POINT('Ctrl Pts',(-15.8803783587726,-3.24388976456301,
-4.05487036079686));
#84379=CARTESIAN_POINT('Ctrl Pts',(-15.9593598810112,-4.45672200774489,
-2.66503722172589));
#84380=CARTESIAN_POINT('Ctrl Pts',(-16.0383414032499,-4.81267446096336,
-1.08247348018632));
#84381=CARTESIAN_POINT('Ctrl Pts',(-16.0559470935321,-4.89201945798192,
-0.729705816362758));
#84382=CARTESIAN_POINT('Ctrl Pts',(-16.0735527838142,-4.92878745914186,
-0.367361674999108));
#84383=CARTESIAN_POINT('Ctrl Pts',(-16.0911584740964,-4.92549411112511,
-0.00435654742202807));
#84384=CARTESIAN_POINT('Ctrl Pts',(-16.3088415259036,-4.92545367141813,
-0.00435907189217227));
#84385=CARTESIAN_POINT('Ctrl Pts',(-16.2911707833941,-4.92875844962247,
-0.3687130630225));
#84386=CARTESIAN_POINT('Ctrl Pts',(-16.2735000408846,-4.89171517974735,
-0.732401377008249));
#84387=CARTESIAN_POINT('Ctrl Pts',(-16.2558292983751,-4.81178759662622,
-1.08640725425502));
#84388=CARTESIAN_POINT('Ctrl Pts',(-16.1768477761364,-4.45454159067236,
-2.66867936598564));
#84389=CARTESIAN_POINT('Ctrl Pts',(-16.0978662538978,-3.24057369784111,
-4.05752048058219));
#84390=CARTESIAN_POINT('Ctrl Pts',(-16.0188847316592,-1.72031055150433,
-4.62321448816053));
#84391=CARTESIAN_POINT('Ctrl Pts',(-15.9399032094205,-0.200047405167556,
-5.18890849573887));
#84392=CARTESIAN_POINT('Ctrl Pts',(-15.8609216871819,1.62651099467473,-4.931455396299));
#84393=CARTESIAN_POINT('Ctrl Pts',(-15.7819401649433,2.93118262060901,-3.96758730739563));
#84394=CARTESIAN_POINT('Ctrl Pts',(-15.7029586427046,4.23585424654329,-3.00371921849225));
#84395=CARTESIAN_POINT('Ctrl Pts',(-15.623977120466,5.01863909856954,-1.33343614012536));
#84396=CARTESIAN_POINT('Ctrl Pts',(-15.5449955982273,4.92461376124743,0.285936880603985));
#84397=CARTESIAN_POINT('Ctrl Pts',(-15.4660140759887,4.83058842392532,1.90530990133333));
#84398=CARTESIAN_POINT('Ctrl Pts',(-15.3870325537501,3.85975289725486,3.47377286442513));
#84399=CARTESIAN_POINT('Ctrl Pts',(-15.3080510315114,2.45229487785007,4.28016710295635));
#84400=CARTESIAN_POINT('Ctrl Pts',(-15.2290695092728,1.04483685844527,5.08656134148757));
#84401=CARTESIAN_POINT('Ctrl Pts',(-15.1500879870342,-0.799243653693828,
5.13088685545821));
#84402=CARTESIAN_POINT('Ctrl Pts',(-15.0711064647955,-2.24381990927576,
4.39304596059483));
#84403=CARTESIAN_POINT('Ctrl Pts',(-14.9921249425569,-3.68839616485769,
3.65520506573145));
#84404=CARTESIAN_POINT('Ctrl Pts',(-14.9131434203183,-4.73346816388242,
2.13519776203403));
#84405=CARTESIAN_POINT('Ctrl Pts',(-14.8341618980796,-4.90518856206808,
0.522212377980333));
#84406=CARTESIAN_POINT('Ctrl Pts',(-14.825721774021,-4.92353894862701,0.349845521019683));
#84407=CARTESIAN_POINT('Ctrl Pts',(-14.8172816499623,-4.9319161064083,0.17641690191672));
#84408=CARTESIAN_POINT('Ctrl Pts',(-14.8088415259036,-4.93070824935115,
0.00287043364757822));
#84409=CARTESIAN_POINT('Origin',(-12.,0.,0.));
#84410=CARTESIAN_POINT('',(-13.0911584740964,-4.91760946231994,0.00158594389483818));
#84411=CARTESIAN_POINT('',(-13.3088415259036,-4.91762225934298,0.00160614365327011));
#84412=CARTESIAN_POINT('',(-12.,-4.925,-6.03138548580071E-16));
#84413=CARTESIAN_POINT('Ctrl Pts',(-13.0911584740964,-4.91760946231994,
0.00158594389483818));
#84414=CARTESIAN_POINT('Ctrl Pts',(-13.1257745169506,-4.91970084079515,
0.718222392324636));
#84415=CARTESIAN_POINT('Ctrl Pts',(-13.1603905598048,-4.77310485360014,
1.43404408902173));
#84416=CARTESIAN_POINT('Ctrl Pts',(-13.195006602659,-4.47351086752437,2.07877002591911));
#84417=CARTESIAN_POINT('Ctrl Pts',(-13.2739881248976,-3.78994373729305,
3.54980575745473));
#84418=CARTESIAN_POINT('Ctrl Pts',(-13.3529696471363,-2.30988370406987,
4.65072378465739));
#84419=CARTESIAN_POINT('Ctrl Pts',(-13.4319511693749,-0.704406556676555,
4.88235554885441));
#84420=CARTESIAN_POINT('Ctrl Pts',(-13.5109326916135,0.901070590716762,
5.11398731305142));
#84421=CARTESIAN_POINT('Ctrl Pts',(-13.5899142138522,2.63196485228022,4.47633281424283));
#84422=CARTESIAN_POINT('Ctrl Pts',(-13.6688957360908,3.70346939189113,3.25851174094001));
#84423=CARTESIAN_POINT('Ctrl Pts',(-13.7478772583294,4.77497393150204,2.04069066763719));
#84424=CARTESIAN_POINT('Ctrl Pts',(-13.8268587805681,5.18708874916036,0.242703019840158));
#84425=CARTESIAN_POINT('Ctrl Pts',(-13.9058403028067,4.75295637277905,-1.32022347387755));
#84426=CARTESIAN_POINT('Ctrl Pts',(-13.9848218250454,4.31882399639775,-2.88314996759526));
#84427=CARTESIAN_POINT('Ctrl Pts',(-14.063803347284,3.03844442597681,-4.21101530723365));
#84428=CARTESIAN_POINT('Ctrl Pts',(-14.1427848695226,1.49235609301499,-4.70175048191197));
#84429=CARTESIAN_POINT('Ctrl Pts',(-14.2217663917613,-0.0537322399468088,
-5.19248565659028));
#84430=CARTESIAN_POINT('Ctrl Pts',(-14.3007479139999,-1.86552933544948,
-4.84609066630856));
#84431=CARTESIAN_POINT('Ctrl Pts',(-14.3797294362385,-3.12154610672844,
-3.81962487766624));
#84432=CARTESIAN_POINT('Ctrl Pts',(-14.4502057821912,-4.24230789994266,
-2.90369472111239));
#84433=CARTESIAN_POINT('Ctrl Pts',(-14.5206821281438,-4.92054355707158,
-1.44627525745988));
#84434=CARTESIAN_POINT('Ctrl Pts',(-14.5911584740964,-4.93067827447104,
0.00288827060414214));
#84435=CARTESIAN_POINT('Ctrl Pts',(-14.8088415259036,-4.93070824935115,
0.00287043364757822));
#84436=CARTESIAN_POINT('Ctrl Pts',(-14.7383001277236,-4.92061314588811,
-1.44760712281891));
#84437=CARTESIAN_POINT('Ctrl Pts',(-14.6677587295437,-4.24096766997707,
-2.90631689952062));
#84438=CARTESIAN_POINT('Ctrl Pts',(-14.5972173313637,-3.11842239638253,
-3.82217508166485));
#84439=CARTESIAN_POINT('Ctrl Pts',(-14.5182358091251,-1.86156703516476,
-4.84761369284634));
#84440=CARTESIAN_POINT('Ctrl Pts',(-14.4392542868864,-0.0494875153826427,
-5.19252745079936));
#84441=CARTESIAN_POINT('Ctrl Pts',(-14.3602727646478,1.49619902186904,-4.70052859624512));
#84442=CARTESIAN_POINT('Ctrl Pts',(-14.2812912424092,3.04188555912074,-4.20852974169087));
#84443=CARTESIAN_POINT('Ctrl Pts',(-14.2023097201705,4.321179113842,-2.87961827462935));
#84444=CARTESIAN_POINT('Ctrl Pts',(-14.1233281979319,4.75403366621063,-1.31633753182672));
#84445=CARTESIAN_POINT('Ctrl Pts',(-14.0443466756933,5.18688821857927,0.246943210975917));
#84446=CARTESIAN_POINT('Ctrl Pts',(-13.9653651534546,4.77330376859529,2.04459322951967));
#84447=CARTESIAN_POINT('Ctrl Pts',(-13.886383631216,3.70080413609518,3.26153788011432));
#84448=CARTESIAN_POINT('Ctrl Pts',(-13.8074021089774,2.62830450359508,4.47848253070897));
#84449=CARTESIAN_POINT('Ctrl Pts',(-13.7284205867387,0.896889688578863,
5.11472181335452));
#84450=CARTESIAN_POINT('Ctrl Pts',(-13.6494390645001,-0.708397448067476,
4.88177771439169));
#84451=CARTESIAN_POINT('Ctrl Pts',(-13.5704575422615,-2.31368458471381,
4.64883361542886));
#84452=CARTESIAN_POINT('Ctrl Pts',(-13.4914760200228,-3.79284404299027,
3.54670613485765));
#84453=CARTESIAN_POINT('Ctrl Pts',(-13.4124944977842,-4.47520836483826,
2.07511221104824));
#84454=CARTESIAN_POINT('Ctrl Pts',(-13.3779435071573,-4.77371316216336,
1.43135369099267));
#84455=CARTESIAN_POINT('Ctrl Pts',(-13.3433925165305,-4.91973662561568,
0.71689100431942));
#84456=CARTESIAN_POINT('Ctrl Pts',(-13.3088415259036,-4.91762225934298,
0.00160614365327011));
#84457=CARTESIAN_POINT('Origin',(-12.,0.,0.));
#84458=CARTESIAN_POINT('',(-11.5911584740964,-4.92509485823308,-0.00437651270843276));
#84459=CARTESIAN_POINT('',(-11.8088415259036,-4.92505452712729,-0.00437787461885928));
#84460=CARTESIAN_POINT('',(-12.,-4.925,-6.03138548580071E-16));
#84461=CARTESIAN_POINT('Ctrl Pts',(-11.5911584740964,-4.92509485823308,
-0.00437651270843276));
#84462=CARTESIAN_POINT('Ctrl Pts',(-11.6518853835188,-4.91377256362929,
1.24798912490446));
#84463=CARTESIAN_POINT('Ctrl Pts',(-11.7126122929412,-4.42697102096967,
2.50818673560203));
#84464=CARTESIAN_POINT('Ctrl Pts',(-11.7733392023636,-3.56493996274647,
3.40951424172587));
#84465=CARTESIAN_POINT('Ctrl Pts',(-11.8523207246022,-2.44378089433587,
4.58178233747355));
#84466=CARTESIAN_POINT('Ctrl Pts',(-11.9313022468408,-0.687896782440381,
5.14699839364787));
#84467=CARTESIAN_POINT('Ctrl Pts',(-12.0102837690794,0.906574858907132,
4.84888712259997));
#84468=CARTESIAN_POINT('Ctrl Pts',(-12.0892652913181,2.50104650025465,4.55077585155208));
#84469=CARTESIAN_POINT('Ctrl Pts',(-12.1682468135567,3.93410567105417,3.38933725328197));
#84470=CARTESIAN_POINT('Ctrl Pts',(-12.2472283357954,4.55598729969703,1.89118059093196));
#84471=CARTESIAN_POINT('Ctrl Pts',(-12.326209858034,5.17786892833988,0.393023928581957));
#84472=CARTESIAN_POINT('Ctrl Pts',(-12.4051913802726,4.98857301482605,-1.44185079784797));
#84473=CARTESIAN_POINT('Ctrl Pts',(-12.4841729025113,4.07392844557266,-2.78149084536912));
#84474=CARTESIAN_POINT('Ctrl Pts',(-12.5631544247499,3.15928387631926,-4.12113089289029));
#84475=CARTESIAN_POINT('Ctrl Pts',(-12.6421359469885,1.51929065132632,-4.96553626150268));
#84476=CARTESIAN_POINT('Ctrl Pts',(-12.7211174692272,-0.102459940931512,
-4.93184410368197));
#84477=CARTESIAN_POINT('Ctrl Pts',(-12.8000989914658,-1.7242105331893,-4.89815194586127));
#84478=CARTESIAN_POINT('Ctrl Pts',(-12.8790805137045,-3.32771849271198,
-3.98636226160747));
#84479=CARTESIAN_POINT('Ctrl Pts',(-12.9580620359431,-4.18593535885357,
-2.6098907015463));
#84480=CARTESIAN_POINT('Ctrl Pts',(-13.0024275153275,-4.66801270559229,
-1.83669946782132));
#84481=CARTESIAN_POINT('Ctrl Pts',(-13.046792994712,-4.91492905748518,-0.916887600665788));
#84482=CARTESIAN_POINT('Ctrl Pts',(-13.0911584740964,-4.91760946231994,
0.00158594389483818));
#84483=CARTESIAN_POINT('Ctrl Pts',(-13.3088415259036,-4.91762225934298,
0.00160614365327011));
#84484=CARTESIAN_POINT('Ctrl Pts',(-13.2644109942918,-4.91490330929803,
-0.91820790615135));
#84485=CARTESIAN_POINT('Ctrl Pts',(-13.21998046268,-4.66721713029717,-1.83938153902219));
#84486=CARTESIAN_POINT('Ctrl Pts',(-13.1755499310683,-4.18380013351818,
-2.61331150839947));
#84487=CARTESIAN_POINT('Ctrl Pts',(-13.0965684088296,-3.32445839493059,
-3.98908093699027));
#84488=CARTESIAN_POINT('Ctrl Pts',(-13.017586886591,-1.72020573233587,-4.89955942712428));
#84489=CARTESIAN_POINT('Ctrl Pts',(-12.9386053643524,-0.0984282630900391,
-4.93192583826895));
#84490=CARTESIAN_POINT('Ctrl Pts',(-12.8596238421137,1.52334920615579,-4.96429224941362));
#84491=CARTESIAN_POINT('Ctrl Pts',(-12.7806423198751,3.16265148205274,-4.11854658156895));
#84492=CARTESIAN_POINT('Ctrl Pts',(-12.7016607976365,4.07620056018163,-2.77815938893629));
#84493=CARTESIAN_POINT('Ctrl Pts',(-12.6226792753978,4.98974963831051,-1.43777219630362));
#84494=CARTESIAN_POINT('Ctrl Pts',(-12.5436977531592,5.17754551867134,0.397256521117021));
#84495=CARTESIAN_POINT('Ctrl Pts',(-12.4647162309206,4.55443944667193,1.89490419909782));
#84496=CARTESIAN_POINT('Ctrl Pts',(-12.3857347086819,3.93133337467253,3.39255187707859));
#84497=CARTESIAN_POINT('Ctrl Pts',(-12.3067531864433,2.49732535031289,4.55281851561955));
#84498=CARTESIAN_POINT('Ctrl Pts',(-12.2277716642046,0.902610666028616,
4.84962623124001));
#84499=CARTESIAN_POINT('Ctrl Pts',(-12.148790141966,-0.692104018255692,
5.14643394686049));
#84500=CARTESIAN_POINT('Ctrl Pts',(-12.0698086197274,-2.44752536246463,
4.57978273956048));
#84501=CARTESIAN_POINT('Ctrl Pts',(-11.9908270974887,-3.5677256766153,3.40659861057621));
#84502=CARTESIAN_POINT('Ctrl Pts',(-11.9301652402937,-4.42809693258498,
2.505533069184));
#84503=CARTESIAN_POINT('Ctrl Pts',(-11.8695033830986,-4.9137495695897,1.2466721022382));
#84504=CARTESIAN_POINT('Ctrl Pts',(-11.8088415259036,-4.92505452712729,
-0.00437787461885928));
#84505=CARTESIAN_POINT('Origin',(-12.,0.,0.));
#84506=CARTESIAN_POINT('',(-10.0911584740964,-4.93097413974624,0.00270638408970972));
#84507=CARTESIAN_POINT('',(-10.3088415259036,-4.93100255652112,0.00268767346070769));
#84508=CARTESIAN_POINT('',(-12.,-4.925,-6.03138548580071E-16));
#84509=CARTESIAN_POINT('Ctrl Pts',(-10.0911584740964,-4.93097413974624,
0.00270638408970972));
#84510=CARTESIAN_POINT('Ctrl Pts',(-10.0990147278483,-4.93204740412384,
0.164224370369626));
#84511=CARTESIAN_POINT('Ctrl Pts',(-10.1068709816003,-4.92479171726874,
0.325644779964446));
#84512=CARTESIAN_POINT('Ctrl Pts',(-10.1147272353522,-4.90888841078112,
0.486208672297471));
#84513=CARTESIAN_POINT('Ctrl Pts',(-10.1937087575908,-4.74900720089645,
2.10041068682757));
#84514=CARTESIAN_POINT('Ctrl Pts',(-10.2726902798295,-3.71511564509976,
3.62804495438529));
#84515=CARTESIAN_POINT('Ctrl Pts',(-10.3516718020681,-2.27599174954493,
4.3764649956925));
#84516=CARTESIAN_POINT('Ctrl Pts',(-10.4306533243067,-0.836867853990087,
5.12488503699971));
#84517=CARTESIAN_POINT('Ctrl Pts',(-10.5096348465454,1.00748838132291,5.09409085205642));
#84518=CARTESIAN_POINT('Ctrl Pts',(-10.588616368784,2.42082519112922,4.29804486906693));
#84519=CARTESIAN_POINT('Ctrl Pts',(-10.6675978910227,3.83416200093553,3.50199888607743));
#84520=CARTESIAN_POINT('Ctrl Pts',(-10.7465794132613,4.81647938523517,1.94070110504172));
#84521=CARTESIAN_POINT('Ctrl Pts',(-10.8255609354999,4.92238364462085,0.322061419122964));
#84522=CARTESIAN_POINT('Ctrl Pts',(-10.9045424577385,5.02828790400653,-1.29657826679578));
#84523=CARTESIAN_POINT('Ctrl Pts',(-10.9835239799772,4.25777903847828,-2.97255985759757));
#84524=CARTESIAN_POINT('Ctrl Pts',(-11.0625055022158,2.96021439376647,-3.94597453684843));
#84525=CARTESIAN_POINT('Ctrl Pts',(-11.1414870244545,1.66264974905462,-4.91938921609932));
#84526=CARTESIAN_POINT('Ctrl Pts',(-11.2204685466931,-0.16197067484082,
-5.19023698379922));
#84527=CARTESIAN_POINT('Ctrl Pts',(-11.2994500689317,-1.68634355050059,
-4.63571242984327));
#84528=CARTESIAN_POINT('Ctrl Pts',(-11.3784315911704,-3.21071642616031,
-4.08118787588734));
#84529=CARTESIAN_POINT('Ctrl Pts',(-11.457413113409,-4.4348417535844,-2.70129100027559));
#84530=CARTESIAN_POINT('Ctrl Pts',(-11.5363946356476,-4.80368740483359,
-1.12168249480923));
#84531=CARTESIAN_POINT('Ctrl Pts',(-11.5546492484639,-4.88893689562171,
-0.756595309208631));
#84532=CARTESIAN_POINT('Ctrl Pts',(-11.5729038612802,-4.92849835935227,
-0.380839764938135));
#84533=CARTESIAN_POINT('Ctrl Pts',(-11.5911584740964,-4.92509485823308,
-0.00437651270843276));
#84534=CARTESIAN_POINT('Ctrl Pts',(-11.8088415259036,-4.92505452712729,
-0.00437787461885928));
#84535=CARTESIAN_POINT('Ctrl Pts',(-11.79052186086,-4.92846858408164,-0.382190516508843));
#84536=CARTESIAN_POINT('Ctrl Pts',(-11.7722021958164,-4.88862125463388,
-0.759290781644309));
#84537=CARTESIAN_POINT('Ctrl Pts',(-11.7538825307728,-4.80276849198252,
-1.12560890613918));
#84538=CARTESIAN_POINT('Ctrl Pts',(-11.6749010085342,-4.4326317091067,-2.70491524320179));
#84539=CARTESIAN_POINT('Ctrl Pts',(-11.5959194862956,-3.20737885926272,
-4.08381086665851));
#84540=CARTESIAN_POINT('Ctrl Pts',(-11.5169379640569,-1.68255330167799,
-4.6370890636446));
#84541=CARTESIAN_POINT('Ctrl Pts',(-11.4379564418183,-0.157727744093241,
-5.19036726063069));
#84542=CARTESIAN_POINT('Ctrl Pts',(-11.3589749195797,1.66667052123224,-4.91802803114613));
#84543=CARTESIAN_POINT('Ctrl Pts',(-11.279993397341,2.96343889606202,-3.94355303076636));
#84544=CARTESIAN_POINT('Ctrl Pts',(-11.2010118751024,4.26020727089178,-2.9690780303866));
#84545=CARTESIAN_POINT('Ctrl Pts',(-11.1220303528637,5.02934575522583,-1.29246725911162));
#84546=CARTESIAN_POINT('Ctrl Pts',(-11.0430488306251,4.9221183495091,0.326085189154109));
#84547=CARTESIAN_POINT('Ctrl Pts',(-10.9640673083865,4.81489094379237,1.94463763741987));
#84548=CARTESIAN_POINT('Ctrl Pts',(-10.8850857861478,3.83129764802485,3.50513176267639));
#84549=CARTESIAN_POINT('Ctrl Pts',(-10.8061042639092,2.4173106741576,4.30002205828802));
#84550=CARTESIAN_POINT('Ctrl Pts',(-10.7271227416706,1.00332370029034,5.09491235389966));
#84551=CARTESIAN_POINT('Ctrl Pts',(-10.6481412194319,-0.84105695167665,
5.12419881986638));
#84552=CARTESIAN_POINT('Ctrl Pts',(-10.5691596971933,-2.27956844569424,
4.37460264464728));
#84553=CARTESIAN_POINT('Ctrl Pts',(-10.4901781749547,-3.7180799397118,3.62500646942819));
#84554=CARTESIAN_POINT('Ctrl Pts',(-10.411196652716,-4.75072227577999,2.0965276530233));
#84555=CARTESIAN_POINT('Ctrl Pts',(-10.3322151304774,-4.9092838579553,0.482195602613046));
#84556=CARTESIAN_POINT('Ctrl Pts',(-10.3244239289528,-4.92492530428061,
0.322948401801202));
#84557=CARTESIAN_POINT('Ctrl Pts',(-10.3166327274282,-4.93206106288763,
0.162865762393093));
#84558=CARTESIAN_POINT('Ctrl Pts',(-10.3088415259036,-4.93100255652112,
0.00268767346070769));
#84559=CARTESIAN_POINT('Origin',(-12.,0.,0.));
#84560=CARTESIAN_POINT('',(-8.59115847409641,-4.91774836348285,0.00178568346280022));
#84561=CARTESIAN_POINT('',(-8.8088415259036,-4.91776282945141,0.0018054816820188));
#84562=CARTESIAN_POINT('',(-12.,-4.925,-6.03138548580071E-16));
#84563=CARTESIAN_POINT('Ctrl Pts',(-8.59115847409641,-4.91774836348285,
0.00178568346280023));
#84564=CARTESIAN_POINT('Ctrl Pts',(-8.62512559441653,-4.9200628213466,0.704938149616686));
#84565=CARTESIAN_POINT('Ctrl Pts',(-8.65909271473664,-4.77912254938096,
1.40720569299442));
#84566=CARTESIAN_POINT('Ctrl Pts',(-8.69305983505676,-4.49031348205501,
2.04222161760194));
#84567=CARTESIAN_POINT('Ctrl Pts',(-8.77204135729539,-3.81876465605063,
3.51878259476466));
#84568=CARTESIAN_POINT('Ctrl Pts',(-8.85102287953402,-2.34773128053141,
4.63173318336878));
#84569=CARTESIAN_POINT('Ctrl Pts',(-8.93000440177266,-0.744196356661722,
4.87644912669527));
#84570=CARTESIAN_POINT('Ctrl Pts',(-9.0089859240113,0.859338567207992,5.12116507002176));
#84571=CARTESIAN_POINT('Ctrl Pts',(-9.08796744624994,2.59537503942818,4.49764636807061));
#84572=CARTESIAN_POINT('Ctrl Pts',(-9.16694896848857,3.6767746879967,3.28860338080236));
#84573=CARTESIAN_POINT('Ctrl Pts',(-9.24593049072721,4.75817433656521,2.07956039353412));
#84574=CARTESIAN_POINT('Ctrl Pts',(-9.32491201296583,5.18493716148205,0.284993120948776));
#84575=CARTESIAN_POINT('Ctrl Pts',(-9.40389353520447,4.76356412017933,-1.28142154479291));
#84576=CARTESIAN_POINT('Ctrl Pts',(-9.48287505744311,4.34219107887662,-2.84783621053459));
#84577=CARTESIAN_POINT('Ctrl Pts',(-9.56185657968176,3.07268217135434,-4.18609826943261));
#84578=CARTESIAN_POINT('Ctrl Pts',(-9.64083810192039,1.53064694885267,-4.68942472169945));
#84579=CARTESIAN_POINT('Ctrl Pts',(-9.71981962415903,-0.0113882736489851,
-5.19275117396628));
#84580=CARTESIAN_POINT('Ctrl Pts',(-9.79880114639765,-1.82594981113003,
-4.86114201960195));
#84581=CARTESIAN_POINT('Ctrl Pts',(-9.87778266863628,-3.09029514788423,
-3.84495256166855));
#84582=CARTESIAN_POINT('Ctrl Pts',(-9.94890793712299,-4.22887666654442,
-2.92984297678998));
#84583=CARTESIAN_POINT('Ctrl Pts',(-10.0200332056097,-4.92125752169593,
-1.45956946675985));
#84584=CARTESIAN_POINT('Ctrl Pts',(-10.0911584740964,-4.93097413974624,
0.00270638408970972));
#84585=CARTESIAN_POINT('Ctrl Pts',(-10.3088415259036,-4.93100255652112,
0.00268767346070769));
#84586=CARTESIAN_POINT('Ctrl Pts',(-10.2376512051896,-4.92133069686354,
-1.46090295328149));
#84587=CARTESIAN_POINT('Ctrl Pts',(-10.1664608844755,-4.22752191947411,
-2.93246263442317));
#84588=CARTESIAN_POINT('Ctrl Pts',(-10.0952705637615,-3.0871507457315,-3.84747720854709));
#84589=CARTESIAN_POINT('Ctrl Pts',(-10.0162890415228,-1.82197522304997,
-4.86263268488127));
#84590=CARTESIAN_POINT('Ctrl Pts',(-9.93730751928421,-0.00714334940447398,
-5.19275835313399));
#84591=CARTESIAN_POINT('Ctrl Pts',(-9.85832599704557,1.53447978605512,-4.68817153945416));
#84592=CARTESIAN_POINT('Ctrl Pts',(-9.77934447480694,3.07610292151471,-4.18358472577433));
#84593=CARTESIAN_POINT('Ctrl Pts',(-9.70036295256829,4.34451731878839,-2.84428543016197));
#84594=CARTESIAN_POINT('Ctrl Pts',(-9.62138143032966,4.76460968983639,-1.27752694714326));
#84595=CARTESIAN_POINT('Ctrl Pts',(-9.54239990809102,5.18470206088438,0.289231535875453));
#84596=CARTESIAN_POINT('Ctrl Pts',(-9.46341838585239,4.75647240570669,2.08344920630051));
#84597=CARTESIAN_POINT('Ctrl Pts',(-9.38443686361376,3.67408484413261,3.29160768550489));
#84598=CARTESIAN_POINT('Ctrl Pts',(-9.30545534137512,2.59169728255855,4.49976616470925));
#84599=CARTESIAN_POINT('Ctrl Pts',(-9.22647381913649,0.855151814588114,
5.12186545269295));
#84600=CARTESIAN_POINT('Ctrl Pts',(-9.14749229689785,-0.748182403404063,
4.87583876767843));
#84601=CARTESIAN_POINT('Ctrl Pts',(-9.06851077465921,-2.35151662139626,
4.62981208266391));
#84602=CARTESIAN_POINT('Ctrl Pts',(-8.98952925242058,-3.8216395894102,3.51565942465113));
#84603=CARTESIAN_POINT('Ctrl Pts',(-8.91054773018194,-4.49198109523854,
2.03855008208786));
#84604=CARTESIAN_POINT('Ctrl Pts',(-8.87664566208916,-4.77971881833972,
1.40451492940035));
#84605=CARTESIAN_POINT('Ctrl Pts',(-8.84274359399638,-4.92009888102638,
0.703605948803637));
#84606=CARTESIAN_POINT('Ctrl Pts',(-8.8088415259036,-4.91776282945141,0.0018054816820188));
#84607=CARTESIAN_POINT('Origin',(-12.,0.,0.));
#84608=CARTESIAN_POINT('',(-7.0911584740964,-4.92469711254938,-0.00438490361534538));
#84609=CARTESIAN_POINT('',(-7.3088415259036,-4.92465698422042,-0.00438510844452123));
#84610=CARTESIAN_POINT('',(-12.,-4.925,-6.03138548580071E-16));
#84611=CARTESIAN_POINT('Ctrl Pts',(-7.0911584740964,-4.92469711254938,-0.00438490361534538));
#84612=CARTESIAN_POINT('Ctrl Pts',(-7.1512364609847,-4.91355887879697,1.23485426137012));
#84613=CARTESIAN_POINT('Ctrl Pts',(-7.21131444787301,-4.43814412276136,
2.4817098635007));
#84614=CARTESIAN_POINT('Ctrl Pts',(-7.27139243476131,-3.59262435392421,
3.38033053923436));
#84615=CARTESIAN_POINT('Ctrl Pts',(-7.35037395699995,-2.4810618351971,4.56170216236331));
#84616=CARTESIAN_POINT('Ctrl Pts',(-7.42935547923858,-0.729845164256781,
5.14121780162075));
#84617=CARTESIAN_POINT('Ctrl Pts',(-7.50833700147721,0.867004414740713,
4.85611857837648));
#84618=CARTESIAN_POINT('Ctrl Pts',(-7.58731852371585,2.46385399373825,4.5710193551322));
#84619=CARTESIAN_POINT('Ctrl Pts',(-7.66630004595449,3.90633648079293,3.42130526938617));
#84620=CARTESIAN_POINT('Ctrl Pts',(-7.74528156819313,4.54041416726393,1.9282695590024));
#84621=CARTESIAN_POINT('Ctrl Pts',(-7.82426309043176,5.17449185373491,0.435233848618645));
#84622=CARTESIAN_POINT('Ctrl Pts',(-7.9032446126704,5.00016473962219,-1.40112348640288));
#84623=CARTESIAN_POINT('Ctrl Pts',(-7.98222613490903,4.09647469008515,-2.74817747171883));
#84624=CARTESIAN_POINT('Ctrl Pts',(-8.06120765714767,3.19278464054811,-4.09523145703475));
#84625=CARTESIAN_POINT('Ctrl Pts',(-8.14018917938631,1.5597316555868,-4.95298209264516));
#84626=CARTESIAN_POINT('Ctrl Pts',(-8.21917070162494,-0.0622397588378364,
-4.93251563757504));
#84627=CARTESIAN_POINT('Ctrl Pts',(-8.29815222386358,-1.68421117326252,
-4.91204918250491));
#84628=CARTESIAN_POINT('Ctrl Pts',(-8.37713374610222,-3.29510101715048,
-4.0133656367542));
#84629=CARTESIAN_POINT('Ctrl Pts',(-8.45611526834085,-4.1645138008497,-2.64393818101814));
#84630=CARTESIAN_POINT('Ctrl Pts',(-8.50112967025937,-4.66002332471387,
-1.86345236429124));
#84631=CARTESIAN_POINT('Ctrl Pts',(-8.54614407217789,-4.91468116392279,
-0.930056269082769));
#84632=CARTESIAN_POINT('Ctrl Pts',(-8.59115847409641,-4.91774836348285,
0.00178568346280023));
#84633=CARTESIAN_POINT('Ctrl Pts',(-8.8088415259036,-4.91776282945141,0.0018054816820188));
#84634=CARTESIAN_POINT('Ctrl Pts',(-8.76376207175774,-4.91465659034033,
-0.931375995346603));
#84635=CARTESIAN_POINT('Ctrl Pts',(-8.71868261761189,-4.65921509964408,
-1.86613370276596));
#84636=CARTESIAN_POINT('Ctrl Pts',(-8.67360316346604,-4.16235075150242,
-2.64734146241595));
#84637=CARTESIAN_POINT('Ctrl Pts',(-8.5946216412274,-3.29181885829526,-4.0160576372427));
#84638=CARTESIAN_POINT('Ctrl Pts',(-8.51564011898876,-1.6801950282382,-4.91342395978241));
#84639=CARTESIAN_POINT('Ctrl Pts',(-8.43665859675013,-0.058207548536371,
-4.93256449308577));
#84640=CARTESIAN_POINT('Ctrl Pts',(-8.35767707451149,1.56377993116546,-4.95170502638914));
#84641=CARTESIAN_POINT('Ctrl Pts',(-8.27869555227285,3.19613106051205,-4.09261977045616));
#84642=CARTESIAN_POINT('Ctrl Pts',(-8.19971403003422,4.0987195627487,-2.74482759806664));
#84643=CARTESIAN_POINT('Ctrl Pts',(-8.12073250779558,5.00130806498535,-1.39703542567712));
#84644=CARTESIAN_POINT('Ctrl Pts',(-8.04175098555695,5.17413394011204,0.439463663168932));
#84645=CARTESIAN_POINT('Ctrl Pts',(-7.96276946331831,4.53883600150744,1.93198042137454));
#84646=CARTESIAN_POINT('Ctrl Pts',(-7.88378794107968,3.90353806290283,3.42449717958015));
#84647=CARTESIAN_POINT('Ctrl Pts',(-7.80480641884104,2.46011631056691,4.57303160714531));
#84648=CARTESIAN_POINT('Ctrl Pts',(-7.7258248966024,0.863034326582695,4.85682533639864));
#84649=CARTESIAN_POINT('Ctrl Pts',(-7.64684337436377,-0.734047657401497,
5.14061906565198));
#84650=CARTESIAN_POINT('Ctrl Pts',(-7.56786185212513,-2.48478987303398,
4.5596720965935));
#84651=CARTESIAN_POINT('Ctrl Pts',(-7.4888803298865,-3.59538619959974,3.37739228887328));
#84652=CARTESIAN_POINT('Ctrl Pts',(-7.42886739522553,-4.43925629594361,
2.47905456581291));
#84653=CARTESIAN_POINT('Ctrl Pts',(-7.36885446056456,-4.91353853831652,
1.2335376806911));
#84654=CARTESIAN_POINT('Ctrl Pts',(-7.3088415259036,-4.92465698422042,-0.00438510844452123));
#84655=CARTESIAN_POINT('Origin',(-12.,0.,0.));
#84656=CARTESIAN_POINT('',(-5.5911584740964,-4.93125390801305,0.00251598733971681));
#84657=CARTESIAN_POINT('',(-5.80884152590359,-4.93128064513841,0.00249645100189436));
#84658=CARTESIAN_POINT('',(-12.,-4.925,-6.03138548580071E-16));
#84659=CARTESIAN_POINT('Ctrl Pts',(-5.5911584740964,-4.93125390801305,0.00251598733971681));
#84660=CARTESIAN_POINT('Ctrl Pts',(-5.59836580531426,-4.93218240192545,
0.150670486559072));
#84661=CARTESIAN_POINT('Ctrl Pts',(-5.60557313653211,-4.92607803394608,
0.298747450142229));
#84662=CARTESIAN_POINT('Ctrl Pts',(-5.61278046774996,-4.91268998808522,
0.446162921385522));
#84663=CARTESIAN_POINT('Ctrl Pts',(-5.6917619899886,-4.76597711893443,2.06161501709073));
#84664=CARTESIAN_POINT('Ctrl Pts',(-5.77074351222723,-3.74457705430679,
3.59762937694339));
#84665=CARTESIAN_POINT('Ctrl Pts',(-5.84972503446586,-2.31160400818357,
4.35775988654768));
#84666=CARTESIAN_POINT('Ctrl Pts',(-5.9287065567045,-0.878630962060319,
5.11789039615198));
#84667=CARTESIAN_POINT('Ctrl Pts',(-6.00768807894314,0.965915065558466,
5.10213705550793));
#84668=CARTESIAN_POINT('Ctrl Pts',(-6.08666960118177,2.38569625012759,4.31764260950633));
#84669=CARTESIAN_POINT('Ctrl Pts',(-6.16565112342041,3.80547743469666,3.53314816350476));
#84670=CARTESIAN_POINT('Ctrl Pts',(-6.24463264565905,4.80049377621606,1.9799126121456));
#84671=CARTESIAN_POINT('Ctrl Pts',(-6.32361416789768,4.91959372867696,0.362190341378671));
#84672=CARTESIAN_POINT('Ctrl Pts',(-6.40259569013632,5.03869368113786,-1.25553192938831));
#84673=CARTESIAN_POINT('Ctrl Pts',(-6.48157721237495,4.2818772445403,-2.93774091956309));
#84674=CARTESIAN_POINT('Ctrl Pts',(-6.56055873461359,2.99229346260409,-3.92170423906757));
#84675=CARTESIAN_POINT('Ctrl Pts',(-6.63954025685222,1.70270968066789,-4.90566755857204));
#84676=CARTESIAN_POINT('Ctrl Pts',(-6.71852177909086,-0.119641446606939,
-5.19138520740618));
#84677=CARTESIAN_POINT('Ctrl Pts',(-6.7975033013295,-1.64848551554391,-4.64930960543246));
#84678=CARTESIAN_POINT('Ctrl Pts',(-6.87648482356814,-3.17732958448089,
-4.10723400345873));
#84679=CARTESIAN_POINT('Ctrl Pts',(-6.95546634580677,-4.41266659508003,
-2.73736515067713));
#84680=CARTESIAN_POINT('Ctrl Pts',(-7.0344478680454,-4.79438091712263,-1.16081692078609));
#84681=CARTESIAN_POINT('Ctrl Pts',(-7.05335140339573,-4.88574089570925,
-0.783483914906529));
#84682=CARTESIAN_POINT('Ctrl Pts',(-7.07225493874606,-4.92820175720184,
-0.394311440374502));
#84683=CARTESIAN_POINT('Ctrl Pts',(-7.0911584740964,-4.92469711254938,-0.00438490361534538));
#84684=CARTESIAN_POINT('Ctrl Pts',(-7.3088415259036,-4.92465698422042,-0.00438510844452123));
#84685=CARTESIAN_POINT('Ctrl Pts',(-7.28987293832593,-4.92817124687141,
-0.395661538646872));
#84686=CARTESIAN_POINT('Ctrl Pts',(-7.27090435074826,-4.88541387252908,
-0.786179292857178));
#84687=CARTESIAN_POINT('Ctrl Pts',(-7.25193576317059,-4.79343001691259,
-1.16473570824833));
#84688=CARTESIAN_POINT('Ctrl Pts',(-7.17295424093195,-4.41042707016064,
-2.74097125126758));
#84689=CARTESIAN_POINT('Ctrl Pts',(-7.09397271869331,-3.17397073915778,
-4.10982969092408));
#84690=CARTESIAN_POINT('Ctrl Pts',(-7.01499119645468,-1.64468416686737,
-4.65065528590648));
#84691=CARTESIAN_POINT('Ctrl Pts',(-6.93600967421605,-0.11539759457693,
-5.19148088088889));
#84692=CARTESIAN_POINT('Ctrl Pts',(-6.85702815197741,1.70671921900106,-4.90427363119719));
#84693=CARTESIAN_POINT('Ctrl Pts',(-6.77804662973878,2.9954981113016,-3.91925651912733));
#84694=CARTESIAN_POINT('Ctrl Pts',(-6.69906510750014,4.28427700360214,-2.93423940705747));
#84695=CARTESIAN_POINT('Ctrl Pts',(-6.6200835852615,5.03971797462523,-1.25141243260946));
#84696=CARTESIAN_POINT('Ctrl Pts',(-6.54110206302287,4.91929563087673,0.366211814021057));
#84697=CARTESIAN_POINT('Ctrl Pts',(-6.46212054078423,4.79887328712824,1.98383606065158));
#84698=CARTESIAN_POINT('Ctrl Pts',(-6.3831390185456,3.80258762860816,3.5362575794646));
#84699=CARTESIAN_POINT('Ctrl Pts',(-6.30415749630696,2.38216572629362,4.31959107430742));
#84700=CARTESIAN_POINT('Ctrl Pts',(-6.22517597406833,0.96174382397912,5.10292456915022));
#84701=CARTESIAN_POINT('Ctrl Pts',(-6.14619445182969,-0.882814322129821,
5.11717004002285));
#84702=CARTESIAN_POINT('Ctrl Pts',(-6.06721292959106,-2.31516539749777,
4.35586843028431));
#84703=CARTESIAN_POINT('Ctrl Pts',(-5.98823140735242,-3.74751647286578,
3.59456682054574));
#84704=CARTESIAN_POINT('Ctrl Pts',(-5.90924988511379,-4.76766047749277,
2.05771813019591));
#84705=CARTESIAN_POINT('Ctrl Pts',(-5.83026836287515,-4.91305270009236,
0.442146762242162));
#84706=CARTESIAN_POINT('Ctrl Pts',(-5.82312608388463,-4.92620048184465,
0.296051053879439));
#84707=CARTESIAN_POINT('Ctrl Pts',(-5.81598380489411,-4.93219494682612,
0.149311587754206));
#84708=CARTESIAN_POINT('Ctrl Pts',(-5.80884152590359,-4.93128064513841,
0.00249645100189436));
#84709=CARTESIAN_POINT('Origin',(-12.,0.,0.));
#84710=CARTESIAN_POINT('',(-4.0911584740964,-4.91790394892889,0.00198131612508923));
#84711=CARTESIAN_POINT('',(-4.30884152590359,-4.91791992129793,0.00200057189650126));
#84712=CARTESIAN_POINT('',(-12.,-4.925,-6.03138548580071E-16));
#84713=CARTESIAN_POINT('Ctrl Pts',(-4.0911584740964,-4.91790394892889,0.00198131612508923));
#84714=CARTESIAN_POINT('Ctrl Pts',(-4.12447667188244,-4.92042735435566,
0.691645796992671));
#84715=CARTESIAN_POINT('Ctrl Pts',(-4.15779486966848,-4.78502020932576,
1.38036363987776));
#84716=CARTESIAN_POINT('Ctrl Pts',(-4.19111306745451,-4.5068173542973,2.00553729863833));
#84717=CARTESIAN_POINT('Ctrl Pts',(-4.27009458969315,-3.8473313544126,3.48752523656628));
#84718=CARTESIAN_POINT('Ctrl Pts',(-4.34907611193179,-2.38542274738594,
4.61243459072995));
#84719=CARTESIAN_POINT('Ctrl Pts',(-4.42805763417042,-0.783936747380577,
4.87021849115426));
#84720=CARTESIAN_POINT('Ctrl Pts',(-4.50703915640906,0.817549252624831,
5.12800239157858));
#84721=CARTESIAN_POINT('Ctrl Pts',(-4.58602067864769,2.55861264560894,4.51866083826349));
#84722=CARTESIAN_POINT('Ctrl Pts',(-4.66500220088633,3.64983552948727,3.31847630846199));
#84723=CARTESIAN_POINT('Ctrl Pts',(-4.74398372312497,4.7410584133656,2.11829177866049));
#84724=CARTESIAN_POINT('Ctrl Pts',(-4.82296524536361,5.18244078813814,0.327264272372587));
#84725=CARTESIAN_POINT('Ctrl Pts',(-4.90194676760224,4.77385508310388,-1.2425343895004));
#84726=CARTESIAN_POINT('Ctrl Pts',(-4.98092828984088,4.36526937806963,-2.81233305137334));
#84727=CARTESIAN_POINT('Ctrl Pts',(-5.05990981207951,3.10671559322865,-4.16090286883138));
#84728=CARTESIAN_POINT('Ctrl Pts',(-5.13889133431815,1.56883603197956,-4.6767871360847));
#84729=CARTESIAN_POINT('Ctrl Pts',(-5.21787285655678,0.0309564707304835,
-5.19267140333802));
#84730=CARTESIAN_POINT('Ctrl Pts',(-5.29685437879541,-1.78624886692669,
-4.87587012038662));
#84731=CARTESIAN_POINT('Ctrl Pts',(-5.37583590103405,-3.05883869891831,
-3.87002456313205));
#84732=CARTESIAN_POINT('Ctrl Pts',(-5.44761009205483,-4.21530040165052,
-2.95596581726907));
#84733=CARTESIAN_POINT('Ctrl Pts',(-5.51938428307562,-4.92200750356521,
-1.47288024548768));
#84734=CARTESIAN_POINT('Ctrl Pts',(-5.5911584740964,-4.93125390801305,0.00251598733971681));
#84735=CARTESIAN_POINT('Ctrl Pts',(-5.80884152590359,-4.93128064513841,
0.00249645100189436));
#84736=CARTESIAN_POINT('Ctrl Pts',(-5.73700228265547,-4.92208431698711,
-1.47421544105046));
#84737=CARTESIAN_POINT('Ctrl Pts',(-5.66516303940736,-4.21393107993154,
-2.95858289742135));
#84738=CARTESIAN_POINT('Ctrl Pts',(-5.59332379615924,-3.05567380905537,
-3.8725234884491));
#84739=CARTESIAN_POINT('Ctrl Pts',(-5.5143422739206,-1.78226225484658,-4.87732832562897));
#84740=CARTESIAN_POINT('Ctrl Pts',(-5.43536075168197,0.0352012941432209,
-5.19264395443107));
#84741=CARTESIAN_POINT('Ctrl Pts',(-5.35637922944334,1.57265851305555,-4.67550273398319));
#84742=CARTESIAN_POINT('Ctrl Pts',(-5.2773977072047,3.11011573196789,-4.1583615135353));
#84743=CARTESIAN_POINT('Ctrl Pts',(-5.19841618496606,4.36756662080275,-2.80876344383742));
#84744=CARTESIAN_POINT('Ctrl Pts',(-5.11943466272742,4.77486887790956,-1.23863140793454));
#84745=CARTESIAN_POINT('Ctrl Pts',(-5.04045314048879,5.18217113501637,0.331500627968312));
#84746=CARTESIAN_POINT('Ctrl Pts',(-4.96147161825015,4.73932476039516,2.12216663007616));
#84747=CARTESIAN_POINT('Ctrl Pts',(-4.88249009601152,3.64712124096917,3.32145860332436));
#84748=CARTESIAN_POINT('Ctrl Pts',(-4.80350857377289,2.55491772154319,4.52075057657256));
#84749=CARTESIAN_POINT('Ctrl Pts',(-4.72452705153425,0.813357057312425,
5.12866852096113));
#84750=CARTESIAN_POINT('Ctrl Pts',(-4.64554552929562,-0.787917616290547,
4.86957560126685));
#84751=CARTESIAN_POINT('Ctrl Pts',(-4.56656400705698,-2.38919228989357,
4.61048268157256));
#84752=CARTESIAN_POINT('Ctrl Pts',(-4.48758248481834,-3.85018097286878,
3.48437889779535));
#84753=CARTESIAN_POINT('Ctrl Pts',(-4.4086009625797,-4.50845510335787,2.00185237675489));
#84754=CARTESIAN_POINT('Ctrl Pts',(-4.375347817021,-4.78560455373875,1.3776725837921));
#84755=CARTESIAN_POINT('Ctrl Pts',(-4.34209467146229,-4.92046360302658,
0.690312754928868));
#84756=CARTESIAN_POINT('Ctrl Pts',(-4.30884152590359,-4.91791992129793,
0.00200057189650126));
#84757=CARTESIAN_POINT('Origin',(-12.,0.,0.));
#84758=CARTESIAN_POINT('',(-2.5911584740964,-4.92431925468094,-0.00436907230553341));
#84759=CARTESIAN_POINT('',(-2.8088415259036,-4.92426410821032,-0.00437867314108101));
#84760=CARTESIAN_POINT('',(-12.,-4.925,-6.03138548580071E-16));
#84761=CARTESIAN_POINT('Ctrl Pts',(-2.5911584740964,-4.92431925468094,-0.00436907230553341));
#84762=CARTESIAN_POINT('Ctrl Pts',(-2.65058753845062,-4.91338616368288,
1.22173429077995));
#84763=CARTESIAN_POINT('Ctrl Pts',(-2.71001660280484,-4.44917797193856,
2.45521514120874));
#84764=CARTESIAN_POINT('Ctrl Pts',(-2.76944566715907,-3.62006233571212,
3.35091658286247));
#84765=CARTESIAN_POINT('Ctrl Pts',(-2.8484271893977,-2.51816352958756,4.54130825572287));
#84766=CARTESIAN_POINT('Ctrl Pts',(-2.92740871163635,-0.77174540757938,
5.13509562040796));
#84767=CARTESIAN_POINT('Ctrl Pts',(-3.00639023387498,0.827372408670279,
4.86302996372663));
#84768=CARTESIAN_POINT('Ctrl Pts',(-3.08537175611362,2.42649022491994,4.5909643070453));
#84769=CARTESIAN_POINT('Ctrl Pts',(-3.16435327835225,3.87830773541108,3.45304562899755));
#84770=CARTESIAN_POINT('Ctrl Pts',(-3.24333480059088,4.52454114442089,1.9652288206206));
#84771=CARTESIAN_POINT('Ctrl Pts',(-3.32231632282952,5.1707745534307,0.47741201224366));
#84772=CARTESIAN_POINT('Ctrl Pts',(-3.40129784506816,5.01142386095919,-1.36030292646248));
#84773=CARTESIAN_POINT('Ctrl Pts',(-3.4802793673068,4.11874747202576,-2.71468058079156));
#84774=CARTESIAN_POINT('Ctrl Pts',(-3.55926088954543,3.22607108309233,-4.06905823512064));
#84775=CARTESIAN_POINT('Ctrl Pts',(-3.63824241178406,1.60006899769698,-4.94009860507265));
#84776=CARTESIAN_POINT('Ctrl Pts',(-3.7172239340227,-0.0220148869955472,
-4.9328595746569));
#84777=CARTESIAN_POINT('Ctrl Pts',(-3.79620545626133,-1.64409877168807,
-4.92562054424115));
#84778=CARTESIAN_POINT('Ctrl Pts',(-3.87518697849998,-3.26226445567777,
-4.04010211345763));
#84779=CARTESIAN_POINT('Ctrl Pts',(-3.95416850073861,-4.14281560130125,
-2.67780963721974));
#84780=CARTESIAN_POINT('Ctrl Pts',(-3.99983182519121,-4.65190800063768,
-1.89019752772115));
#84781=CARTESIAN_POINT('Ctrl Pts',(-4.0454951496438,-4.91444556617158,-0.943219056221707));
#84782=CARTESIAN_POINT('Ctrl Pts',(-4.0911584740964,-4.91790394892889,0.00198131612508923));
#84783=CARTESIAN_POINT('Ctrl Pts',(-4.30884152590359,-4.91791992129793,
0.00200057189650126));
#84784=CARTESIAN_POINT('Ctrl Pts',(-4.26311314922366,-4.9144219533828,-0.944538417130053));
#84785=CARTESIAN_POINT('Ctrl Pts',(-4.21738477254373,-4.65108670196389,
-1.89287836832389));
#84786=CARTESIAN_POINT('Ctrl Pts',(-4.1716563958638,-4.14062462025537,-2.68119534003646));
#84787=CARTESIAN_POINT('Ctrl Pts',(-4.09267487362516,-3.25896042866083,
-4.04276727748366));
#84788=CARTESIAN_POINT('Ctrl Pts',(-4.01369335138653,-1.64007246746879,
-4.92696189407442));
#84789=CARTESIAN_POINT('Ctrl Pts',(-3.93471182914789,-0.017982895669106,
-4.93287521506465));
#84790=CARTESIAN_POINT('Ctrl Pts',(-3.85573030690925,1.60410667613065,-4.93878853605489));
#84791=CARTESIAN_POINT('Ctrl Pts',(-3.77674878467062,3.22939785853806,-4.06642056144451));
#84792=CARTESIAN_POINT('Ctrl Pts',(-3.69776726243198,4.12096588213986,-2.71131315212336));
#84793=CARTESIAN_POINT('Ctrl Pts',(-3.61878574019335,5.01253390574162,-1.35620574280227));
#84794=CARTESIAN_POINT('Ctrl Pts',(-3.53980421795471,5.17037877053785,0.481641101229505));
#84795=CARTESIAN_POINT('Ctrl Pts',(-3.46082269571608,4.52293098642232,1.96892791915868));
#84796=CARTESIAN_POINT('Ctrl Pts',(-3.38184117347744,3.87548320230678,3.45621473708788));
#84797=CARTESIAN_POINT('Ctrl Pts',(-3.3028596512388,2.42274276927944,4.59294152891443));
#84798=CARTESIAN_POINT('Ctrl Pts',(-3.22387812900017,0.823400118075912,
4.86370196309625));
#84799=CARTESIAN_POINT('Ctrl Pts',(-3.14489660676153,-0.775942533127614,
5.13446239727806));
#84800=CARTESIAN_POINT('Ctrl Pts',(-3.0659150845229,-2.52188740250734,4.53925647381515));
#84801=CARTESIAN_POINT('Ctrl Pts',(-2.98693356228426,-3.62280671808846,
3.34796044550116));
#84802=CARTESIAN_POINT('Ctrl Pts',(-2.92756955015737,-4.4502785842728,2.45255972559769));
#84803=CARTESIAN_POINT('Ctrl Pts',(-2.86820553803048,-4.91335544898741,
1.22040916167002));
#84804=CARTESIAN_POINT('Ctrl Pts',(-2.8088415259036,-4.92426410821032,-0.00437867314108101));
#84805=CARTESIAN_POINT('Origin',(-12.,0.,0.));
#84806=CARTESIAN_POINT('',(-1.0911584740964,-4.93200687334489,0.00268308223936954));
#84807=CARTESIAN_POINT('',(-1.30884152590359,-4.93160574955951,0.00236265628207036));
#84808=CARTESIAN_POINT('',(-12.,-4.925,-6.03138548580071E-16));
#84809=CARTESIAN_POINT('Ctrl Pts',(-1.0911584740964,-4.93200687334489,0.00268308223936954));
#84810=CARTESIAN_POINT('Ctrl Pts',(-1.09771688278017,-4.93287970031965,
0.137538864357011));
#84811=CARTESIAN_POINT('Ctrl Pts',(-1.10427529146395,-4.92789883599096,
0.272326647907248));
#84812=CARTESIAN_POINT('Ctrl Pts',(-1.11083370014772,-4.9168679637995,0.406605328980769));
#84813=CARTESIAN_POINT('Ctrl Pts',(-1.18981522238635,-4.78402551385315,
2.02369495342365));
#84814=CARTESIAN_POINT('Ctrl Pts',(-1.26879674462499,-3.77375809971144,
3.56695009160872));
#84815=CARTESIAN_POINT('Ctrl Pts',(-1.34777826686363,-2.3466871175824,4.33849087224895));
#84816=CARTESIAN_POINT('Ctrl Pts',(-1.42675978910226,-0.919616135453348,
5.11003165288917));
#84817=CARTESIAN_POINT('Ctrl Pts',(-1.5057413113409,0.924258414663064,5.10985807598457));
#84818=CARTESIAN_POINT('Ctrl Pts',(-1.58472283357954,2.35021224641849,4.33709640744291));
#84819=CARTESIAN_POINT('Ctrl Pts',(-1.66370435581817,3.77616607817389,3.56433473890127));
#84820=CARTESIAN_POINT('Ctrl Pts',(-1.74268587805681,4.78419919156834,2.01898497872259));
#84821=CARTESIAN_POINT('Ctrl Pts',(-1.82166740029545,4.91657901060328,0.402220613908327));
#84822=CARTESIAN_POINT('Ctrl Pts',(-1.90064892253408,5.04895882963822,-1.21454375090592));
#84823=CARTESIAN_POINT('Ctrl Pts',(-1.97963044477271,4.30568535431372,-2.90272272035571));
#84824=CARTESIAN_POINT('Ctrl Pts',(-2.05861196701135,3.02412028001077,-3.89713434643312));
#84825=CARTESIAN_POINT('Ctrl Pts',(-2.13759348924998,1.74255520570778,-4.89154597251055));
#84826=CARTESIAN_POINT('Ctrl Pts',(-2.21657501148862,-0.0773014675737066,
-5.1921902552155));
#84827=CARTESIAN_POINT('Ctrl Pts',(-2.29555653372726,-1.61049013445835,
-4.66261781559276));
#84828=CARTESIAN_POINT('Ctrl Pts',(-2.3745380559659,-3.143678801343,-4.13304537597002));
#84829=CARTESIAN_POINT('Ctrl Pts',(-2.45351957820454,-4.39019946183083,
-2.7732562140196));
#84830=CARTESIAN_POINT('Ctrl Pts',(-2.53250110044317,-4.78477004695423,
-1.19986364252654));
#84831=CARTESIAN_POINT('Ctrl Pts',(-2.55205355832758,-4.88244890308899,
-0.810358716338717));
#84832=CARTESIAN_POINT('Ctrl Pts',(-2.57160601621199,-4.92791629602104,
-0.407763179703401));
#84833=CARTESIAN_POINT('Ctrl Pts',(-2.5911584740964,-4.92431925468094,-0.00436907230553341));
#84834=CARTESIAN_POINT('Ctrl Pts',(-2.8088415259036,-4.92426410821032,-0.00437867314108101));
#84835=CARTESIAN_POINT('Ctrl Pts',(-2.78922401579185,-4.92786899819237,
-0.409123684020632));
#84836=CARTESIAN_POINT('Ctrl Pts',(-2.7696065056801,-4.88209500064219,-0.813064650368606));
#84837=CARTESIAN_POINT('Ctrl Pts',(-2.74998899556835,-4.78377456269397,
-1.20378326321075));
#84838=CARTESIAN_POINT('Ctrl Pts',(-2.67100747332972,-4.38792932993585,
-2.77684481044359));
#84839=CARTESIAN_POINT('Ctrl Pts',(-2.59202595109108,-3.14034510263708,
-4.13558177174419));
#84840=CARTESIAN_POINT('Ctrl Pts',(-2.51304442885244,-1.60670226458731,
-4.66391570202061));
#84841=CARTESIAN_POINT('Ctrl Pts',(-2.43406290661381,-0.0730594265375867,
-5.19224963229702));
#84842=CARTESIAN_POINT('Ctrl Pts',(-2.35508138437518,1.74664202226318,-4.89018053154927));
#84843=CARTESIAN_POINT('Ctrl Pts',(-2.27609986213654,3.02735160190436,-3.89469276235409));
#84844=CARTESIAN_POINT('Ctrl Pts',(-2.19711833989791,4.30806118154559,-2.89920499315886));
#84845=CARTESIAN_POINT('Ctrl Pts',(-2.11813681765927,5.04977889202728,-1.21029855551616));
#84846=CARTESIAN_POINT('Ctrl Pts',(-2.03915529542063,4.91615834188518,0.406301359031337));
#84847=CARTESIAN_POINT('Ctrl Pts',(-1.96017377318199,4.78253779174308,2.02290127357878));
#84848=CARTESIAN_POINT('Ctrl Pts',(-1.88119225094336,3.77357898097728,3.56719466503099));
#84849=CARTESIAN_POINT('Ctrl Pts',(-1.80221072870473,2.34683826566193,4.33889729935906));
#84850=CARTESIAN_POINT('Ctrl Pts',(-1.72322920646609,0.920097550346556,
5.11059993368714));
#84851=CARTESIAN_POINT('Ctrl Pts',(-1.64424768422745,-0.924425069518355,
5.10971181089104));
#84852=CARTESIAN_POINT('Ctrl Pts',(-1.56526616198882,-2.35056209376295,
4.33679759797832));
#84853=CARTESIAN_POINT('Ctrl Pts',(-1.48628463975018,-3.77669911800752,
3.56388338506561));
#84854=CARTESIAN_POINT('Ctrl Pts',(-1.40730311751155,-4.78445054663177,
2.01894308203631));
#84855=CARTESIAN_POINT('Ctrl Pts',(-1.32832159527291,-4.91658376485791,
0.402158723870856));
#84856=CARTESIAN_POINT('Ctrl Pts',(-1.32182823881647,-4.9274469143815,0.269237037212939));
#84857=CARTESIAN_POINT('Ctrl Pts',(-1.31533488236003,-4.93239169170165,
0.135829750947967));
#84858=CARTESIAN_POINT('Ctrl Pts',(-1.30884152590359,-4.93160574955951,
0.00236265628207036));
#84859=CARTESIAN_POINT('Origin',(-26.8478126690739,0.,0.));
#84860=CARTESIAN_POINT('',(-0.597812669073861,-4.07629116303561,0.00221756066080352));
#84861=CARTESIAN_POINT('',(-0.4,-4.0705,-3.86641296674787E-13));
#84862=CARTESIAN_POINT('',(-26.8478126690739,-4.0705,-3.86641296674787E-13));
#84863=CARTESIAN_POINT('',(-0.399999999999999,-2.75232012058015,-3.00608727173434));
#84864=CARTESIAN_POINT('Ctrl Pts',(-0.597812669073861,-4.07629116303561,
0.00221756066080327));
#84865=CARTESIAN_POINT('Ctrl Pts',(-0.531875112715907,-4.06903839051772,
-1.11836915205891));
#84866=CARTESIAN_POINT('Ctrl Pts',(-0.465937556357953,-3.57275045796359,
-2.24463667173769));
#84867=CARTESIAN_POINT('Ctrl Pts',(-0.399999999999999,-2.75232012058015,
-3.00608727173434));
#84868=CARTESIAN_POINT('Origin',(-0.4,0.,0.));
#84869=CARTESIAN_POINT('Origin',(-26.8478126690739,0.,0.));
#84870=CARTESIAN_POINT('',(-2.09781266907387,-4.06993736572157,-0.00361102717157364));
#84871=CARTESIAN_POINT('',(-1.80218733092609,-4.07595963524507,0.00195272942007198));
#84872=CARTESIAN_POINT('',(-26.8478126690739,-4.0705,-3.86641296674787E-13));
#84873=CARTESIAN_POINT('Ctrl Pts',(-2.09781266907387,-4.06993736572157,
-0.00361102717157308));
#84874=CARTESIAN_POINT('Ctrl Pts',(-2.07826021118946,-4.07291031125962,
-0.337015233093018));
#84875=CARTESIAN_POINT('Ctrl Pts',(-1.97972623106641,-3.88353374239935,
-2.01386882969969));
#84876=CARTESIAN_POINT('Ctrl Pts',(-1.80221072870472,-1.56799638829454,
-4.53981380438684));
#84877=CARTESIAN_POINT('Ctrl Pts',(-1.56526616198882,2.94432437633009,-3.79436859458956));
#84878=CARTESIAN_POINT('Ctrl Pts',(-1.32832159527291,4.78726529895451,0.391458306006858));
#84879=CARTESIAN_POINT('Ctrl Pts',(-1.091377028557,2.2878548696719,4.22314126974725));
#84880=CARTESIAN_POINT('Ctrl Pts',(-0.854432461841093,-2.28401803768771,
4.22357165236047));
#84881=CARTESIAN_POINT('Ctrl Pts',(-0.689911008680048,-4.02331967771076,
1.56666502026864));
#84882=CARTESIAN_POINT('Ctrl Pts',(-0.604371077757637,-4.07701255231495,
0.113675522307533));
#84883=CARTESIAN_POINT('Ctrl Pts',(-0.597812669073861,-4.07629116303561,
0.00221756066080327));
#84884=CARTESIAN_POINT('',(-0.4,-3.73359974356525,1.62148179294418));
#84885=CARTESIAN_POINT('Origin',(-0.4,0.,0.));
#84886=CARTESIAN_POINT('Ctrl Pts',(-1.8021873309261,-4.07595963524507,0.0019527294200722));
#84887=CARTESIAN_POINT('Ctrl Pts',(-1.72969916514391,-4.06870809992297,
-1.22948823727804));
#84888=CARTESIAN_POINT('Ctrl Pts',(-1.57822947712309,-2.82015237778342,
-3.81555274243349));
#84889=CARTESIAN_POINT('Ctrl Pts',(-1.34777826686363,1.56724719957269,-4.53861602703052));
#84890=CARTESIAN_POINT('Ctrl Pts',(-1.11083370014772,4.66076829913842,-1.17009430681153));
#84891=CARTESIAN_POINT('Ctrl Pts',(-0.873889133431818,3.52050501373642,
3.26683163619313));
#84892=CARTESIAN_POINT('Ctrl Pts',(-0.676435327835224,-0.0771870156949762,
4.48297617612786));
#84893=CARTESIAN_POINT('Ctrl Pts',(-0.518472283357957,-2.61623498089622,
3.32972304474434));
#84894=CARTESIAN_POINT('Ctrl Pts',(-0.439490761119318,-3.46537663594235,
2.23908831199168));
#84895=CARTESIAN_POINT('Ctrl Pts',(-0.4,-3.73359974356525,1.62148179294418));
#84896=CARTESIAN_POINT('Origin',(-26.8478126690739,0.,0.));
#84897=CARTESIAN_POINT('',(-3.59781266907387,-4.06463513180001,0.00163755274865575));
#84898=CARTESIAN_POINT('',(-3.3021873309261,-4.06989178730358,-0.00361896223824931));
#84899=CARTESIAN_POINT('',(-26.8478126690739,-4.0705,-3.86641296674787E-13));
#84900=CARTESIAN_POINT('Ctrl Pts',(-3.59781266907387,-4.06463513180001,
0.00163755274865576));
#84901=CARTESIAN_POINT('Ctrl Pts',(-3.55214934462127,-4.06177678722871,
-0.779568156010273));
#84902=CARTESIAN_POINT('Ctrl Pts',(-3.42750449793004,-3.46947945121757,
-2.91599699349249));
#84903=CARTESIAN_POINT('Ctrl Pts',(-3.22387812900017,-0.021433631162604,
-4.80289161377419));
#84904=CARTESIAN_POINT('Ctrl Pts',(-2.98693356228425,4.01022615884859,-2.64315364876519));
#84905=CARTESIAN_POINT('Ctrl Pts',(-2.74998899556836,4.40533498750148,1.91344654900335));
#84906=CARTESIAN_POINT('Ctrl Pts',(-2.51304442885244,0.805564524686711,
4.73490724686727));
#84907=CARTESIAN_POINT('Ctrl Pts',(-2.29565232002095,-3.1673390925526,3.38410818030933));
#84908=CARTESIAN_POINT('Ctrl Pts',(-2.15724173342809,-4.06090119376066,
1.00976029048111));
#84909=CARTESIAN_POINT('Ctrl Pts',(-2.09781266907387,-4.06993736572157,
-0.00361102717157308));
#84910=CARTESIAN_POINT('Ctrl Pts',(-3.3021873309261,-4.06989178730358,-0.00361896223824917));
#84911=CARTESIAN_POINT('Ctrl Pts',(-3.28256982081436,-4.07287121972424,
-0.338139686458441));
#84912=CARTESIAN_POINT('Ctrl Pts',(-3.18397078846399,-3.8827243702829,-2.01612514156527));
#84913=CARTESIAN_POINT('Ctrl Pts',(-3.00639023387498,-1.56436205950543,
-4.54104048789013));
#84914=CARTESIAN_POINT('Ctrl Pts',(-2.76944566715907,2.94757382720121,-3.79206245260455));
#84915=CARTESIAN_POINT('Ctrl Pts',(-2.53250110044317,4.78665724274367,0.395568199836796));
#84916=CARTESIAN_POINT('Ctrl Pts',(-2.29555653372726,2.28495155387725,4.2246319053635));
#84917=CARTESIAN_POINT('Ctrl Pts',(-2.05861196701135,-2.28852823748934,
4.22242981165284));
#84918=CARTESIAN_POINT('Ctrl Pts',(-1.89415556607763,-4.02281228208769,
1.56367365284633));
#84919=CARTESIAN_POINT('Ctrl Pts',(-1.80868068738254,-4.07660921443078,
0.11226294441258));
#84920=CARTESIAN_POINT('Ctrl Pts',(-1.8021873309261,-4.07595963524507,0.0019527294200722));
#84921=CARTESIAN_POINT('Origin',(-26.8478126690739,0.,0.));
#84922=CARTESIAN_POINT('',(-5.09781266907386,-4.07566883909993,0.00207945715039542));
#84923=CARTESIAN_POINT('',(-4.8021873309261,-4.06464833292248,0.00165346759433443));
#84924=CARTESIAN_POINT('',(-26.8478126690739,-4.0705,-3.86641296674787E-13));
#84925=CARTESIAN_POINT('Ctrl Pts',(-5.09781266907386,-4.07566883909993,
0.00207945715039548));
#84926=CARTESIAN_POINT('Ctrl Pts',(-5.02603847805308,-4.06802670929178,
-1.21733178462092));
#84927=CARTESIAN_POINT('Ctrl Pts',(-4.87528276479367,-2.84119087257745,
-3.79195219447061));
#84928=CARTESIAN_POINT('Ctrl Pts',(-4.6455455292956,1.52750104386647,-4.55356519178499));
#84929=CARTESIAN_POINT('Ctrl Pts',(-4.40860096257971,4.64807557048283,-1.20979659769575));
#84930=CARTESIAN_POINT('Ctrl Pts',(-4.17165639586379,3.55367133301375,3.23104246687973));
#84931=CARTESIAN_POINT('Ctrl Pts',(-3.93471182914789,-0.763282093062437,
4.74190020866793));
#84932=CARTESIAN_POINT('Ctrl Pts',(-3.74343058688458,-3.68951325648252,
2.49022401471519));
#84933=CARTESIAN_POINT('Ctrl Pts',(-3.6311308668599,-4.06672071998065,0.571643495768228));
#84934=CARTESIAN_POINT('Ctrl Pts',(-3.59781266907387,-4.06463513180001,
0.00163755274865576));
#84935=CARTESIAN_POINT('Ctrl Pts',(-4.8021873309261,-4.06464833292248,0.00165346759433443));
#84936=CARTESIAN_POINT('Ctrl Pts',(-4.75645895424617,-4.06175727131862,
-0.78065860445274));
#84937=CARTESIAN_POINT('Ctrl Pts',(-4.63174905532762,-3.46819584903415,
-2.91823041531605));
#84938=CARTESIAN_POINT('Ctrl Pts',(-4.42805763417042,-0.0175089406698063,
-4.80290610693659));
#84939=CARTESIAN_POINT('Ctrl Pts',(-4.19111306745452,4.01238817079558,-2.63987635628594));
#84940=CARTESIAN_POINT('Ctrl Pts',(-3.9541685007386,4.40376331119336,1.91705089973334));
#84941=CARTESIAN_POINT('Ctrl Pts',(-3.71722393402271,0.801704468977416,
4.73555632478705));
#84942=CARTESIAN_POINT('Ctrl Pts',(-3.49989687741853,-3.16893402598616,
3.38193537513361));
#84943=CARTESIAN_POINT('Ctrl Pts',(-3.361551343053,-4.06087580814292,1.00866507463471));
#84944=CARTESIAN_POINT('Ctrl Pts',(-3.3021873309261,-4.06989178730358,-0.00361896223824917));
#84945=CARTESIAN_POINT('Origin',(-26.8478126690739,0.,0.));
#84946=CARTESIAN_POINT('',(-6.59781266907387,-4.07024966429081,-0.00362411170895328));
#84947=CARTESIAN_POINT('',(-6.3021873309261,-4.07569093726617,0.00206331041636865));
#84948=CARTESIAN_POINT('',(-26.8478126690739,-4.0705,-3.86641296674787E-13));
#84949=CARTESIAN_POINT('Ctrl Pts',(-6.59781266907387,-4.07024966429081,
-0.00362411170895308));
#84950=CARTESIAN_POINT('Ctrl Pts',(-6.57890913372353,-4.07314624420103,
-0.325897404679135));
#84951=CARTESIAN_POINT('Ctrl Pts',(-6.48102407613457,-3.89142584068926,
-1.99144484346476));
#84952=CARTESIAN_POINT('Ctrl Pts',(-6.30415749630696,-1.60505193339804,
-4.52681160940636));
#84953=CARTESIAN_POINT('Ctrl Pts',(-6.06721292959105,2.91345381090988,-3.81837687463714));
#84954=CARTESIAN_POINT('Ctrl Pts',(-5.83026836287515,4.78997440289178,0.352647507803434));
#84955=CARTESIAN_POINT('Ctrl Pts',(-5.59332379615923,2.322838960361,4.20388323073168));
#84956=CARTESIAN_POINT('Ctrl Pts',(-5.35637922944334,-2.25069887035317,
4.24294351890926));
#84957=CARTESIAN_POINT('Ctrl Pts',(-5.1912088537482,-4.01610269075381,1.58807231517304));
#84958=CARTESIAN_POINT('Ctrl Pts',(-5.10502000029171,-4.07643623696194,
0.124528774728565));
#84959=CARTESIAN_POINT('Ctrl Pts',(-5.09781266907386,-4.07566883909993,
0.00207945715039548));
#84960=CARTESIAN_POINT('Ctrl Pts',(-6.3021873309261,-4.07569093726617,0.00206331041636901));
#84961=CARTESIAN_POINT('Ctrl Pts',(-6.23034808767799,-4.06809019538989,
-1.21843532036503));
#84962=CARTESIAN_POINT('Ctrl Pts',(-6.07952732219125,-2.83932709572212,
-3.79405859128264));
#84963=CARTESIAN_POINT('Ctrl Pts',(-5.84972503446587,1.53122279065449,-4.55231461594934));
#84964=CARTESIAN_POINT('Ctrl Pts',(-5.61278046774996,4.6490626950213,-1.20599647826086));
#84965=CARTESIAN_POINT('Ctrl Pts',(-5.37583590103405,3.55102848107464,3.23394623945287));
#84966=CARTESIAN_POINT('Ctrl Pts',(-5.13889133431815,-0.767157925271441,
4.74127415374739));
#84967=CARTESIAN_POINT('Ctrl Pts',(-4.94767514428216,-3.69055317518662,
2.48797370675018));
#84968=CARTESIAN_POINT('Ctrl Pts',(-4.83544047648481,-4.06675067941523,
0.570541739885505));
#84969=CARTESIAN_POINT('Ctrl Pts',(-4.8021873309261,-4.06464833292248,0.00165346759433443));
#84970=CARTESIAN_POINT('Origin',(-26.8478126690739,0.,0.));
#84971=CARTESIAN_POINT('',(-8.09781266907387,-4.06450654082374,0.00147586284968758));
#84972=CARTESIAN_POINT('',(-7.8021873309261,-4.07021649832878,-0.00362428100020962));
#84973=CARTESIAN_POINT('',(-26.8478126690739,-4.0705,-3.86641296674787E-13));
#84974=CARTESIAN_POINT('Ctrl Pts',(-8.09781266907387,-4.06450654082374,
0.00147586284968748));
#84975=CARTESIAN_POINT('Ctrl Pts',(-8.05279826715535,-4.0619715081721,-0.768689145848125));
#84976=CARTESIAN_POINT('Ctrl Pts',(-7.9288023429982,-3.48220316311878,-2.89371114037708));
#84977=CARTESIAN_POINT('Ctrl Pts',(-7.7258248966024,-0.0605998926332336,
-4.80255585185065));
#84978=CARTESIAN_POINT('Ctrl Pts',(-7.48888032988651,3.98854254916481,-2.67576968195071));
#84979=CARTESIAN_POINT('Ctrl Pts',(-7.25193576317058,4.42078530124335,1.87746434781877));
#84980=CARTESIAN_POINT('Ctrl Pts',(-7.01499119645469,0.844160957960478,
4.72817166925782));
#84981=CARTESIAN_POINT('Ctrl Pts',(-6.79695016508911,-3.15155064707133,
3.40590389765473));
#84982=CARTESIAN_POINT('Ctrl Pts',(-6.65789065596217,-4.06104394236409,
1.02060391287446));
#84983=CARTESIAN_POINT('Ctrl Pts',(-6.59781266907387,-4.07024966429081,
-0.00362411170895308));
#84984=CARTESIAN_POINT('Ctrl Pts',(-7.8021873309261,-4.07021649832878,-0.00362428100020934));
#84985=CARTESIAN_POINT('Ctrl Pts',(-7.78321874334844,-4.07312102749033,
-0.327013257474892));
#84986=CARTESIAN_POINT('Ctrl Pts',(-7.68526863353215,-3.89063799663387,
-1.99369332115123));
#84987=CARTESIAN_POINT('Ctrl Pts',(-7.50833700147722,-1.60135074079071,
-4.52812183462507));
#84988=CARTESIAN_POINT('Ctrl Pts',(-7.2713924347613,2.91657402449002,-3.81599364587164));
#84989=CARTESIAN_POINT('Ctrl Pts',(-7.03444786804541,4.78968416005308,0.356563023868872));
#84990=CARTESIAN_POINT('Ctrl Pts',(-6.79750330132949,2.31940145568391,4.2057803592973));
#84991=CARTESIAN_POINT('Ctrl Pts',(-6.5605587346136,-2.25416642273435,4.24110189585783));
#84992=CARTESIAN_POINT('Ctrl Pts',(-6.39545341114579,-4.01670480150413,
1.58583480923292));
#84993=CARTESIAN_POINT('Ctrl Pts',(-6.30932960991663,-4.07644660529051,
0.123405648315058));
#84994=CARTESIAN_POINT('Ctrl Pts',(-6.3021873309261,-4.07569093726617,0.00206331041636901));
#84995=CARTESIAN_POINT('Origin',(-26.8478126690739,0.,0.));
#84996=CARTESIAN_POINT('',(-9.59781266907388,-4.07543761133748,0.00223681958108363));
#84997=CARTESIAN_POINT('',(-9.30218733092611,-4.06451849691004,0.00149222602727483));
#84998=CARTESIAN_POINT('',(-26.8478126690739,-4.0705,-3.86641296674787E-13));
#84999=CARTESIAN_POINT('Ctrl Pts',(-9.59781266907388,-4.07543761133748,
0.00223681958108334));
#85000=CARTESIAN_POINT('Ctrl Pts',(-9.52668740058717,-4.06740685118034,
-1.20633045978605));
#85001=CARTESIAN_POINT('Ctrl Pts',(-9.37658060986182,-2.85969592298694,
-3.77090943721607));
#85002=CARTESIAN_POINT('Ctrl Pts',(-9.14749229689786,1.49031812597541,-4.56586979014612));
#85003=CARTESIAN_POINT('Ctrl Pts',(-8.91054773018194,4.63805579586533,-1.24765920492107));
#85004=CARTESIAN_POINT('Ctrl Pts',(-8.67360316346604,3.57990062094709,3.20195668323646));
#85005=CARTESIAN_POINT('Ctrl Pts',(-8.43665859675013,-0.724588593371072,
4.74796655711994));
#85006=CARTESIAN_POINT('Ctrl Pts',(-8.24472843195274,-3.67907357692905,
2.51267002599099));
#85007=CARTESIAN_POINT('Ctrl Pts',(-8.13177978939398,-4.06641943437389,
0.582629591474945));
#85008=CARTESIAN_POINT('Ctrl Pts',(-8.09781266907387,-4.06450654082374,
0.00147586284968748));
#85009=CARTESIAN_POINT('Ctrl Pts',(-9.30218733092611,-4.06451849691004,
0.00149222602727511));
#85010=CARTESIAN_POINT('Ctrl Pts',(-9.25710787678026,-4.06195119816851,
-0.76977989625584));
#85011=CARTESIAN_POINT('Ctrl Pts',(-9.13304690039577,-3.48093330077731,
-2.89594568183173));
#85012=CARTESIAN_POINT('Ctrl Pts',(-8.93000440177266,-0.0566739212580544,
-4.80260342014054));
#85013=CARTESIAN_POINT('Ctrl Pts',(-8.69305983505675,3.99072827488727,-2.67250806931295));
#85014=CARTESIAN_POINT('Ctrl Pts',(-8.45611526834084,4.41924871633079,1.88107743798526));
#85015=CARTESIAN_POINT('Ctrl Pts',(-8.21917070162494,0.840295471934814,
4.72885980594699));
#85016=CARTESIAN_POINT('Ctrl Pts',(-8.00119472248669,-3.15314178729772,
3.40372167243926));
#85017=CARTESIAN_POINT('Ctrl Pts',(-7.86220026558708,-4.06102713100874,
1.01951576228452));
#85018=CARTESIAN_POINT('Ctrl Pts',(-7.8021873309261,-4.07021649832878,-0.00362428100020934));
#85019=CARTESIAN_POINT('Origin',(-26.8478126690739,0.,0.));
#85020=CARTESIAN_POINT('',(-11.0978126690739,-4.07057840008889,-0.00361717664568562));
#85021=CARTESIAN_POINT('',(-10.8021873309261,-4.07546109772978,0.00222135529329905));
#85022=CARTESIAN_POINT('',(-26.8478126690739,-4.0705,-3.86641296674787E-13));
#85023=CARTESIAN_POINT('Ctrl Pts',(-11.0978126690739,-4.07057840008889,
-0.00361717664568554));
#85024=CARTESIAN_POINT('Ctrl Pts',(-11.0795580562576,-4.07339138512556,
-0.314763099123047));
#85025=CARTESIAN_POINT('Ctrl Pts',(-10.9823219212027,-3.8992231551958,-1.96901630061212));
#85026=CARTESIAN_POINT('Ctrl Pts',(-10.8061042639092,-1.64191250099602,
-4.51357268649284));
#85027=CARTESIAN_POINT('Ctrl Pts',(-10.5691596971933,2.88221994700369,-3.84200770877353));
#85028=CARTESIAN_POINT('Ctrl Pts',(-10.3322151304774,4.79269081226222,0.313575884338453));
#85029=CARTESIAN_POINT('Ctrl Pts',(-10.0952705637615,2.35704233746519,4.18480184436228));
#85030=CARTESIAN_POINT('Ctrl Pts',(-9.85832599704557,-2.21602490467178,
4.26115579145559));
#85031=CARTESIAN_POINT('Ctrl Pts',(-9.69250669881637,-4.0100399692706,1.61039529938039));
#85032=CARTESIAN_POINT('Ctrl Pts',(-9.6056689228258,-4.07632466162154,0.135731025297307));
#85033=CARTESIAN_POINT('Ctrl Pts',(-9.59781266907388,-4.07543761133748,
0.00223681958108334));
#85034=CARTESIAN_POINT('Ctrl Pts',(-10.8021873309261,-4.07546109772978,
0.00222135529329927));
#85035=CARTESIAN_POINT('Ctrl Pts',(-10.7309970102121,-4.06746733027052,
-1.20743258301197));
#85036=CARTESIAN_POINT('Ctrl Pts',(-10.5808251672594,-2.85784756339483,
-3.7730208783109));
#85037=CARTESIAN_POINT('Ctrl Pts',(-10.3516718020681,1.49404997724334,-4.56464962620395));
#85038=CARTESIAN_POINT('Ctrl Pts',(-10.1147272353522,4.63907381730574,-1.24386722044341));
#85039=CARTESIAN_POINT('Ctrl Pts',(-9.8777826686363,3.57728164792448,3.20488183181962));
#85040=CARTESIAN_POINT('Ctrl Pts',(-9.64083810192037,-0.728469617480856,
4.74737227957853));
#85041=CARTESIAN_POINT('Ctrl Pts',(-9.44897298935032,-3.68012533608753,
2.51041990486184));
#85042=CARTESIAN_POINT('Ctrl Pts',(-9.3360893990189,-4.06644923760776,0.581528530883969));
#85043=CARTESIAN_POINT('Ctrl Pts',(-9.30218733092611,-4.06451849691004,
0.00149222602727511));
#85044=CARTESIAN_POINT('Origin',(-26.8478126690739,0.,0.));
#85045=CARTESIAN_POINT('',(-12.5978126690739,-4.06439173936514,0.00131077860369149));
#85046=CARTESIAN_POINT('',(-12.3021873309261,-4.07054506653231,-0.00361830226162985));
#85047=CARTESIAN_POINT('',(-26.8478126690739,-4.0705,-3.86641296674787E-13));
#85048=CARTESIAN_POINT('Ctrl Pts',(-12.5978126690739,-4.06439173936514,
0.00131077860369144));
#85049=CARTESIAN_POINT('Ctrl Pts',(-12.5534471896894,-4.06217639157224,
-0.757805274824507));
#85050=CARTESIAN_POINT('Ctrl Pts',(-12.4301001880664,-3.49479538377389,
-2.87141087514505));
#85051=CARTESIAN_POINT('Ctrl Pts',(-12.2277716642046,-0.0997603707836814,
-4.80190201124536));
#85052=CARTESIAN_POINT('Ctrl Pts',(-11.9908270974887,3.96659034332826,-2.70820532925335));
#85053=CARTESIAN_POINT('Ctrl Pts',(-11.7538825307728,4.43594811954626,1.84135258380226));
#85054=CARTESIAN_POINT('Ctrl Pts',(-11.5169379640569,0.882688817166835,
4.72113074477184));
#85055=CARTESIAN_POINT('Ctrl Pts',(-11.2982480101573,-3.1355959094005,3.4276518469622));
#85056=CARTESIAN_POINT('Ctrl Pts',(-11.1585395784963,-4.06122055233565,
1.03145984424838));
#85057=CARTESIAN_POINT('Ctrl Pts',(-11.0978126690739,-4.07057840008889,
-0.00361717664568554));
#85058=CARTESIAN_POINT('Ctrl Pts',(-12.3021873309261,-4.07054506653231,
-0.00361830226162995));
#85059=CARTESIAN_POINT('Ctrl Pts',(-12.2838676658825,-4.07336677593993,
-0.315879491868212));
#85060=CARTESIAN_POINT('Ctrl Pts',(-12.1865664786003,-3.89844601596142,
-1.97126432893802));
#85061=CARTESIAN_POINT('Ctrl Pts',(-12.0102837690795,-1.63822211600786,
-4.514913049343));
#85062=CARTESIAN_POINT('Ctrl Pts',(-11.7733392023635,2.88535949150936,-3.83965000348491));
#85063=CARTESIAN_POINT('Ctrl Pts',(-11.5363946356477,4.79243250703115,0.317493637819545));
#85064=CARTESIAN_POINT('Ctrl Pts',(-11.2994500689317,2.35362041946459,4.18672693945812));
#85065=CARTESIAN_POINT('Ctrl Pts',(-11.0625055022158,-2.21950736358003,
4.25934250882913));
#85066=CARTESIAN_POINT('Ctrl Pts',(-10.8967512562139,-4.0106518183616,1.60815703963873));
#85067=CARTESIAN_POINT('Ctrl Pts',(-10.8099785324507,-4.07633595055516,
0.134608139252678));
#85068=CARTESIAN_POINT('Ctrl Pts',(-10.8021873309261,-4.07546109772978,
0.00222135529329927));
#85069=CARTESIAN_POINT('Origin',(-26.8478126690739,0.,0.));
#85070=CARTESIAN_POINT('',(-14.0978126690739,-4.07519307943845,0.00238714832353424));
#85071=CARTESIAN_POINT('',(-13.8021873309261,-4.0644023160722,0.00132747365239078));
#85072=CARTESIAN_POINT('',(-26.8478126690739,-4.0705,-3.86641296674787E-13));
#85073=CARTESIAN_POINT('Ctrl Pts',(-14.0978126690739,-4.07519307943845,
0.00238714832353427));
#85074=CARTESIAN_POINT('Ctrl Pts',(-14.0273363231212,-4.06681676123038,
-1.19534282954133));
#85075=CARTESIAN_POINT('Ctrl Pts',(-13.87787845493,-2.87804755341778,-3.74981687266502));
#85076=CARTESIAN_POINT('Ctrl Pts',(-13.6494390645001,1.45303614102348,-4.57787079656698));
#85077=CARTESIAN_POINT('Ctrl Pts',(-13.4124944977842,4.6277275367991,-1.28543879758337));
#85078=CARTESIAN_POINT('Ctrl Pts',(-13.1755499310683,3.6058919843453,3.17265788486808));
#85079=CARTESIAN_POINT('Ctrl Pts',(-12.9386053643524,-0.68584715780348,
4.75371735942664));
#85080=CARTESIAN_POINT('Ctrl Pts',(-12.7460262770209,-3.66851217096832,
2.53511162155732));
#85081=CARTESIAN_POINT('Ctrl Pts',(-12.6324287119281,-4.06612025836685,
0.593608984356713));
#85082=CARTESIAN_POINT('Ctrl Pts',(-12.5978126690739,-4.06439173936514,
0.00131077860369144));
#85083=CARTESIAN_POINT('Ctrl Pts',(-13.8021873309261,-4.0644023160722,0.00132747365239085));
#85084=CARTESIAN_POINT('Ctrl Pts',(-13.7577567993143,-4.06215511076084,
-0.758896503957548));
#85085=CARTESIAN_POINT('Ctrl Pts',(-13.6343447454639,-3.49353872825462,
-2.87364679360195));
#85086=CARTESIAN_POINT('Ctrl Pts',(-13.4319511693749,-0.0958349178438527,
-4.80198159232485));
#85087=CARTESIAN_POINT('Ctrl Pts',(-13.195006602659,3.96880259324556,-2.70496164859175));
#85088=CARTESIAN_POINT('Ctrl Pts',(-12.9580620359431,4.43444104868229,1.84497808395286));
#85089=CARTESIAN_POINT('Ctrl Pts',(-12.7211174692272,0.878829071125367,
4.72185037969754));
#85090=CARTESIAN_POINT('Ctrl Pts',(-12.5024925675548,-3.13720164930185,
3.42547292377134));
#85091=CARTESIAN_POINT('Ctrl Pts',(-12.3628491881212,-4.06120154782041,
1.03037132835712));
#85092=CARTESIAN_POINT('Ctrl Pts',(-12.3021873309261,-4.07054506653231,
-0.00361830226162995));
#85093=CARTESIAN_POINT('Origin',(-26.8478126690739,0.,0.));
#85094=CARTESIAN_POINT('',(-15.5978126690739,-4.07090838159082,-0.0036006753872044));
#85095=CARTESIAN_POINT('',(-15.3021873309261,-4.07521785360078,0.00237240612388764));
#85096=CARTESIAN_POINT('',(-26.8478126690739,-4.0705,-3.86641296674787E-13));
#85097=CARTESIAN_POINT('Ctrl Pts',(-15.5978126690739,-4.07090838159082,
-0.00360067538720397));
#85098=CARTESIAN_POINT('Ctrl Pts',(-15.5802069787917,-4.0736303253679,-0.303623491996831));
#85099=CARTESIAN_POINT('Ctrl Pts',(-15.4836197662709,-3.90691400355826,
-1.94659239353253));
#85100=CARTESIAN_POINT('Ctrl Pts',(-15.3080510315115,-1.6786638864531,-4.50003362359639));
#85101=CARTESIAN_POINT('Ctrl Pts',(-15.0711064647955,2.85079442437809,-3.86538306085168));
#85102=CARTESIAN_POINT('Ctrl Pts',(-14.8341618980796,4.79508852002207,0.274483409940331));
#85103=CARTESIAN_POINT('Ctrl Pts',(-14.5972173313637,2.39108898052815,4.16544217873422));
#85104=CARTESIAN_POINT('Ctrl Pts',(-14.3602727646478,-2.18120358456222,
4.27908471286496));
#85105=CARTESIAN_POINT('Ctrl Pts',(-14.1938045438845,-4.00387976925298,
1.632725694837));
#85106=CARTESIAN_POINT('Ctrl Pts',(-14.1063178453599,-4.07620394431835,
0.14693074613754));
#85107=CARTESIAN_POINT('Ctrl Pts',(-14.0978126690739,-4.07519307943845,
0.00238714832353427));
#85108=CARTESIAN_POINT('Ctrl Pts',(-15.3021873309261,-4.07521785360078,
0.0023724061238877));
#85109=CARTESIAN_POINT('Ctrl Pts',(-15.2316459327462,-4.06687427621052,
-1.19644361288041));
#85110=CARTESIAN_POINT('Ctrl Pts',(-15.0821230123276,-2.87621455521643,
-3.75193325755229));
#85111=CARTESIAN_POINT('Ctrl Pts',(-14.8536185696703,1.45677781805249,-4.57668110461451));
#85112=CARTESIAN_POINT('Ctrl Pts',(-14.6166740029544,4.62877644616991,-1.28165524065066));
#85113=CARTESIAN_POINT('Ctrl Pts',(-14.3797294362385,3.60329695155474,3.17560429263805));
#85114=CARTESIAN_POINT('Ctrl Pts',(-14.1427848695226,-0.689732898916454,
4.75315474949608));
#85115=CARTESIAN_POINT('Ctrl Pts',(-13.9502708344185,-3.66957612834082,
2.53286193889574));
#85116=CARTESIAN_POINT('Ctrl Pts',(-13.836738321553,-4.06614983443025,0.59250859554932));
#85117=CARTESIAN_POINT('Ctrl Pts',(-13.8021873309261,-4.0644023160722,0.00132747365239085));
#85118=CARTESIAN_POINT('Origin',(-26.8478126690739,0.,0.));
#85119=CARTESIAN_POINT('',(-17.0978126690739,-4.06429080835649,0.00114260236847386));
#85120=CARTESIAN_POINT('',(-16.8021873309261,-4.07087495827563,-0.00360276185568886));
#85121=CARTESIAN_POINT('',(-26.8478126690739,-4.0705,-3.86641296674787E-13));
#85122=CARTESIAN_POINT('Ctrl Pts',(-17.0978126690739,-4.06429080835649,
0.00114260236847394));
#85123=CARTESIAN_POINT('Ctrl Pts',(-17.0540961122235,-4.06239068999993,
-0.746916525723744));
#85124=CARTESIAN_POINT('Ctrl Pts',(-16.9313980331345,-3.50725618954384,
-2.84909725496437));
#85125=CARTESIAN_POINT('Ctrl Pts',(-16.7297184318069,-0.138914215188535,
-4.80092885781891));
#85126=CARTESIAN_POINT('Ctrl Pts',(-16.492773865091,3.94437437056674,-2.74046088863915));
#85127=CARTESIAN_POINT('Ctrl Pts',(-16.2558292983751,4.45081595990773,1.8051183751108));
#85128=CARTESIAN_POINT('Ctrl Pts',(-16.0188847316592,0.921157980137197,
4.71377587850701));
#85129=CARTESIAN_POINT('Ctrl Pts',(-15.7995458552254,-3.11949526030155,
3.44936632830614));
#85130=CARTESIAN_POINT('Ctrl Pts',(-15.6591885010303,-4.06141931520493,
1.04231968787035));
#85131=CARTESIAN_POINT('Ctrl Pts',(-15.5978126690739,-4.07090838159082,
-0.00360067538720397));
#85132=CARTESIAN_POINT('Ctrl Pts',(-16.8021873309261,-4.07087495827563,
-0.00360276185568931));
#85133=CARTESIAN_POINT('Ctrl Pts',(-16.7845165884166,-4.07360634907373,
-0.304740410768458));
#85134=CARTESIAN_POINT('Ctrl Pts',(-16.6878643236685,-3.90614750997477,
-1.94883994785539));
#85135=CARTESIAN_POINT('Ctrl Pts',(-16.5122305366817,-1.67498455417103,
-4.50140403516247));
#85136=CARTESIAN_POINT('Ctrl Pts',(-16.2752859699658,2.85395309043288,-3.86305103540403));
#85137=CARTESIAN_POINT('Ctrl Pts',(-16.0383414032499,4.79486217074114,0.278403139515235));
#85138=CARTESIAN_POINT('Ctrl Pts',(-15.801396836534,2.38768287451035,4.16739511388991));
#85139=CARTESIAN_POINT('Ctrl Pts',(-15.5644522698181,-2.18470071411643,
4.27729988827614));
#85140=CARTESIAN_POINT('Ctrl Pts',(-15.3980491012821,-4.00450141399627,
1.63048669485744));
#85141=CARTESIAN_POINT('Ctrl Pts',(-15.3106274549848,-4.07621614439291,
0.145808121675198));
#85142=CARTESIAN_POINT('Ctrl Pts',(-15.3021873309261,-4.07521785360078,
0.0023724061238877));
#85143=CARTESIAN_POINT('Origin',(-26.8478126690739,0.,0.));
#85144=CARTESIAN_POINT('',(-18.5978126690739,-4.07493625768978,0.00253007724807807));
#85145=CARTESIAN_POINT('',(-18.3021873309261,-4.06429998606454,0.00115958952258771));
#85146=CARTESIAN_POINT('',(-26.8478126690739,-4.0705,-3.86641296674787E-13));
#85147=CARTESIAN_POINT('Ctrl Pts',(-18.5978126690739,-4.07493625768978,
0.00253007724807795));
#85148=CARTESIAN_POINT('Ctrl Pts',(-18.5279852456553,-4.06625599752369,
-1.18436818426556));
#85149=CARTESIAN_POINT('Ctrl Pts',(-18.3791762999982,-2.89624616201064,
-3.72867561089757));
#85150=CARTESIAN_POINT('Ctrl Pts',(-18.1513858321023,1.41565753192185,-4.58956738674043));
#85151=CARTESIAN_POINT('Ctrl Pts',(-17.9144412653864,4.61709154776294,-1.32313291269056));
#85152=CARTESIAN_POINT('Ctrl Pts',(-17.6774966986705,3.63164356582701,3.14314811403285));
#85153=CARTESIAN_POINT('Ctrl Pts',(-17.4405521319546,-0.647060115157983,
4.75915205295132));
#85154=CARTESIAN_POINT('Ctrl Pts',(-17.247324122089,-3.65782874417121,2.55754855348124));
#85155=CARTESIAN_POINT('Ctrl Pts',(-17.1330776344621,-4.06582358250215,
0.604581691838573));
#85156=CARTESIAN_POINT('Ctrl Pts',(-17.0978126690739,-4.06429080835649,
0.00114260236847394));
#85157=CARTESIAN_POINT('Ctrl Pts',(-18.3021873309261,-4.06429998606454,
0.00115958952258736));
#85158=CARTESIAN_POINT('Ctrl Pts',(-18.2584057218484,-4.0623684874239,-0.74800825355675));
#85159=CARTESIAN_POINT('Ctrl Pts',(-18.1356425905321,-3.50601267898312,
-2.8513344844204));
#85160=CARTESIAN_POINT('Ctrl Pts',(-17.9338979369771,-0.134989541855146,
-4.801040446262));
#85161=CARTESIAN_POINT('Ctrl Pts',(-17.6969533702612,3.94661299763452,-2.73723535571292));
#85162=CARTESIAN_POINT('Ctrl Pts',(-17.4600088035453,4.44933850329186,1.80875604418168));
#85163=CARTESIAN_POINT('Ctrl Pts',(-17.2230642368294,0.917304230718045,
4.71452696382671));
#85164=CARTESIAN_POINT('Ctrl Pts',(-17.003790412623,-3.12111565197432,3.44719080073753));
#85165=CARTESIAN_POINT('Ctrl Pts',(-16.8634981106552,-4.06139806733649,
1.0412307560742));
#85166=CARTESIAN_POINT('Ctrl Pts',(-16.8021873309261,-4.07087495827563,
-0.00360276185568931));
#85167=CARTESIAN_POINT('Origin',(-26.8478126690739,0.,0.));
#85168=CARTESIAN_POINT('',(-20.0978126690739,-4.071238829888,-0.00357457003402451));
#85169=CARTESIAN_POINT('',(-19.8021873309261,-4.07496222722346,0.00251610070729075));
#85170=CARTESIAN_POINT('',(-26.8478126690739,-4.0705,-3.86641296674787E-13));
#85171=CARTESIAN_POINT('Ctrl Pts',(-20.0978126690739,-4.071238829888,-0.00357457003402478));
#85172=CARTESIAN_POINT('Ctrl Pts',(-20.0808559013258,-4.07386284930607,
-0.292478704003469));
#85173=CARTESIAN_POINT('Ctrl Pts',(-19.9849176113391,-3.91449912999133,
-1.92417326350588));
#85174=CARTESIAN_POINT('Ctrl Pts',(-19.8099977991137,-1.71530351140438,
-4.48619540698215));
#85175=CARTESIAN_POINT('Ctrl Pts',(-19.5730532323978,2.8191792622351,-3.88850133137423));
#85176=CARTESIAN_POINT('Ctrl Pts',(-19.3361086656818,4.79716740439492,0.23537265996686));
#85177=CARTESIAN_POINT('Ctrl Pts',(-19.099164098966,2.42497660407891,4.14580553515268));
#85178=CARTESIAN_POINT('Ctrl Pts',(-18.86221953225,-2.14623721078936,4.29672908104936));
#85179=CARTESIAN_POINT('Ctrl Pts',(-18.6951023889527,-3.99762156681033,
1.65506339659562));
#85180=CARTESIAN_POINT('Ctrl Pts',(-18.606966767894,-4.07607420543945,0.158127741365762));
#85181=CARTESIAN_POINT('Ctrl Pts',(-18.5978126690739,-4.07493625768978,
0.00253007724807795));
#85182=CARTESIAN_POINT('Ctrl Pts',(-19.8021873309261,-4.07496222722346,
0.0025161007072908));
#85183=CARTESIAN_POINT('Ctrl Pts',(-19.7322948552802,-4.06631060333232,
-1.18546768844045));
#85184=CARTESIAN_POINT('Ctrl Pts',(-19.5834208573957,-2.89442846977801,
-3.73079684269773));
#85185=CARTESIAN_POINT('Ctrl Pts',(-19.3555653372726,1.4194087785671,-4.58840823893679));
#85186=CARTESIAN_POINT('Ctrl Pts',(-19.1186207705567,4.61817127913257,-1.31935803851751));
#85187=CARTESIAN_POINT('Ctrl Pts',(-18.8816762038408,3.62907264384353,3.14611558694568));
#85188=CARTESIAN_POINT('Ctrl Pts',(-18.6447316371248,-0.650950313849541,
4.75862114706335));
#85189=CARTESIAN_POINT('Ctrl Pts',(-18.4515686794867,-3.65890496319905,
2.55529935938178));
#85190=CARTESIAN_POINT('Ctrl Pts',(-18.3373872440871,-4.06585288888957,
0.603481970423879));
#85191=CARTESIAN_POINT('Ctrl Pts',(-18.3021873309261,-4.06429998606454,
0.00115958952258736));
#85192=CARTESIAN_POINT('Origin',(-26.8478126690739,0.,0.));
#85193=CARTESIAN_POINT('',(-21.5978126690739,-4.06419832734502,0.00096815537284884));
#85194=CARTESIAN_POINT('',(-21.3021873309261,-4.07120543337986,-0.00357758459923085));
#85195=CARTESIAN_POINT('',(-26.8478126690739,-4.0705,-3.86641296674787E-13));
#85196=CARTESIAN_POINT('Ctrl Pts',(-21.5978126690739,-4.06419832734502,
0.000968155372848833));
#85197=CARTESIAN_POINT('Ctrl Pts',(-21.5547450347576,-4.06261112671129,
-0.736024486956658));
#85198=CARTESIAN_POINT('Ctrl Pts',(-21.4326958782027,-3.51959617795593,
-2.826764557928));
#85199=CARTESIAN_POINT('Ctrl Pts',(-21.2316651994091,-0.178052071836572,
-4.79964076861094));
#85200=CARTESIAN_POINT('Ctrl Pts',(-20.9947206326932,3.92189259497827,-2.77253197087948));
#85201=CARTESIAN_POINT('Ctrl Pts',(-20.7577760659773,4.46538966209699,1.76876296315944));
#85202=CARTESIAN_POINT('Ctrl Pts',(-20.5208314992614,0.959564937147886,
4.70610816747424));
#85203=CARTESIAN_POINT('Ctrl Pts',(-20.3008437002936,-3.10324779081687,
3.47104615142249));
#85204=CARTESIAN_POINT('Ctrl Pts',(-20.1598374235644,-4.06164064687329,
1.05318390227358));
#85205=CARTESIAN_POINT('Ctrl Pts',(-20.0978126690739,-4.071238829888,-0.00357457003402478));
#85206=CARTESIAN_POINT('Ctrl Pts',(-21.3021873309261,-4.07120543337986,
-0.00357758459923137));
#85207=CARTESIAN_POINT('Ctrl Pts',(-21.2851655109507,-4.07383969984574,
-0.293595973708156));
#85208=CARTESIAN_POINT('Ctrl Pts',(-21.1891621687366,-3.91374404213,-1.92641954377506));
#85209=CARTESIAN_POINT('Ctrl Pts',(-21.0141773042839,-1.71163476880105,
-4.48759644703182));
#85210=CARTESIAN_POINT('Ctrl Pts',(-20.777232737568,2.82235647137499,-3.88619479158027));
#85211=CARTESIAN_POINT('Ctrl Pts',(-20.5402881708521,4.79697321791449,0.239293923164062));
#85212=CARTESIAN_POINT('Ctrl Pts',(-20.3033436041362,2.42158643669063,4.14778627515724));
#85213=CARTESIAN_POINT('Ctrl Pts',(-20.0663990374203,-2.14974872645911,
4.2949727839084));
#85214=CARTESIAN_POINT('Ctrl Pts',(-19.8993469463503,-3.99825306426731,
1.65282367123152));
#85215=CARTESIAN_POINT('Ctrl Pts',(-19.8112763775189,-4.07608731274838,
0.157005406047044));
#85216=CARTESIAN_POINT('Ctrl Pts',(-19.8021873309261,-4.07496222722346,
0.0025161007072908));
#85217=CARTESIAN_POINT('Origin',(-26.8478126690739,0.,0.));
#85218=CARTESIAN_POINT('',(-23.0978126690739,-4.07427440555673,0.00241395537052257));
#85219=CARTESIAN_POINT('',(-22.8021873309261,-4.06417652423825,0.000957366820343863));
#85220=CARTESIAN_POINT('',(-26.8478126690739,-4.0705,-3.86641296674787E-13));
#85221=CARTESIAN_POINT('Ctrl Pts',(-23.0978126690739,-4.07427440555673,
0.002413955370523));
#85222=CARTESIAN_POINT('Ctrl Pts',(-23.0286341681894,-4.06525490317439,
-1.17370585999422));
#85223=CARTESIAN_POINT('Ctrl Pts',(-22.8804741450663,-2.91490401827704,
-3.70709582083626));
#85224=CARTESIAN_POINT('Ctrl Pts',(-22.6533325997046,1.37852450357098,-4.60117581069992));
#85225=CARTESIAN_POINT('Ctrl Pts',(-22.4163880329887,4.60597174073038,-1.36062610156221));
#85226=CARTESIAN_POINT('Ctrl Pts',(-22.1794434662727,3.65724566378385,3.11337055406841));
#85227=CARTESIAN_POINT('Ctrl Pts',(-21.9424988995569,-0.608277930885338,
4.76430086728238));
#85228=CARTESIAN_POINT('Ctrl Pts',(-21.7486219671572,-3.64701097805702,
2.57997285182622));
#85229=CARTESIAN_POINT('Ctrl Pts',(-21.6337265569962,-4.0655218861282,0.615542686256921));
#85230=CARTESIAN_POINT('Ctrl Pts',(-21.5978126690739,-4.06419832734502,
0.000968155372848833));
#85231=CARTESIAN_POINT('Ctrl Pts',(-22.8021873309261,-4.06417652423825,
0.000957366820343933));
#85232=CARTESIAN_POINT('Ctrl Pts',(-22.7590546443825,-4.06257329236665,
-0.737130721986723));
#85233=CARTESIAN_POINT('Ctrl Pts',(-22.6369404356002,-3.51841833318712,
-2.82895318080592));
#85234=CARTESIAN_POINT('Ctrl Pts',(-22.4358447045794,-0.174092888986568,
-4.79981806178492));
#85235=CARTESIAN_POINT('Ctrl Pts',(-22.1989001378634,3.92413894310881,-2.76930725388711));
#85236=CARTESIAN_POINT('Ctrl Pts',(-21.9619555711476,4.46395155275901,1.77240342487198));
#85237=CARTESIAN_POINT('Ctrl Pts',(-21.7250110044316,0.955712424786761,
4.70689540849193));
#85238=CARTESIAN_POINT('Ctrl Pts',(-21.5050882576912,-3.10488082295939,
3.46887215836906));
#85239=CARTESIAN_POINT('Ctrl Pts',(-21.3641470331893,-4.0616166604905,1.05209408070949));
#85240=CARTESIAN_POINT('Ctrl Pts',(-21.3021873309261,-4.07120543337986,
-0.00357758459923137));
#85241=CARTESIAN_POINT('Origin',(-0.4,4.52129938221115E-16,0.));
#85242=CARTESIAN_POINT('',(-0.4,4.77615934004777,-1.20163511869221));
#85243=CARTESIAN_POINT('Ctrl Pts',(-0.399999999999999,-2.75232012058015,
-3.00608727173434));
#85244=CARTESIAN_POINT('Ctrl Pts',(-0.399999999999999,-2.67884530085595,
-3.08970388103118));
#85245=CARTESIAN_POINT('Ctrl Pts',(-0.399999999999998,-2.60192581722023,
-3.16993140988783));
#85246=CARTESIAN_POINT('Ctrl Pts',(-0.399999999999999,-2.52168473419593,
-3.24649039328315));
#85247=CARTESIAN_POINT('Ctrl Pts',(-0.4,-2.43283015801532,-3.33126761420314));
#85248=CARTESIAN_POINT('Ctrl Pts',(-0.399999999999997,-2.33990343083429,
-3.41154791660084));
#85249=CARTESIAN_POINT('Ctrl Pts',(-0.399999999999995,-2.24331760456818,
-3.48732708244347));
#85250=CARTESIAN_POINT('Ctrl Pts',(-0.399999999999994,-2.17934863242522,
-3.53751576473985));
#85251=CARTESIAN_POINT('Ctrl Pts',(-0.399999999999999,-2.11377364367761,
-3.5857294623203));
#85252=CARTESIAN_POINT('Ctrl Pts',(-0.4,-2.04670293396042,-3.63195924784765));
#85253=CARTESIAN_POINT('Ctrl Pts',(-0.4,-2.02167655430602,-3.64920916467166));
#85254=CARTESIAN_POINT('Ctrl Pts',(-0.400000000000003,-1.99644185707205,
-3.66618279846621));
#85255=CARTESIAN_POINT('Ctrl Pts',(-0.400000000000003,-1.97100433623467,
-3.68287944933743));
#85256=CARTESIAN_POINT('Ctrl Pts',(-0.400000000000003,-1.94833071868495,
-3.69776193252576));
#85257=CARTESIAN_POINT('Ctrl Pts',(-0.399999999999998,-1.92549295693954,
-3.71242611279588));
#85258=CARTESIAN_POINT('Ctrl Pts',(-0.399999999999998,-1.90251718347535,
-3.72685775571483));
#85259=CARTESIAN_POINT('Ctrl Pts',(-0.399999999999998,-1.79577386745123,
-3.79390583238766));
#85260=CARTESIAN_POINT('Ctrl Pts',(-0.400000000000007,-1.68596470474815,
-3.85599838796523));
#85261=CARTESIAN_POINT('Ctrl Pts',(-0.400000000000006,-1.57352241925111,
-3.91313343837503));
#85262=CARTESIAN_POINT('Ctrl Pts',(-0.400000000000006,-1.45755473669459,
-3.97205984101337));
#85263=CARTESIAN_POINT('Ctrl Pts',(-0.400000000000004,-1.33878571496281,
-4.02571347884009));
#85264=CARTESIAN_POINT('Ctrl Pts',(-0.400000000000004,-1.21764940630657,
-4.07405401109807));
#85265=CARTESIAN_POINT('Ctrl Pts',(-0.400000000000004,-1.16465227126946,
-4.09520299396094));
#85266=CARTESIAN_POINT('Ctrl Pts',(-0.4,-1.11120155664704,-4.11533448914209));
#85267=CARTESIAN_POINT('Ctrl Pts',(-0.4,-1.05733168943948,-4.13444256176185));
#85268=CARTESIAN_POINT('Ctrl Pts',(-0.4,-1.02977013518471,-4.14421886542683));
#85269=CARTESIAN_POINT('Ctrl Pts',(-0.400000000000004,-1.00209884390297,
-4.15372724442471));
#85270=CARTESIAN_POINT('Ctrl Pts',(-0.400000000000005,-0.974322331280067,
-4.16296673702109));
#85271=CARTESIAN_POINT('Ctrl Pts',(-0.400000000000005,-0.950830465098206,
-4.17078099817797));
#85272=CARTESIAN_POINT('Ctrl Pts',(-0.400000000000003,-0.927260172172898,
-4.1784038296046));
#85273=CARTESIAN_POINT('Ctrl Pts',(-0.400000000000003,-0.903638597056394,
-4.18582717574358));
#85274=CARTESIAN_POINT('Ctrl Pts',(-0.400000000000003,-0.777616734918826,
-4.22543096588513));
#85275=CARTESIAN_POINT('Ctrl Pts',(-0.400000000000009,-0.650003521738759,
-4.25940648821455));
#85276=CARTESIAN_POINT('Ctrl Pts',(-0.400000000000008,-0.521253026605198,
-4.28774813192643));
#85277=CARTESIAN_POINT('Ctrl Pts',(-0.400000000000007,-0.390643175835227,
-4.31649907266608));
#85278=CARTESIAN_POINT('Ctrl Pts',(-0.399999999999999,-0.258862245080765,
-4.33945261889705));
#85279=CARTESIAN_POINT('Ctrl Pts',(-0.4,-0.126350901762778,-4.35656076619393));
#85280=CARTESIAN_POINT('Ctrl Pts',(-0.4,0.00669532870704109,-4.3737379711877));
#85281=CARTESIAN_POINT('Ctrl Pts',(-0.400000000000008,0.140478697090108,
-4.38502282639319));
#85282=CARTESIAN_POINT('Ctrl Pts',(-0.400000000000009,0.274574911972207,
-4.39031924043944));
#85283=CARTESIAN_POINT('Ctrl Pts',(-0.40000000000001,0.375147073133782,
-4.39429155097413));
#85284=CARTESIAN_POINT('Ctrl Pts',(-0.400000000000009,0.475895739149746,
-4.39489441889364));
#85285=CARTESIAN_POINT('Ctrl Pts',(-0.40000000000001,0.576645629621254,
-4.39206814261951));
#85286=CARTESIAN_POINT('Ctrl Pts',(-0.40000000000001,0.621564747135451,
-4.39080805354654));
#85287=CARTESIAN_POINT('Ctrl Pts',(-0.400000000000001,0.666484127834017,
-4.38886609187459));
#85288=CARTESIAN_POINT('Ctrl Pts',(-0.400000000000001,0.711388257581674,
-4.38623584493183));
#85289=CARTESIAN_POINT('Ctrl Pts',(-0.4,0.729692703889777,-4.38516366706731));
#85290=CARTESIAN_POINT('Ctrl Pts',(-0.400000000000005,0.747994987199218,
-4.3839770260269));
#85291=CARTESIAN_POINT('Ctrl Pts',(-0.400000000000005,0.76627878126558,
-4.3826767175198));
#85292=CARTESIAN_POINT('Ctrl Pts',(-0.400000000000004,0.903799577305213,
-4.37289650120665));
#85293=CARTESIAN_POINT('Ctrl Pts',(-0.400000000000001,1.04048239370559,
-4.35667845015307));
#85294=CARTESIAN_POINT('Ctrl Pts',(-0.400000000000001,1.17587220890522,
-4.33397675466201));
#85295=CARTESIAN_POINT('Ctrl Pts',(-0.400000000000001,1.27545468382726,
-4.31727911002314));
#85296=CARTESIAN_POINT('Ctrl Pts',(-0.400000000000001,1.37433826386558,
-4.29707290664842));
#85297=CARTESIAN_POINT('Ctrl Pts',(-0.400000000000001,1.47234696797353,
-4.27332264316194));
#85298=CARTESIAN_POINT('Ctrl Pts',(-0.400000000000001,1.60147130364406,
-4.24203218766002));
#85299=CARTESIAN_POINT('Ctrl Pts',(-0.400000000000009,1.72907757991282,
-4.20459238895073));
#85300=CARTESIAN_POINT('Ctrl Pts',(-0.400000000000011,1.85486206446225,
-4.16133352902126));
#85301=CARTESIAN_POINT('Ctrl Pts',(-0.400000000000013,1.98260002701008,
-4.11740284353705));
#85302=CARTESIAN_POINT('Ctrl Pts',(-0.400000000000002,2.10845986782647,
-4.06747070160946));
#85303=CARTESIAN_POINT('Ctrl Pts',(-0.400000000000002,2.23211522018608,
-4.01182989632834));
#85304=CARTESIAN_POINT('Ctrl Pts',(-0.400000000000003,2.27057077740154,
-3.99452617165995));
#85305=CARTESIAN_POINT('Ctrl Pts',(-0.399999999999999,2.30881302678684,
-3.97666996889792));
#85306=CARTESIAN_POINT('Ctrl Pts',(-0.399999999999999,2.34683182515979,
-3.9582691309213));
#85307=CARTESIAN_POINT('Ctrl Pts',(-0.399999999999999,2.36665698110855,
-3.94867389124813));
#85308=CARTESIAN_POINT('Ctrl Pts',(-0.400000000000004,2.38642137382624,
-3.93893054872392));
#85309=CARTESIAN_POINT('Ctrl Pts',(-0.400000000000004,2.4061235432385,-3.92904016894681));
#85310=CARTESIAN_POINT('Ctrl Pts',(-0.400000000000004,2.42353838620782,
-3.92029801435859));
#85311=CARTESIAN_POINT('Ctrl Pts',(-0.399999999999997,2.44089803817829,
-3.91144424865044));
#85312=CARTESIAN_POINT('Ctrl Pts',(-0.399999999999997,2.45819532721275,
-3.90248319304769));
#85313=CARTESIAN_POINT('Ctrl Pts',(-0.399999999999998,2.5798934217451,-3.83943612308888));
#85314=CARTESIAN_POINT('Ctrl Pts',(-0.400000000000001,2.69860205934974,
-3.77103373158167));
#85315=CARTESIAN_POINT('Ctrl Pts',(-0.400000000000001,2.81401193712609,
-3.69765307721598));
#85316=CARTESIAN_POINT('Ctrl Pts',(-0.400000000000001,2.93213331951802,
-3.62254837646153));
#85317=CARTESIAN_POINT('Ctrl Pts',(-0.400000000000009,3.04679984508726,
-3.54222851204289));
#85318=CARTESIAN_POINT('Ctrl Pts',(-0.400000000000008,3.15767190543002,
-3.45704308422265));
#85319=CARTESIAN_POINT('Ctrl Pts',(-0.400000000000006,3.26771397659399,
-3.37249535523351));
#85320=CARTESIAN_POINT('Ctrl Pts',(-0.400000000000003,3.37401887476973,
-3.28315413650226));
#85321=CARTESIAN_POINT('Ctrl Pts',(-0.400000000000004,3.47623612856816,
-3.18931392989282));
#85322=CARTESIAN_POINT('Ctrl Pts',(-0.400000000000004,3.54991652696762,
-3.12167188755712));
#85323=CARTESIAN_POINT('Ctrl Pts',(-0.400000000000001,3.62147269323696,
-3.05169124259841));
#85324=CARTESIAN_POINT('Ctrl Pts',(-0.400000000000002,3.69082794584072,
-2.97947697283326));
#85325=CARTESIAN_POINT('Ctrl Pts',(-0.400000000000002,3.72117086885487,
-2.94788322981101));
#85326=CARTESIAN_POINT('Ctrl Pts',(-0.399999999999995,3.75109241135012,
-2.91586182386534));
#85327=CARTESIAN_POINT('Ctrl Pts',(-0.399999999999995,3.78058559715336,
-2.88342095501289));
#85328=CARTESIAN_POINT('Ctrl Pts',(-0.399999999999995,3.79948466987934,
-2.86263302305373));
#85329=CARTESIAN_POINT('Ctrl Pts',(-0.400000000000004,3.81820784472281,
-2.8416728452019));
#85330=CARTESIAN_POINT('Ctrl Pts',(-0.400000000000004,3.83675320660352,
-2.82054250757437));
#85331=CARTESIAN_POINT('Ctrl Pts',(-0.400000000000004,3.84994386245842,
-2.80551325047303));
#85332=CARTESIAN_POINT('Ctrl Pts',(-0.399999999999998,3.86303916500851,
-2.79040401859846));
#85333=CARTESIAN_POINT('Ctrl Pts',(-0.399999999999998,3.87603459396517,
-2.77522058695776));
#85334=CARTESIAN_POINT('Ctrl Pts',(-0.399999999999999,3.96865254349779,
-2.66700882187327));
#85335=CARTESIAN_POINT('Ctrl Pts',(-0.400000000000009,4.0562655215007,-2.55495685843537));
#85336=CARTESIAN_POINT('Ctrl Pts',(-0.400000000000009,4.13871251510199,
-2.43943448304065));
#85337=CARTESIAN_POINT('Ctrl Pts',(-0.400000000000009,4.22224141115088,
-2.32239617680077));
#85338=CARTESIAN_POINT('Ctrl Pts',(-0.400000000000003,4.30046841967742,
-2.20179534626246));
#85339=CARTESIAN_POINT('Ctrl Pts',(-0.400000000000003,4.37319725428977,
-2.07797192475027));
#85340=CARTESIAN_POINT('Ctrl Pts',(-0.400000000000002,4.44584600861285,
-1.954284842772));
#85341=CARTESIAN_POINT('Ctrl Pts',(-0.400000000000005,4.51300920794952,
-1.82738171523173));
#85342=CARTESIAN_POINT('Ctrl Pts',(-0.400000000000006,4.574454549482,-1.69756469246434));
#85343=CARTESIAN_POINT('Ctrl Pts',(-0.400000000000006,4.63508808389366,
-1.56946279375448));
#85344=CARTESIAN_POINT('Ctrl Pts',(-0.4,4.69015427300349,-1.43852290445209));
#85345=CARTESIAN_POINT('Ctrl Pts',(-0.4,4.73938732007769,-1.3050081252555));
#85346=CARTESIAN_POINT('Ctrl Pts',(-0.4,4.75203130269614,-1.27071899127353));
#85347=CARTESIAN_POINT('Ctrl Pts',(-0.4,4.76429031498248,-1.23625991144432));
#85348=CARTESIAN_POINT('Ctrl Pts',(-0.4,4.77615934004777,-1.20163511869221));
#85349=CARTESIAN_POINT('',(-0.4,-6.03138548580071E-16,4.925));
#85350=CARTESIAN_POINT('Origin',(-0.4,0.,0.));
#85351=CARTESIAN_POINT('',(-0.4,3.87692992261799,3.04758435726506));
#85352=CARTESIAN_POINT('Origin',(-0.4,0.,0.));
#85353=CARTESIAN_POINT('Ctrl Pts',(-0.400000000000003,3.87692992261803,
3.04758435726501));
#85354=CARTESIAN_POINT('Ctrl Pts',(-0.400000000000002,3.7866811565513,3.14569047611427));
#85355=CARTESIAN_POINT('Ctrl Pts',(-0.400000000000005,3.69239500566201,
3.23969491248585));
#85356=CARTESIAN_POINT('Ctrl Pts',(-0.400000000000002,3.59413579950762,
3.32924783641162));
#85357=CARTESIAN_POINT('Ctrl Pts',(-0.4,3.48778565756658,3.42617479667806));
#85358=CARTESIAN_POINT('Ctrl Pts',(-0.399999999999996,3.37678079498109,
3.51788765012915));
#85359=CARTESIAN_POINT('Ctrl Pts',(-0.399999999999994,3.2615705131932,3.60429059305081));
#85360=CARTESIAN_POINT('Ctrl Pts',(-0.399999999999993,3.19124267296232,
3.65703356243664));
#85361=CARTESIAN_POINT('Ctrl Pts',(-0.399999999999997,3.11934726363608,
3.70779701613254));
#85362=CARTESIAN_POINT('Ctrl Pts',(-0.399999999999996,3.04598312559039,
3.75655034537377));
#85363=CARTESIAN_POINT('Ctrl Pts',(-0.399999999999996,3.00363685050327,
3.78469109569754));
#85364=CARTESIAN_POINT('Ctrl Pts',(-0.399999999999999,2.96080120507407,
3.81216201228181));
#85365=CARTESIAN_POINT('Ctrl Pts',(-0.399999999999999,2.9174949863662,3.83895616530978));
#85366=CARTESIAN_POINT('Ctrl Pts',(-0.4,2.89770430810063,3.85120093009869));
#85367=CARTESIAN_POINT('Ctrl Pts',(-0.400000000000002,2.87781497051338,
3.86330449470594));
#85368=CARTESIAN_POINT('Ctrl Pts',(-0.400000000000001,2.85784196930167,
3.87525848021691));
#85369=CARTESIAN_POINT('Ctrl Pts',(-0.4,2.73551505654073,3.94847202119883));
#85370=CARTESIAN_POINT('Ctrl Pts',(-0.400000000000002,2.60993309562182,
4.01615280664636));
#85371=CARTESIAN_POINT('Ctrl Pts',(-0.400000000000003,2.48153782508233,
4.07821468153474));
#85372=CARTESIAN_POINT('Ctrl Pts',(-0.400000000000004,2.35692693580737,
4.13844731617477));
#85373=CARTESIAN_POINT('Ctrl Pts',(-0.4,2.22966530561295,4.19338727339985));
#85374=CARTESIAN_POINT('Ctrl Pts',(-0.399999999999998,2.10014532784416,
4.24291112487635));
#85375=CARTESIAN_POINT('Ctrl Pts',(-0.399999999999998,2.03971372870769,
4.26601802770075));
#85376=CARTESIAN_POINT('Ctrl Pts',(-0.400000000000003,1.97879040175326,
4.28794521994513));
#85377=CARTESIAN_POINT('Ctrl Pts',(-0.400000000000004,1.91741505878211,
4.30867678401833));
#85378=CARTESIAN_POINT('Ctrl Pts',(-0.400000000000004,1.88122280084346,
4.32090192326947));
#85379=CARTESIAN_POINT('Ctrl Pts',(-0.399999999999999,1.84487336389223,
4.33271126438745));
#85380=CARTESIAN_POINT('Ctrl Pts',(-0.399999999999999,1.8083749234927,4.34410118547454));
#85381=CARTESIAN_POINT('Ctrl Pts',(-0.399999999999999,1.7905238413653,4.34967190067565));
#85382=CARTESIAN_POINT('Ctrl Pts',(-0.399999999999998,1.77263621214053,
4.35514255273796));
#85383=CARTESIAN_POINT('Ctrl Pts',(-0.399999999999998,1.75471579018526,
4.36051185834341));
#85384=CARTESIAN_POINT('Ctrl Pts',(-0.399999999999997,1.61980899273671,
4.40093254852367));
#85385=CARTESIAN_POINT('Ctrl Pts',(-0.399999999999992,1.48344756261164,
4.4354938576941));
#85386=CARTESIAN_POINT('Ctrl Pts',(-0.399999999999992,1.34604936009094,
4.4641147523174));
#85387=CARTESIAN_POINT('Ctrl Pts',(-0.399999999999992,1.20915742171099,
4.49263018899178));
#85388=CARTESIAN_POINT('Ctrl Pts',(-0.399999999999996,1.07123549650562,
4.51524897193337));
#85389=CARTESIAN_POINT('Ctrl Pts',(-0.399999999999997,0.932692055242528,
4.53183975365004));
#85390=CARTESIAN_POINT('Ctrl Pts',(-0.399999999999998,0.791946814713625,
4.54869420408079));
#85391=CARTESIAN_POINT('Ctrl Pts',(-0.399999999999994,0.650559268185746,
4.55932778291634));
#85392=CARTESIAN_POINT('Ctrl Pts',(-0.399999999999993,0.508965718232696,
4.56354719544793));
#85393=CARTESIAN_POINT('Ctrl Pts',(-0.399999999999993,0.402770555767909,
4.56671175484662));
#85394=CARTESIAN_POINT('Ctrl Pts',(-0.400000000000001,0.296459603189304,
4.5662672082447));
#85395=CARTESIAN_POINT('Ctrl Pts',(-0.400000000000002,0.190224357752561,
4.56211075806113));
#85396=CARTESIAN_POINT('Ctrl Pts',(-0.400000000000002,0.149138750040393,
4.56050328512674));
#85397=CARTESIAN_POINT('Ctrl Pts',(-0.4,0.108064552956015,4.5583404300336));
#85398=CARTESIAN_POINT('Ctrl Pts',(-0.4,0.0670132119983308,4.55561550073097));
#85399=CARTESIAN_POINT('Ctrl Pts',(-0.4,0.0389733158602479,4.55375425252697));
#85400=CARTESIAN_POINT('Ctrl Pts',(-0.400000000000004,0.0109440877756324,
4.55163075999061));
#85401=CARTESIAN_POINT('Ctrl Pts',(-0.400000000000004,-0.017070759942624,
4.54924277763623));
#85402=CARTESIAN_POINT('Ctrl Pts',(-0.400000000000004,-0.0352366249698258,
4.54769432141853));
#85403=CARTESIAN_POINT('Ctrl Pts',(-0.400000000000003,-0.0533870669854209,
4.5460354437308));
#85404=CARTESIAN_POINT('Ctrl Pts',(-0.400000000000003,-0.0715190897426694,
4.5442660769587));
#85405=CARTESIAN_POINT('Ctrl Pts',(-0.400000000000003,-0.204503034352091,
4.53128918100152));
#85406=CARTESIAN_POINT('Ctrl Pts',(-0.400000000000005,-0.336533808014188,
4.51236994685749));
#85407=CARTESIAN_POINT('Ctrl Pts',(-0.400000000000005,-0.467248957372364,
4.48738348767377));
#85408=CARTESIAN_POINT('Ctrl Pts',(-0.400000000000005,-0.563130622195358,
4.4690555179141));
#85409=CARTESIAN_POINT('Ctrl Pts',(-0.400000000000008,-0.658304353226521,
4.44746208615338));
#85410=CARTESIAN_POINT('Ctrl Pts',(-0.400000000000007,-0.752621900496299,
4.42253677366799));
#85411=CARTESIAN_POINT('Ctrl Pts',(-0.400000000000006,-0.882855492363467,
4.38811992264345));
#85412=CARTESIAN_POINT('Ctrl Pts',(-0.399999999999997,-1.01145813828583,
4.34735181884672));
#85413=CARTESIAN_POINT('Ctrl Pts',(-0.399999999999995,-1.13804025543659,
4.30050936743311));
#85414=CARTESIAN_POINT('Ctrl Pts',(-0.399999999999993,-1.26429577728981,
4.25378777451596));
#85415=CARTESIAN_POINT('Ctrl Pts',(-0.40000000000001,-1.38854185763495,
4.20102250581896));
#85416=CARTESIAN_POINT('Ctrl Pts',(-0.40000000000001,-1.51035703949907,
4.14245041098922));
#85417=CARTESIAN_POINT('Ctrl Pts',(-0.40000000000001,-1.55643596961048,
4.12029439215119));
#85418=CARTESIAN_POINT('Ctrl Pts',(-0.400000000000005,-1.60216665890396,
4.09730714941568));
#85419=CARTESIAN_POINT('Ctrl Pts',(-0.400000000000005,-1.64752468421034,
4.07350036769371));
#85420=CARTESIAN_POINT('Ctrl Pts',(-0.400000000000005,-1.66484982409097,
4.06440703039221));
#85421=CARTESIAN_POINT('Ctrl Pts',(-0.400000000000003,-1.68212182349379,
4.05519337578249));
#85422=CARTESIAN_POINT('Ctrl Pts',(-0.400000000000003,-1.69932318947039,
4.04586897304114));
#85423=CARTESIAN_POINT('Ctrl Pts',(-0.400000000000004,-1.81540496360726,
3.98294413239445));
#85424=CARTESIAN_POINT('Ctrl Pts',(-0.399999999999996,-1.92844024788491,
3.91489260676169));
#85425=CARTESIAN_POINT('Ctrl Pts',(-0.399999999999998,-2.03808463169202,
3.84200800987513));
#85426=CARTESIAN_POINT('Ctrl Pts',(-0.399999999999999,-2.14729220487318,
3.76941377684746));
#85427=CARTESIAN_POINT('Ctrl Pts',(-0.400000000000001,-2.25313646136716,
3.69202425594331));
#85428=CARTESIAN_POINT('Ctrl Pts',(-0.400000000000001,-2.35524312129288,
3.61009135281258));
#85429=CARTESIAN_POINT('Ctrl Pts',(-0.400000000000001,-2.45294910305158,
3.53168966241793));
#85430=CARTESIAN_POINT('Ctrl Pts',(-0.400000000000005,-2.54723297607989,
3.4491270787068));
#85431=CARTESIAN_POINT('Ctrl Pts',(-0.400000000000005,-2.63772970486551,
3.36259935817761));
#85432=CARTESIAN_POINT('Ctrl Pts',(-0.400000000000005,-2.70045032911986,
3.30262953695066));
#85433=CARTESIAN_POINT('Ctrl Pts',(-0.400000000000001,-2.76135096672307,
3.2407545396391));
#85434=CARTESIAN_POINT('Ctrl Pts',(-0.400000000000001,-2.82034722332256,
3.17704902576884));
#85435=CARTESIAN_POINT('Ctrl Pts',(-0.400000000000001,-2.84998809096459,
3.14504213561113));
#85436=CARTESIAN_POINT('Ctrl Pts',(-0.400000000000005,-2.8791480950544,
3.11257312640867));
#85437=CARTESIAN_POINT('Ctrl Pts',(-0.400000000000005,-2.90781559435835,
3.07965121601423));
#85438=CARTESIAN_POINT('Ctrl Pts',(-0.400000000000005,-2.92363627213933,
3.06148266455593));
#85439=CARTESIAN_POINT('Ctrl Pts',(-0.400000000000008,-2.93930694212779,
3.04317617572848));
#85440=CARTESIAN_POINT('Ctrl Pts',(-0.400000000000008,-2.95482556230634,
3.02473328303618));
#85441=CARTESIAN_POINT('Ctrl Pts',(-0.400000000000008,-2.96600453499757,
3.01144778526754));
#85442=CARTESIAN_POINT('Ctrl Pts',(-0.400000000000003,-2.97710217566663,
2.99809433168513));
#85443=CARTESIAN_POINT('Ctrl Pts',(-0.400000000000003,-2.98811180444513,
2.98468107674361));
#85444=CARTESIAN_POINT('Ctrl Pts',(-0.400000000000003,-3.07107784142571,
2.88360186436529));
#85445=CARTESIAN_POINT('Ctrl Pts',(-0.400000000000007,-3.14915436767407,
2.77900529093076));
#85446=CARTESIAN_POINT('Ctrl Pts',(-0.400000000000006,-3.22213021391048,
2.67119388412099));
#85447=CARTESIAN_POINT('Ctrl Pts',(-0.400000000000005,-3.2932206471212,
2.56616790620585));
#85448=CARTESIAN_POINT('Ctrl Pts',(-0.4,-3.35947070624474,2.45809028694776));
#85449=CARTESIAN_POINT('Ctrl Pts',(-0.399999999999998,-3.42063827617722,
2.34721892088016));
#85450=CARTESIAN_POINT('Ctrl Pts',(-0.399999999999997,-3.48423921431184,
2.23193687024534));
#85451=CARTESIAN_POINT('Ctrl Pts',(-0.400000000000001,-3.54234599826298,
2.11363372392856));
#85452=CARTESIAN_POINT('Ctrl Pts',(-0.400000000000001,-3.59462745933778,
1.99258608284811));
#85453=CARTESIAN_POINT('Ctrl Pts',(-0.400000000000002,-3.64331564762821,
1.87985797196755));
#85454=CARTESIAN_POINT('Ctrl Pts',(-0.399999999999998,-3.68695142065924,
1.76474903921935));
#85455=CARTESIAN_POINT('Ctrl Pts',(-0.399999999999998,-3.72521579217317,
1.64748078441541));
#85456=CARTESIAN_POINT('Ctrl Pts',(-0.399999999999998,-3.728039769191,1.63882618371547));
#85457=CARTESIAN_POINT('Ctrl Pts',(-0.4,-3.73083446619856,1.63015982325057));
#85458=CARTESIAN_POINT('Ctrl Pts',(-0.4,-3.73359974356525,1.62148179294418));
#85459=CARTESIAN_POINT('Ctrl Pts',(-24.5683458050225,-1.79217368492185,
3.6547344271607));
#85460=CARTESIAN_POINT('Ctrl Pts',(-24.5288550439032,-2.39673442057434,
3.3582757205249));
#85461=CARTESIAN_POINT('Ctrl Pts',(-24.4498735216646,-3.44699120888544,
2.45967327826949));
#85462=CARTESIAN_POINT('Ctrl Pts',(-24.2919104771873,-4.48175779295681,
-0.129924271761729));
#85463=CARTESIAN_POINT('Ctrl Pts',(-24.0944566715907,-3.10076527220938,
-3.66761492221252));
#85464=CARTESIAN_POINT('Ctrl Pts',(-23.8575121048748,1.38408548988815,-4.60175935722059));
#85465=CARTESIAN_POINT('Ctrl Pts',(-23.6205675381589,4.60615095363263,-1.3559766287573));
#85466=CARTESIAN_POINT('Ctrl Pts',(-23.383622971443,3.65518318625674,3.11589977766662));
#85467=CARTESIAN_POINT('Ctrl Pts',(-23.1466784047271,-0.612424310989975,
4.764040620714));
#85468=CARTESIAN_POINT('Ctrl Pts',(-22.9097338380112,-4.32361166112413,
2.09108995787177));
#85469=CARTESIAN_POINT('Ctrl Pts',(-22.6727892712952,-4.11460291030966,
-2.47761200147492));
#85470=CARTESIAN_POINT('Ctrl Pts',(-22.4358447045794,-0.174092888986568,
-4.79981806178492));
#85471=CARTESIAN_POINT('Ctrl Pts',(-22.1989001378634,3.92413894310881,-2.76930725388711));
#85472=CARTESIAN_POINT('Ctrl Pts',(-21.9619555711476,4.46395155275901,1.77240342487198));
#85473=CARTESIAN_POINT('Ctrl Pts',(-21.7250110044316,0.955712424786761,
4.70689540849193));
#85474=CARTESIAN_POINT('Ctrl Pts',(-21.4880664377158,-3.4191670361001,3.37305028818365));
#85475=CARTESIAN_POINT('Ctrl Pts',(-21.2511218709998,-4.69348025162024,
-1.01954248977653));
#85476=CARTESIAN_POINT('Ctrl Pts',(-21.0141773042839,-1.71163476880105,
-4.48759644703182));
#85477=CARTESIAN_POINT('Ctrl Pts',(-20.777232737568,2.82235647137499,-3.88619479158027));
#85478=CARTESIAN_POINT('Ctrl Pts',(-20.5402881708521,4.79697321791449,0.239293923164062));
#85479=CARTESIAN_POINT('Ctrl Pts',(-20.3033436041362,2.42158643669063,4.14778627515724));
#85480=CARTESIAN_POINT('Ctrl Pts',(-20.0663990374203,-2.14974872645911,
4.2949727839084));
#85481=CARTESIAN_POINT('Ctrl Pts',(-19.8294544707044,-4.77164382869297,
0.547382001344689));
#85482=CARTESIAN_POINT('Ctrl Pts',(-19.5925099039885,-3.06650535307055,
-3.69658713851903));
#85483=CARTESIAN_POINT('Ctrl Pts',(-19.3555653372726,1.4194087785671,-4.58840823893679));
#85484=CARTESIAN_POINT('Ctrl Pts',(-19.1186207705567,4.61817127913257,-1.31935803851751));
#85485=CARTESIAN_POINT('Ctrl Pts',(-18.8816762038408,3.62907264384353,3.14611558694568));
#85486=CARTESIAN_POINT('Ctrl Pts',(-18.6447316371248,-0.650950313849541,
4.75862114706335));
#85487=CARTESIAN_POINT('Ctrl Pts',(-18.407787070409,-4.34067695608756,2.05590250627856));
#85488=CARTESIAN_POINT('Ctrl Pts',(-18.170842503693,-4.09418054167253,-2.51115456224217));
#85489=CARTESIAN_POINT('Ctrl Pts',(-17.9338979369771,-0.134989541855146,
-4.801040446262));
#85490=CARTESIAN_POINT('Ctrl Pts',(-17.6969533702612,3.94661299763452,-2.73723535571292));
#85491=CARTESIAN_POINT('Ctrl Pts',(-17.4600088035453,4.44933850329186,1.80875604418168));
#85492=CARTESIAN_POINT('Ctrl Pts',(-17.2230642368294,0.917304230718045,
4.71452696382671));
#85493=CARTESIAN_POINT('Ctrl Pts',(-16.9861196701135,-3.44656205740185,
3.34505927139524));
#85494=CARTESIAN_POINT('Ctrl Pts',(-16.7491751033976,-4.6850087010358,-1.05778306645274));
#85495=CARTESIAN_POINT('Ctrl Pts',(-16.5122305366817,-1.67498455417103,
-4.50140403516247));
#85496=CARTESIAN_POINT('Ctrl Pts',(-16.2752859699658,2.85395309043288,-3.86305103540403));
#85497=CARTESIAN_POINT('Ctrl Pts',(-16.0383414032499,4.79486217074114,0.278403139515235));
#85498=CARTESIAN_POINT('Ctrl Pts',(-15.801396836534,2.38768287451035,4.16739511388991));
#85499=CARTESIAN_POINT('Ctrl Pts',(-15.5644522698181,-2.18470071411643,
4.27729988827614));
#85500=CARTESIAN_POINT('Ctrl Pts',(-15.3275077031021,-4.77594877829719,
0.508453352418028));
#85501=CARTESIAN_POINT('Ctrl Pts',(-15.0905631363863,-3.03625955368752,
-3.72147006801695));
#85502=CARTESIAN_POINT('Ctrl Pts',(-14.8536185696703,1.45677781805249,-4.57668110461451));
#85503=CARTESIAN_POINT('Ctrl Pts',(-14.6166740029544,4.62877644616991,-1.28165524065066));
#85504=CARTESIAN_POINT('Ctrl Pts',(-14.3797294362385,3.60329695155474,3.17560429263805));
#85505=CARTESIAN_POINT('Ctrl Pts',(-14.1427848695226,-0.689732898916454,
4.75315474949608));
#85506=CARTESIAN_POINT('Ctrl Pts',(-13.9058403028067,-4.35729751307742,
2.02043805325335));
#85507=CARTESIAN_POINT('Ctrl Pts',(-13.6688957360908,-4.07356717962569,
-2.54445710861498));
#85508=CARTESIAN_POINT('Ctrl Pts',(-13.4319511693749,-0.0958349178438527,
-4.80198159232485));
#85509=CARTESIAN_POINT('Ctrl Pts',(-13.195006602659,3.96880259324556,-2.70496164859175));
#85510=CARTESIAN_POINT('Ctrl Pts',(-12.9580620359431,4.43444104868229,1.84497808395286));
#85511=CARTESIAN_POINT('Ctrl Pts',(-12.7211174692272,0.878829071125367,
4.72185037969754));
#85512=CARTESIAN_POINT('Ctrl Pts',(-12.4841729025113,-3.47372478568834,
3.31684302580018));
#85513=CARTESIAN_POINT('Ctrl Pts',(-12.2472283357954,-4.67622722785964,
-1.09595185018732));
#85514=CARTESIAN_POINT('Ctrl Pts',(-12.0102837690795,-1.63822211600786,
-4.514913049343));
#85515=CARTESIAN_POINT('Ctrl Pts',(-11.7733392023635,2.88535949150936,-3.83965000348491));
#85516=CARTESIAN_POINT('Ctrl Pts',(-11.5363946356477,4.79243250703115,0.317493637819545));
#85517=CARTESIAN_POINT('Ctrl Pts',(-11.2994500689317,2.35362041946459,4.18672693945812));
#85518=CARTESIAN_POINT('Ctrl Pts',(-11.0625055022158,-2.21950736358003,
4.25934250882913));
#85519=CARTESIAN_POINT('Ctrl Pts',(-10.8255609354999,-4.77993617310215,
0.469490921716715));
#85520=CARTESIAN_POINT('Ctrl Pts',(-10.588616368784,-3.00581183494387,-3.74610554541864));
#85521=CARTESIAN_POINT('Ctrl Pts',(-10.3516718020681,1.49404997724334,-4.56464962620395));
#85522=CARTESIAN_POINT('Ctrl Pts',(-10.1147272353522,4.63907381730574,-1.24386722044341));
#85523=CARTESIAN_POINT('Ctrl Pts',(-9.8777826686363,3.57728164792448,3.20488183181962));
#85524=CARTESIAN_POINT('Ctrl Pts',(-9.64083810192037,-0.728469617480856,
4.74737227957853));
#85525=CARTESIAN_POINT('Ctrl Pts',(-9.40389353520448,-4.37362832284165,
1.9848392474317));
#85526=CARTESIAN_POINT('Ctrl Pts',(-9.16694896848857,-4.05268293663714,
-2.5775904561419));
#85527=CARTESIAN_POINT('Ctrl Pts',(-8.93000440177266,-0.0566739212580544,
-4.80260342014054));
#85528=CARTESIAN_POINT('Ctrl Pts',(-8.69305983505675,3.99072827488727,-2.67250806931295));
#85529=CARTESIAN_POINT('Ctrl Pts',(-8.45611526834084,4.41924871633079,1.88107743798526));
#85530=CARTESIAN_POINT('Ctrl Pts',(-8.21917070162494,0.840295471934814,
4.72885980594699));
#85531=CARTESIAN_POINT('Ctrl Pts',(-7.98222613490903,-3.50065652120147,
3.28840621962052));
#85532=CARTESIAN_POINT('Ctrl Pts',(-7.74528156819312,-4.66713479887029,
-1.13404775627675));
#85533=CARTESIAN_POINT('Ctrl Pts',(-7.50833700147722,-1.60135074079071,
-4.52812183462507));
#85534=CARTESIAN_POINT('Ctrl Pts',(-7.2713924347613,2.91657402449002,-3.81599364587164));
#85535=CARTESIAN_POINT('Ctrl Pts',(-7.03444786804541,4.78968416005308,0.356563023868872));
#85536=CARTESIAN_POINT('Ctrl Pts',(-6.79750330132949,2.31940145568391,4.2057803592973));
#85537=CARTESIAN_POINT('Ctrl Pts',(-6.5605587346136,-2.25416642273435,4.24110189585783));
#85538=CARTESIAN_POINT('Ctrl Pts',(-6.32361416789768,-4.78360571461287,
0.430497270029063));
#85539=CARTESIAN_POINT('Ctrl Pts',(-6.08666960118177,-2.9751642405108,-3.77049191521503));
#85540=CARTESIAN_POINT('Ctrl Pts',(-5.84972503446587,1.53122279065449,-4.55231461594934));
#85541=CARTESIAN_POINT('Ctrl Pts',(-5.61278046774996,4.6490626950213,-1.20599647826086));
#85542=CARTESIAN_POINT('Ctrl Pts',(-5.37583590103405,3.55102848107464,3.23394623945287));
#85543=CARTESIAN_POINT('Ctrl Pts',(-5.13889133431815,-0.767157925271441,
4.74127415374739));
#85544=CARTESIAN_POINT('Ctrl Pts',(-4.90194676760223,-4.38966824042904,
1.9491083962661));
#85545=CARTESIAN_POINT('Ctrl Pts',(-4.66500220088633,-4.03152931388751,
-2.61055228754619));
#85546=CARTESIAN_POINT('Ctrl Pts',(-4.42805763417042,-0.0175089406698063,
-4.80290610693659));
#85547=CARTESIAN_POINT('Ctrl Pts',(-4.19111306745452,4.01238817079558,-2.63987635628594));
#85548=CARTESIAN_POINT('Ctrl Pts',(-3.9541685007386,4.40376331119336,1.91705089973334));
#85549=CARTESIAN_POINT('Ctrl Pts',(-3.71722393402271,0.801704468977416,
4.73555632478705));
#85550=CARTESIAN_POINT('Ctrl Pts',(-3.48027936730679,-3.5273525406531,3.25974776958548));
#85551=CARTESIAN_POINT('Ctrl Pts',(-3.24333480059089,-4.6577376517205,-1.17206253805825));
#85552=CARTESIAN_POINT('Ctrl Pts',(-3.00639023387498,-1.56436205950543,
-4.54104048789013));
#85553=CARTESIAN_POINT('Ctrl Pts',(-2.76944566715907,2.94757382720121,-3.79206245260455));
#85554=CARTESIAN_POINT('Ctrl Pts',(-2.53250110044317,4.78665724274367,0.395568199836796));
#85555=CARTESIAN_POINT('Ctrl Pts',(-2.29555653372726,2.28495155387725,4.2246319053635));
#85556=CARTESIAN_POINT('Ctrl Pts',(-2.05861196701135,-2.28852823748934,
4.22242981165284));
#85557=CARTESIAN_POINT('Ctrl Pts',(-1.82166740029544,-4.7872402315289,0.391762093796413));
#85558=CARTESIAN_POINT('Ctrl Pts',(-1.58472283357954,-2.9437748544915,-3.79517919940816));
#85559=CARTESIAN_POINT('Ctrl Pts',(-1.34777826686363,1.56724719957269,-4.53861602703052));
#85560=CARTESIAN_POINT('Ctrl Pts',(-1.11083370014772,4.66076829913842,-1.17009430681153));
#85561=CARTESIAN_POINT('Ctrl Pts',(-0.873889133431818,3.52050501373642,
3.26683163619313));
#85562=CARTESIAN_POINT('Ctrl Pts',(-0.676435327835224,-0.0771870156949762,
4.48297617612786));
#85563=CARTESIAN_POINT('Ctrl Pts',(-0.518472283357957,-2.61623498089622,
3.32972304474434));
#85564=CARTESIAN_POINT('Ctrl Pts',(-0.439490761119318,-3.46537663594235,
2.23908831199168));
#85565=CARTESIAN_POINT('Ctrl Pts',(-0.4,-3.73359974356525,1.62148179294418));
#85566=CARTESIAN_POINT('Ctrl Pts',(-24.4038972033484,-1.91758108071806,
3.91047455474609));
#85567=CARTESIAN_POINT('Ctrl Pts',(-24.364406442229,-2.56444596808124,3.59327114313381));
#85568=CARTESIAN_POINT('Ctrl Pts',(-24.2854249199904,-3.68819449988101,
2.63178897382545));
#85569=CARTESIAN_POINT('Ctrl Pts',(-24.1274618755131,-4.7953689000347,-0.139015725737088));
#85570=CARTESIAN_POINT('Ctrl Pts',(-23.9300080699165,-3.31774139513474,
-3.92425636274236));
#85571=CARTESIAN_POINT('Ctrl Pts',(-23.6930635032006,1.4809369046291,-4.9237675765831));
#85572=CARTESIAN_POINT('Ctrl Pts',(-23.4561189364847,4.92846647505743,-1.4508611252789));
#85573=CARTESIAN_POINT('Ctrl Pts',(-23.2191743697688,3.91095471577045,3.33393493796763));
#85574=CARTESIAN_POINT('Ctrl Pts',(-22.9822298030529,-0.65527871657001,
5.09740447531009));
#85575=CARTESIAN_POINT('Ctrl Pts',(-22.745285236337,-4.62615648890371,2.23741402690521));
#85576=CARTESIAN_POINT('Ctrl Pts',(-22.5083406696211,-4.40252234583026,
-2.65098295960946));
#85577=CARTESIAN_POINT('Ctrl Pts',(-22.2713961029052,-0.18627504299217,
-5.13568544366227));
#85578=CARTESIAN_POINT('Ctrl Pts',(-22.0344515361893,4.19873065804033,-2.96308959417674));
#85579=CARTESIAN_POINT('Ctrl Pts',(-21.7975069694734,4.77631666775984,1.89642739625574));
#85580=CARTESIAN_POINT('Ctrl Pts',(-21.5605624027575,1.02258842421195,5.03626052551738));
#85581=CARTESIAN_POINT('Ctrl Pts',(-21.3236178360416,-3.65842332994994,
3.60907956151234));
#85582=CARTESIAN_POINT('Ctrl Pts',(-21.0866732693257,-5.02190664272777,
-1.09088499950208));
#85583=CARTESIAN_POINT('Ctrl Pts',(-20.8497287026098,-1.83140645204561,
-4.80161611406605));
#85584=CARTESIAN_POINT('Ctrl Pts',(-20.6127841358938,3.01985093190725,-4.15813136361528));
#85585=CARTESIAN_POINT('Ctrl Pts',(-20.375839569178,5.13264153177503,0.256038521071223));
#85586=CARTESIAN_POINT('Ctrl Pts',(-20.138895002462,2.59103700461042,4.43802771741427));
#85587=CARTESIAN_POINT('Ctrl Pts',(-19.9019504357462,-2.30017744420541,
4.59551360558059));
#85588=CARTESIAN_POINT('Ctrl Pts',(-19.6650058690302,-5.10553971794639,
0.58568506977604));
#85589=CARTESIAN_POINT('Ctrl Pts',(-19.4280613023143,-3.28108413734759,
-3.95525591056704));
#85590=CARTESIAN_POINT('Ctrl Pts',(-19.1911167355984,1.51873194126499,-4.90948221348304));
#85591=CARTESIAN_POINT('Ctrl Pts',(-18.9541721688825,4.94132792311723,-1.41168014832495));
#85592=CARTESIAN_POINT('Ctrl Pts',(-18.7172276021666,3.88301708753714,3.36626509921239));
#85593=CARTESIAN_POINT('Ctrl Pts',(-18.4802830354507,-0.696500577386702,
5.09160577386314));
#85594=CARTESIAN_POINT('Ctrl Pts',(-18.2433384687348,-4.64441592828398,
2.19976433255833));
#85595=CARTESIAN_POINT('Ctrl Pts',(-18.0063939020189,-4.38067092146694,
-2.68687266185611));
#85596=CARTESIAN_POINT('Ctrl Pts',(-17.769449335303,-0.144435438224605,
-5.1369933645219));
#85597=CARTESIAN_POINT('Ctrl Pts',(-17.532504768587,4.2227773350606,-2.92877346417273));
#85598=CARTESIAN_POINT('Ctrl Pts',(-17.2955602018711,4.76068106981219,1.9353237909575));
#85599=CARTESIAN_POINT('Ctrl Pts',(-17.0586156351552,0.981492615859015,
5.04442609911638));
#85600=CARTESIAN_POINT('Ctrl Pts',(-16.8216710684393,-3.68773531851224,
3.57912987266515));
#85601=CARTESIAN_POINT('Ctrl Pts',(-16.5847265017234,-5.01284229519173,
-1.13180146143153));
#85602=CARTESIAN_POINT('Ctrl Pts',(-16.3477819350075,-1.79219163778398,
-4.81638988850122));
#85603=CARTESIAN_POINT('Ctrl Pts',(-16.1108373682916,3.0536585251276,-4.13336812255573));
#85604=CARTESIAN_POINT('Ctrl Pts',(-15.8738928015757,5.13038276402602,0.297884405757334));
#85605=CARTESIAN_POINT('Ctrl Pts',(-15.6369482348598,2.55476103986837,4.45900868509891));
#85606=CARTESIAN_POINT('Ctrl Pts',(-15.4000036681439,-2.33757519802194,
4.57660404866038));
#85607=CARTESIAN_POINT('Ctrl Pts',(-15.163059101428,-5.11014590650051,0.544032387724225));
#85608=CARTESIAN_POINT('Ctrl Pts',(-14.9261145347121,-3.24872188744064,
-3.98188002364241));
#85609=CARTESIAN_POINT('Ctrl Pts',(-14.6891699679962,1.55871588016816,-4.89693447266046));
#85610=CARTESIAN_POINT('Ctrl Pts',(-14.4522254012803,4.95267518696769,-1.37133909628972));
#85611=CARTESIAN_POINT('Ctrl Pts',(-14.2152808345644,3.85543774057359,3.39781727777984));
#85612=CARTESIAN_POINT('Ctrl Pts',(-13.9783362678484,-0.737996974756748,
5.08575686499741));
#85613=CARTESIAN_POINT('Ctrl Pts',(-13.7413917011325,-4.66219950914051,
2.16181825359773));
#85614=CARTESIAN_POINT('Ctrl Pts',(-13.5044471344166,-4.35861513892556,
-2.7225055546954));
#85615=CARTESIAN_POINT('Ctrl Pts',(-13.2675025677007,-0.102540968476285,
-5.13800036730267));
#85616=CARTESIAN_POINT('Ctrl Pts',(-13.0305580009848,4.24651964814693,-2.89424140363592));
#85617=CARTESIAN_POINT('Ctrl Pts',(-12.7936134342689,4.74474116546558,1.97408046881445));
#85618=CARTESIAN_POINT('Ctrl Pts',(-12.556668867553,0.940325156068005,5.05226197118519));
#85619=CARTESIAN_POINT('Ctrl Pts',(-12.3197243008371,-3.71679875935009,
3.54893919462028));
#85620=CARTESIAN_POINT('Ctrl Pts',(-12.0827797341212,-5.00344633822333,
-1.17264110670656));
#85621=CARTESIAN_POINT('Ctrl Pts',(-11.8458351674053,-1.75285674714482,
-4.83084419626708));
#85622=CARTESIAN_POINT('Ctrl Pts',(-11.6088906006894,3.08726258985882,-4.10832960287713));
#85623=CARTESIAN_POINT('Ctrl Pts',(-11.3719460339735,5.12778308454073,0.33971026260081));
#85624=CARTESIAN_POINT('Ctrl Pts',(-11.1350014672576,2.51831506372883,4.47969325561639));
#85625=CARTESIAN_POINT('Ctrl Pts',(-10.8980569005416,-2.37481744360122,
4.55739010116378));
#85626=CARTESIAN_POINT('Ctrl Pts',(-10.6611123338258,-5.11441231935083,
0.502343560017281));
#85627=CARTESIAN_POINT('Ctrl Pts',(-10.4241677671098,-3.21614358886106,
-4.00823936915529));
#85628=CARTESIAN_POINT('Ctrl Pts',(-10.1872232003939,1.59859615957589,-4.88406109126486));
#85629=CARTESIAN_POINT('Ctrl Pts',(-9.95027863367802,4.96369311689119,-1.33090685847881));
#85630=CARTESIAN_POINT('Ctrl Pts',(-9.7133340669621,3.82760201545932,3.42914351345493));
#85631=CARTESIAN_POINT('Ctrl Pts',(-9.47638950024621,-0.779444296114679,
5.07956976661125));
#85632=CARTESIAN_POINT('Ctrl Pts',(-9.23944493353029,-4.67967306770249,
2.12372842050058));
#85633=CARTESIAN_POINT('Ctrl Pts',(-9.00250036681439,-4.33626952054219,
-2.75795740899559));
#85634=CARTESIAN_POINT('Ctrl Pts',(-8.76555580009848,-0.0606396802324226,
-5.1386657075344));
#85635=CARTESIAN_POINT('Ctrl Pts',(-8.52861123338258,4.26997957987774,-2.85951688438303));
#85636=CARTESIAN_POINT('Ctrl Pts',(-8.29166666666666,4.72848574930011,2.01270587599516));
#85637=CARTESIAN_POINT('Ctrl Pts',(-8.05472209995076,0.899095167366884,
5.05976188220148));
#85638=CARTESIAN_POINT('Ctrl Pts',(-7.81777753323486,-3.74561504368981,
3.51851252225869));
#85639=CARTESIAN_POINT('Ctrl Pts',(-7.58083296651895,-4.99371766630138,
-1.2134027747215));
#85640=CARTESIAN_POINT('Ctrl Pts',(-7.34388839980304,-1.71340529657878,
-4.84497726661025));
#85641=CARTESIAN_POINT('Ctrl Pts',(-7.10694383308713,3.1206613605197,-4.08301789108291));
#85642=CARTESIAN_POINT('Ctrl Pts',(-6.86999926637123,5.12484242191816,0.38151352985876));
#85643=CARTESIAN_POINT('Ctrl Pts',(-6.63305469965531,2.48170162715197,4.50007993895741));
#85644=CARTESIAN_POINT('Ctrl Pts',(-6.39611013293941,-2.41190177123586,
4.53787310087038));
#85645=CARTESIAN_POINT('Ctrl Pts',(-6.1591655662235,-5.11833863711515,0.460621326634736));
#85646=CARTESIAN_POINT('Ctrl Pts',(-5.9222209995076,-3.18335142828599,-4.03433217575231));
#85647=CARTESIAN_POINT('Ctrl Pts',(-5.68527643279169,1.63837014148066,-4.87086293837728));
#85648=CARTESIAN_POINT('Ctrl Pts',(-5.44833186607578,4.97438096656006,-1.29038611022042));
#85649=CARTESIAN_POINT('Ctrl Pts',(-5.21138729935987,3.79951178264107,3.46024170369659));
#85650=CARTESIAN_POINT('Ctrl Pts',(-4.97444273264398,-0.820839819153767,
5.07304492428149));
#85651=CARTESIAN_POINT('Ctrl Pts',(-4.73749816592805,-4.69683537890069,
2.08549730218345));
#85652=CARTESIAN_POINT('Ctrl Pts',(-4.50055359921216,-4.31363567254264,
-2.79322574532843));
#85653=CARTESIAN_POINT('Ctrl Pts',(-4.26360903249624,-0.0187341292054296,
-5.13898957484612));
#85654=CARTESIAN_POINT('Ctrl Pts',(-4.02666446578034,4.29315512751217,-2.82460176646869));
#85655=CARTESIAN_POINT('Ctrl Pts',(-3.78971989906443,4.71191675257361,2.05119658157601));
#85656=CARTESIAN_POINT('Ctrl Pts',(-3.55277533234853,0.857803758068979,
5.06692699010502));
#85657=CARTESIAN_POINT('Ctrl Pts',(-3.31583076563262,-3.77417911773109,
3.48784869650773));
#85658=CARTESIAN_POINT('Ctrl Pts',(-3.07888619891671,-4.98366295355854,
-1.25407764175316));
#85659=CARTESIAN_POINT('Ctrl Pts',(-2.8419416322008,-1.67382833144973,-4.85879990294167));
#85660=CARTESIAN_POINT('Ctrl Pts',(-2.6049970654849,3.15383037515544,-4.05741211200355));
#85661=CARTESIAN_POINT('Ctrl Pts',(-2.36805249876899,5.12160369599876,0.42324809393336));
#85662=CARTESIAN_POINT('Ctrl Pts',(-2.13110793205308,2.44484109265533,4.52025062240341));
#85663=CARTESIAN_POINT('Ctrl Pts',(-1.89416336533717,-2.44866805478732,
4.51789443713354));
#85664=CARTESIAN_POINT('Ctrl Pts',(-1.65721879862127,-5.12222747943796,
0.419175655533249));
#85665=CARTESIAN_POINT('Ctrl Pts',(-1.42027423190536,-3.14976556924097,
-4.06074695323808));
#85666=CARTESIAN_POINT('Ctrl Pts',(-1.18332966518945,1.67691535926105,-4.85620579037636));
#85667=CARTESIAN_POINT('Ctrl Pts',(-0.946385098473546,4.98690567060087,
-1.25197168347867));
#85668=CARTESIAN_POINT('Ctrl Pts',(-0.70944053175764,3.76685243495724,3.49542825684799));
#85669=CARTESIAN_POINT('Ctrl Pts',(-0.511986726161047,-0.0825881789354425,
4.79667253959683));
#85670=CARTESIAN_POINT('Ctrl Pts',(-0.354023681683779,-2.79930608527943,
3.56272049319328));
#85671=CARTESIAN_POINT('Ctrl Pts',(-0.27504215944514,-3.70786644762908,
2.39576856933903));
#85672=CARTESIAN_POINT('Ctrl Pts',(-0.235551398325822,-3.99485847352278,
1.73494501958064));
#85673=CARTESIAN_POINT('Ctrl Pts',(-24.2394486016742,-2.04298847651427,
4.16621468233147));
#85674=CARTESIAN_POINT('Ctrl Pts',(-24.1999578405549,-2.73215751558814,
3.82826656574272));
#85675=CARTESIAN_POINT('Ctrl Pts',(-24.1209763183162,-3.92939779087658,
2.80390466938141));
#85676=CARTESIAN_POINT('Ctrl Pts',(-23.963013273839,-5.10898000711258,-0.14810717971244));
#85677=CARTESIAN_POINT('Ctrl Pts',(-23.7655594682423,-3.53471751806012,
-4.18089780327223));
#85678=CARTESIAN_POINT('Ctrl Pts',(-23.5286149015265,1.57778831937005,-5.24577579594559));
#85679=CARTESIAN_POINT('Ctrl Pts',(-23.2916703348105,5.25078199648223,-1.5457456218005));
#85680=CARTESIAN_POINT('Ctrl Pts',(-23.0547257680946,4.16672624528416,3.55197009826865));
#85681=CARTESIAN_POINT('Ctrl Pts',(-22.8177812013787,-0.698133122150042,
5.43076832990618));
#85682=CARTESIAN_POINT('Ctrl Pts',(-22.5808366346628,-4.92870131668329,
2.38373809593864));
#85683=CARTESIAN_POINT('Ctrl Pts',(-22.3438920679469,-4.69044178135086,
-2.824353917744));
#85684=CARTESIAN_POINT('Ctrl Pts',(-22.106947501231,-0.198457196997771,
-5.47155282553962));
#85685=CARTESIAN_POINT('Ctrl Pts',(-21.8700029345151,4.47332237297185,-3.15687193446637));
#85686=CARTESIAN_POINT('Ctrl Pts',(-21.6330583677992,5.08868178276068,2.0204513676395));
#85687=CARTESIAN_POINT('Ctrl Pts',(-21.3961138010833,1.08946442363714,5.36562564254283));
#85688=CARTESIAN_POINT('Ctrl Pts',(-21.1591692343674,-3.89767962379977,
3.84510883484102));
#85689=CARTESIAN_POINT('Ctrl Pts',(-20.9222246676515,-5.3503330338353,-1.16222750922764));
#85690=CARTESIAN_POINT('Ctrl Pts',(-20.6852801009356,-1.95117813529016,
-5.11563578110029));
#85691=CARTESIAN_POINT('Ctrl Pts',(-20.4483355342197,3.2173453924395,-4.4300679356503));
#85692=CARTESIAN_POINT('Ctrl Pts',(-20.2113909675038,5.46830984563556,0.272783118978384));
#85693=CARTESIAN_POINT('Ctrl Pts',(-19.9744464007879,2.76048757253021,4.72826915967129));
#85694=CARTESIAN_POINT('Ctrl Pts',(-19.7375018340719,-2.45060616195172,
4.89605442725277));
#85695=CARTESIAN_POINT('Ctrl Pts',(-19.500557267356,-5.4394356071998,0.623988138207389));
#85696=CARTESIAN_POINT('Ctrl Pts',(-19.2636127006401,-3.49566292162464,
-4.21392468261504));
#85697=CARTESIAN_POINT('Ctrl Pts',(-19.0266681339242,1.61805510396288,-5.2305561880293));
#85698=CARTESIAN_POINT('Ctrl Pts',(-18.7897235672083,5.26448456710188,-1.5040022581324));
#85699=CARTESIAN_POINT('Ctrl Pts',(-18.5527790004924,4.13696153123076,3.58641461147908));
#85700=CARTESIAN_POINT('Ctrl Pts',(-18.3158344337765,-0.742050840923869,
5.42459040066293));
#85701=CARTESIAN_POINT('Ctrl Pts',(-18.0788898670606,-4.94815490048041,
2.34362615883809));
#85702=CARTESIAN_POINT('Ctrl Pts',(-17.8419453003447,-4.66716130126134,
-2.86259076147005));
#85703=CARTESIAN_POINT('Ctrl Pts',(-17.6050007336288,-0.153881334594059,
-5.47294628278181));
#85704=CARTESIAN_POINT('Ctrl Pts',(-17.3680561669129,4.49894167248667,-3.12031157263254));
#85705=CARTESIAN_POINT('Ctrl Pts',(-17.1311116001969,5.07202363633252,2.06189153773331));
#85706=CARTESIAN_POINT('Ctrl Pts',(-16.8941670334811,1.04568100099998,5.37432523440605));
#85707=CARTESIAN_POINT('Ctrl Pts',(-16.6572224667651,-3.92890857962264,
3.81320047393507));
#85708=CARTESIAN_POINT('Ctrl Pts',(-16.4202779000492,-5.34067588934766,
-1.20581985641032));
#85709=CARTESIAN_POINT('Ctrl Pts',(-16.1833333333333,-1.90939872139693,
-5.13137574183997));
#85710=CARTESIAN_POINT('Ctrl Pts',(-15.9463887666174,3.25336395982232,-4.40368520970743));
#85711=CARTESIAN_POINT('Ctrl Pts',(-15.7094441999015,5.46590335731091,0.31736567199943));
#85712=CARTESIAN_POINT('Ctrl Pts',(-15.4724996331856,2.72183920522639,4.75062225630792));
#85713=CARTESIAN_POINT('Ctrl Pts',(-15.2355550664697,-2.49044968192745,
4.87590820904461));
#85714=CARTESIAN_POINT('Ctrl Pts',(-14.9986104997538,-5.44434303470384,
0.579611423030416));
#85715=CARTESIAN_POINT('Ctrl Pts',(-14.7616659330379,-3.46118422119377,
-4.24228997926785));
#85716=CARTESIAN_POINT('Ctrl Pts',(-14.524721366322,1.66065394228382,-5.21718784070642));
#85717=CARTESIAN_POINT('Ctrl Pts',(-14.2877767996061,5.27657392776547,-1.46102295192877));
#85718=CARTESIAN_POINT('Ctrl Pts',(-14.0508322328902,4.10757852959245,3.62003026292162));
#85719=CARTESIAN_POINT('Ctrl Pts',(-13.8138876661743,-0.786261050597038,
5.41835898049874));
#85720=CARTESIAN_POINT('Ctrl Pts',(-13.5769430994584,-4.9671015052036,2.3031984539421));
#85721=CARTESIAN_POINT('Ctrl Pts',(-13.3399985327424,-4.64366309822542,
-2.90055400077583));
#85722=CARTESIAN_POINT('Ctrl Pts',(-13.1030539660265,-0.109247019108718,
-5.47401914228049));
#85723=CARTESIAN_POINT('Ctrl Pts',(-12.8661093993106,4.5242367030483,-3.08352115868009));
#85724=CARTESIAN_POINT('Ctrl Pts',(-12.6291648325947,5.05504128224888,2.10318285367604));
#85725=CARTESIAN_POINT('Ctrl Pts',(-12.3922202658788,1.00182124101064,5.38267356267285));
#85726=CARTESIAN_POINT('Ctrl Pts',(-12.1552756991629,-3.95987273301183,
3.78103536344037));
#85727=CARTESIAN_POINT('Ctrl Pts',(-11.918331132447,-5.33066544858701,-1.2493303632258));
#85728=CARTESIAN_POINT('Ctrl Pts',(-11.6813865657311,-1.86749137828179,
-5.14677534319116));
#85729=CARTESIAN_POINT('Ctrl Pts',(-11.4444419990152,3.28916568820829,-4.37700920226935));
#85730=CARTESIAN_POINT('Ctrl Pts',(-11.2074974322993,5.4631336620503,0.361926887382075));
#85731=CARTESIAN_POINT('Ctrl Pts',(-10.9705528655834,2.68300970799308,4.77265957177466));
#85732=CARTESIAN_POINT('Ctrl Pts',(-10.7336082988675,-2.53012752362241,
4.85543769349845));
#85733=CARTESIAN_POINT('Ctrl Pts',(-10.4966637321516,-5.44888846559951,
0.535196198317838));
#85734=CARTESIAN_POINT('Ctrl Pts',(-10.2597191654356,-3.42647534277826,
-4.27037319289192));
#85735=CARTESIAN_POINT('Ctrl Pts',(-10.0227745987198,1.70314234190846,-5.20347255632578));
#85736=CARTESIAN_POINT('Ctrl Pts',(-9.78583003200384,5.28831241647663,-1.41794649651421));
#85737=CARTESIAN_POINT('Ctrl Pts',(-9.54888546528793,4.07792238299417,3.65340519509024));
#85738=CARTESIAN_POINT('Ctrl Pts',(-9.31194089857203,-0.830418974748515,
5.41176725364395));
#85739=CARTESIAN_POINT('Ctrl Pts',(-9.07499633185612,-4.98571781256332,
2.26261759356947));
#85740=CARTESIAN_POINT('Ctrl Pts',(-8.83805176514021,-4.61985610444725,
-2.93832436184929));
#85741=CARTESIAN_POINT('Ctrl Pts',(-8.60110719842431,-0.0646054392067775,
-5.47472799492826));
#85742=CARTESIAN_POINT('Ctrl Pts',(-8.36416263170839,4.54923088486819,-3.0465256994531));
#85743=CARTESIAN_POINT('Ctrl Pts',(-8.12721806499249,5.03772278226943,2.14433431400508));
#85744=CARTESIAN_POINT('Ctrl Pts',(-7.89027349827659,0.957894862798949,
5.39066395845597));
#85745=CARTESIAN_POINT('Ctrl Pts',(-7.65332893156067,-3.99057356617815,
3.74861882489686));
#85746=CARTESIAN_POINT('Ctrl Pts',(-7.41638436484478,-5.32030053373246,
-1.29275779316626));
#85747=CARTESIAN_POINT('Ctrl Pts',(-7.17943979812886,-1.82545985236685,
-5.16183269859543));
#85748=CARTESIAN_POINT('Ctrl Pts',(-6.94249523141296,3.32474869654938,-4.35004213629419));
#85749=CARTESIAN_POINT('Ctrl Pts',(-6.70555066469704,5.46000068378324,0.406464035848652));
#85750=CARTESIAN_POINT('Ctrl Pts',(-6.46860609798114,2.64400179862004,4.79437951861751));
#85751=CARTESIAN_POINT('Ctrl Pts',(-6.23166153126523,-2.56963711973737,
4.83464430588292));
#85752=CARTESIAN_POINT('Ctrl Pts',(-5.99471696454932,-5.45307155961744,
0.490745383240414));
#85753=CARTESIAN_POINT('Ctrl Pts',(-5.75777239783342,-3.39153861606119,
-4.29817243628959));
#85754=CARTESIAN_POINT('Ctrl Pts',(-5.52082783111751,1.74551749230684,-5.18941126080523));
#85755=CARTESIAN_POINT('Ctrl Pts',(-5.28388326440161,5.29969923809883,-1.37477574217999));
#85756=CARTESIAN_POINT('Ctrl Pts',(-5.04693869768569,4.04799508420751,3.68653716794031));
#85757=CARTESIAN_POINT('Ctrl Pts',(-4.80999413096979,-0.874521713036094,
5.4048156948156));
#85758=CARTESIAN_POINT('Ctrl Pts',(-4.57304956425388,-5.00400251737233,
2.22188620810079));
#85759=CARTESIAN_POINT('Ctrl Pts',(-4.33610499753798,-4.59574203119776,
-2.97589920311067));
#85760=CARTESIAN_POINT('Ctrl Pts',(-4.09916043082206,-0.0199593177410495,
-5.47507304275567));
#85761=CARTESIAN_POINT('Ctrl Pts',(-3.86221586410616,4.57392208422876,-3.00932717665144));
#85762=CARTESIAN_POINT('Ctrl Pts',(-3.62527129739025,5.02007019395386,2.18534226341869));
#85763=CARTESIAN_POINT('Ctrl Pts',(-3.38832673067435,0.913903047160537,
5.398297655423));
#85764=CARTESIAN_POINT('Ctrl Pts',(-3.15138216395844,-4.02100569480907,
3.71594962342999));
#85765=CARTESIAN_POINT('Ctrl Pts',(-2.91443759724253,-5.30958825539658,
-1.33609274544807));
#85766=CARTESIAN_POINT('Ctrl Pts',(-2.67749303052662,-1.78329460339402,
-5.17655931799322));
#85767=CARTESIAN_POINT('Ctrl Pts',(-2.44054846381072,3.36008692310967,-4.32276177140254));
#85768=CARTESIAN_POINT('Ctrl Pts',(-2.20360389709481,5.45655014925385,0.450927988029921));
#85769=CARTESIAN_POINT('Ctrl Pts',(-1.96665933037891,2.6047306314334,4.81586933944332));
#85770=CARTESIAN_POINT('Ctrl Pts',(-1.72971476366299,-2.6088078720853,4.81335906261424));
#85771=CARTESIAN_POINT('Ctrl Pts',(-1.49277019694709,-5.45721472734701,
0.44658921727009));
#85772=CARTESIAN_POINT('Ctrl Pts',(-1.25582563023118,-3.35575628399046,
-4.326314707068));
#85773=CARTESIAN_POINT('Ctrl Pts',(-1.01888106351528,1.78658351894942,-5.17379555372219));
#85774=CARTESIAN_POINT('Ctrl Pts',(-0.781936496799368,5.31304304206331,
-1.33384906014582));
#85775=CARTESIAN_POINT('Ctrl Pts',(-0.544991930083462,4.01319985617806,
3.72402487750285));
#85776=CARTESIAN_POINT('Ctrl Pts',(-0.347538124486869,-0.0879893421759137,
5.11036890306578));
#85777=CARTESIAN_POINT('Ctrl Pts',(-0.189575080009601,-2.98237718966264,
3.79571794164222));
#85778=CARTESIAN_POINT('Ctrl Pts',(-0.110593557770963,-3.95035625931582,
2.55244882668638));
#85779=CARTESIAN_POINT('Ctrl Pts',(-0.0711027966516446,-4.25611720348031,
1.8484082462171));
#85780=CARTESIAN_POINT('Ctrl Pts',(-24.075,-2.16839587231048,4.42195480991686));
#85781=CARTESIAN_POINT('Ctrl Pts',(-24.0355092388807,-2.89986906309504,
4.06326198835163));
#85782=CARTESIAN_POINT('Ctrl Pts',(-23.956527716642,-4.17060108187215,2.97602036493736));
#85783=CARTESIAN_POINT('Ctrl Pts',(-23.7985646721648,-5.42259111419047,
-0.157198633687794));
#85784=CARTESIAN_POINT('Ctrl Pts',(-23.6011108665682,-3.75169364098549,
-4.43753924380208));
#85785=CARTESIAN_POINT('Ctrl Pts',(-23.3641662998523,1.67463973411099,-5.56778401530808));
#85786=CARTESIAN_POINT('Ctrl Pts',(-23.1272217331364,5.57309751790704,-1.6406301183221));
#85787=CARTESIAN_POINT('Ctrl Pts',(-22.8902771664205,4.42249777479786,3.77000525856966));
#85788=CARTESIAN_POINT('Ctrl Pts',(-22.6533325997046,-0.740987527730072,
5.76413218450227));
#85789=CARTESIAN_POINT('Ctrl Pts',(-22.4163880329886,-5.23124614446287,
2.53006216497207));
#85790=CARTESIAN_POINT('Ctrl Pts',(-22.1794434662727,-4.97836121687146,
-2.99772487587854));
#85791=CARTESIAN_POINT('Ctrl Pts',(-21.9424988995568,-0.210639351003371,
-5.80742020741697));
#85792=CARTESIAN_POINT('Ctrl Pts',(-21.7055543328409,4.74791408790337,-3.350654274756));
#85793=CARTESIAN_POINT('Ctrl Pts',(-21.468609766125,5.40104689776153,2.14447533902325));
#85794=CARTESIAN_POINT('Ctrl Pts',(-21.2316651994091,1.15634042306232,5.69499075956829));
#85795=CARTESIAN_POINT('Ctrl Pts',(-20.9947206326932,-4.13693591764961,
4.0811381081697));
#85796=CARTESIAN_POINT('Ctrl Pts',(-20.7577760659773,-5.67875942494283,
-1.23357001895319));
#85797=CARTESIAN_POINT('Ctrl Pts',(-20.5208314992614,-2.07094981853471,
-5.42965544813453));
#85798=CARTESIAN_POINT('Ctrl Pts',(-20.2838869325455,3.41483985297175,-4.70200450768531));
#85799=CARTESIAN_POINT('Ctrl Pts',(-20.0469423658296,5.8039781594961,0.289527716885543));
#85800=CARTESIAN_POINT('Ctrl Pts',(-19.8099977991137,2.92993814044999,5.01851060192832));
#85801=CARTESIAN_POINT('Ctrl Pts',(-19.5730532323978,-2.60103487969802,
5.19659524892496));
#85802=CARTESIAN_POINT('Ctrl Pts',(-19.3361086656819,-5.77333149645322,
0.662291206638737));
#85803=CARTESIAN_POINT('Ctrl Pts',(-19.099164098966,-3.71024170590167,-4.47259345466305));
#85804=CARTESIAN_POINT('Ctrl Pts',(-18.86221953225,1.71737826666076,-5.55163016257556));
#85805=CARTESIAN_POINT('Ctrl Pts',(-18.6252749655341,5.58764121108655,-1.59632436793984));
#85806=CARTESIAN_POINT('Ctrl Pts',(-18.3883303988182,4.39090597492436,3.80656412374579));
#85807=CARTESIAN_POINT('Ctrl Pts',(-18.1513858321023,-0.787601104461023,
5.75757502746272));
#85808=CARTESIAN_POINT('Ctrl Pts',(-17.9144412653864,-5.25189387267684,
2.48748798511786));
#85809=CARTESIAN_POINT('Ctrl Pts',(-17.6774966986705,-4.95365168105575,
-3.03830886108399));
#85810=CARTESIAN_POINT('Ctrl Pts',(-17.4405521319546,-0.163327230963516,
-5.80889920104172));
#85811=CARTESIAN_POINT('Ctrl Pts',(-17.2036075652387,4.77510600991274,-3.31184968109235));
#85812=CARTESIAN_POINT('Ctrl Pts',(-16.9666629985228,5.38336620285286,2.18845928450913));
#85813=CARTESIAN_POINT('Ctrl Pts',(-16.7297184318069,1.10986938614095,5.70422436969573));
#85814=CARTESIAN_POINT('Ctrl Pts',(-16.492773865091,-4.17008184073304,4.04727107520497));
#85815=CARTESIAN_POINT('Ctrl Pts',(-16.2558292983751,-5.6685094835036,-1.27983825138911));
#85816=CARTESIAN_POINT('Ctrl Pts',(-16.0188847316592,-2.02660580500988,
-5.44636159517873));
#85817=CARTESIAN_POINT('Ctrl Pts',(-15.7819401649432,3.45306939451705,-4.67400229685913));
#85818=CARTESIAN_POINT('Ctrl Pts',(-15.5449955982273,5.80142395059578,0.336846938241531));
#85819=CARTESIAN_POINT('Ctrl Pts',(-15.3080510315114,2.88891737058441,5.04223582751692));
#85820=CARTESIAN_POINT('Ctrl Pts',(-15.0711064647955,-2.64332416583296,
5.17521236942885));
#85821=CARTESIAN_POINT('Ctrl Pts',(-14.8341618980796,-5.77854016290716,
0.615190458336615));
#85822=CARTESIAN_POINT('Ctrl Pts',(-14.5972173313637,-3.67364655494689,
-4.50269993489332));
#85823=CARTESIAN_POINT('Ctrl Pts',(-14.3602727646478,1.76259200439949,-5.53744120875238));
#85824=CARTESIAN_POINT('Ctrl Pts',(-14.1233281979319,5.60047266856326,-1.55070680756783));
#85825=CARTESIAN_POINT('Ctrl Pts',(-13.886383631216,4.3597193186113,3.84224324806341));
#85826=CARTESIAN_POINT('Ctrl Pts',(-13.6494390645001,-0.834525126437326,
5.75096109600007));
#85827=CARTESIAN_POINT('Ctrl Pts',(-13.4124944977842,-5.2720035012667,2.44457865428648));
#85828=CARTESIAN_POINT('Ctrl Pts',(-13.1755499310683,-4.92871105752529,
-3.07860244685626));
#85829=CARTESIAN_POINT('Ctrl Pts',(-12.9386053643524,-0.115953069741155,
-5.8100379172583));
#85830=CARTESIAN_POINT('Ctrl Pts',(-12.7016607976365,4.80195375794968,-3.27280091372428));
#85831=CARTESIAN_POINT('Ctrl Pts',(-12.4647162309206,5.36534139903216,2.23228523853764));
#85832=CARTESIAN_POINT('Ctrl Pts',(-12.2277716642046,1.06331732595328,5.7130851541605));
#85833=CARTESIAN_POINT('Ctrl Pts',(-11.9908270974887,-4.20294670667358,
4.01313153226046));
#85834=CARTESIAN_POINT('Ctrl Pts',(-11.7538825307728,-5.6578845589507,-1.32601961974504));
#85835=CARTESIAN_POINT('Ctrl Pts',(-11.5169379640569,-1.98212600941875,
-5.46270649011525));
#85836=CARTESIAN_POINT('Ctrl Pts',(-11.279993397341,3.49106878655774,-4.64568880166157));
#85837=CARTESIAN_POINT('Ctrl Pts',(-11.0430488306251,5.79848423955988,0.384143512163343));
#85838=CARTESIAN_POINT('Ctrl Pts',(-10.8061042639092,2.84770435225732,5.06562588793293));
#85839=CARTESIAN_POINT('Ctrl Pts',(-10.5691596971933,-2.6854376036436,5.15348528583311));
#85840=CARTESIAN_POINT('Ctrl Pts',(-10.3322151304774,-5.78336461184819,
0.5680488366184));
#85841=CARTESIAN_POINT('Ctrl Pts',(-10.0952705637615,-3.63680709669546,
-4.53250701662856));
#85842=CARTESIAN_POINT('Ctrl Pts',(-9.85832599704558,1.80768852424102,-5.5228840213867));
#85843=CARTESIAN_POINT('Ctrl Pts',(-9.62138143032965,5.61293171606208,-1.5049861345496));
#85844=CARTESIAN_POINT('Ctrl Pts',(-9.38443686361376,4.328242750529,3.87766687672554));
#85845=CARTESIAN_POINT('Ctrl Pts',(-9.14749229689785,-0.881393653382343,
5.74396474067666));
#85846=CARTESIAN_POINT('Ctrl Pts',(-8.91054773018194,-5.29176255742414,
2.40150676663836));
#85847=CARTESIAN_POINT('Ctrl Pts',(-8.67360316346604,-4.90344268835231,
-3.11869131470298));
#85848=CARTESIAN_POINT('Ctrl Pts',(-8.43665859675012,-0.0685711981811391,
-5.81079028232212));
#85849=CARTESIAN_POINT('Ctrl Pts',(-8.19971403003422,4.82848218985865,-3.23353451452318));
#85850=CARTESIAN_POINT('Ctrl Pts',(-7.96276946331831,5.34695981523874,2.27596275201499));
#85851=CARTESIAN_POINT('Ctrl Pts',(-7.7258248966024,1.01669455823101,5.72156603471045));
#85852=CARTESIAN_POINT('Ctrl Pts',(-7.4888803298865,-4.23553208866649,3.97872512753503));
#85853=CARTESIAN_POINT('Ctrl Pts',(-7.2519357631706,-5.64688340116356,-1.37211281161101));
#85854=CARTESIAN_POINT('Ctrl Pts',(-7.01499119645468,-1.93751440815492,
-5.4786881305806));
#85855=CARTESIAN_POINT('Ctrl Pts',(-6.77804662973878,3.52883603257905,-4.61706638150548));
#85856=CARTESIAN_POINT('Ctrl Pts',(-6.54110206302287,5.79515894564832,0.431414541838547));
#85857=CARTESIAN_POINT('Ctrl Pts',(-6.30415749630696,2.8063019700881,5.08867909827761));
#85858=CARTESIAN_POINT('Ctrl Pts',(-6.06721292959106,-2.72737246823887,
5.13141551089547));
#85859=CARTESIAN_POINT('Ctrl Pts',(-5.83026836287515,-5.78780448211972,
0.520869439846087));
#85860=CARTESIAN_POINT('Ctrl Pts',(-5.59332379615924,-3.59972580383638,
-4.56201269682687));
#85861=CARTESIAN_POINT('Ctrl Pts',(-5.35637922944334,1.85266484313302,-5.50795958323318));
#85862=CARTESIAN_POINT('Ctrl Pts',(-5.11943466272742,5.62501750963759,-1.45916537413956));
#85863=CARTESIAN_POINT('Ctrl Pts',(-4.88249009601152,4.29647838577394,3.91283263218402));
#85864=CARTESIAN_POINT('Ctrl Pts',(-4.64554552929562,-0.928203606918421,
5.73658646534971));
#85865=CARTESIAN_POINT('Ctrl Pts',(-4.4086009625797,-5.31116965584398,2.35827511401814));
#85866=CARTESIAN_POINT('Ctrl Pts',(-4.1716563958638,-4.87784838985289,-3.15857266089292));
#85867=CARTESIAN_POINT('Ctrl Pts',(-3.93471182914789,-0.0211845062766748,
-5.8111565106652));
#85868=CARTESIAN_POINT('Ctrl Pts',(-3.69776726243199,4.85468904094535,-3.19405258683419));
#85869=CARTESIAN_POINT('Ctrl Pts',(-3.46082269571607,5.3282236353341,2.31948794526136));
#85870=CARTESIAN_POINT('Ctrl Pts',(-3.22387812900017,0.970002336252103,
5.72966832074098));
#85871=CARTESIAN_POINT('Ctrl Pts',(-2.98693356228426,-4.26783227188706,
3.94405055035223));
#85872=CARTESIAN_POINT('Ctrl Pts',(-2.74998899556836,-5.63551355723462,
-1.41810784914298));
#85873=CARTESIAN_POINT('Ctrl Pts',(-2.51304442885244,-1.89276087533832,
-5.49431873304477));
#85874=CARTESIAN_POINT('Ctrl Pts',(-2.27609986213654,3.56634347106391,-4.58811143080153));
#85875=CARTESIAN_POINT('Ctrl Pts',(-2.03915529542063,5.79149660250893,0.478607882126479));
#85876=CARTESIAN_POINT('Ctrl Pts',(-1.80221072870473,2.76462017021148,5.11148805648324));
#85877=CARTESIAN_POINT('Ctrl Pts',(-1.56526616198882,-2.76894768938328,
5.10882368809493));
#85878=CARTESIAN_POINT('Ctrl Pts',(-1.32832159527291,-5.79220197525607,
0.474002779006931));
#85879=CARTESIAN_POINT('Ctrl Pts',(-1.091377028557,-3.56174699873994,-4.59188246089791));
#85880=CARTESIAN_POINT('Ctrl Pts',(-0.854432461841098,1.89625167863778,
-5.49138531706803));
#85881=CARTESIAN_POINT('Ctrl Pts',(-0.61748789512519,5.63918041352576,-1.41572643681296));
#85882=CARTESIAN_POINT('Ctrl Pts',(-0.380543328409284,4.25954727739888,
3.9526214981577));
#85883=CARTESIAN_POINT('Ctrl Pts',(-0.183089522812691,-0.0933905054163845,
5.42406526653476));
#85884=CARTESIAN_POINT('Ctrl Pts',(-0.0251264783354233,-3.16544829404585,
4.02871539009116));
#85885=CARTESIAN_POINT('Ctrl Pts',(0.0538550439032153,-4.19284607100255,
2.70912908403373));
#85886=CARTESIAN_POINT('Ctrl Pts',(0.0933458050225333,-4.51737593343784,
1.96187147285355));
#85887=CARTESIAN_POINT('Ctrl Pts',(-1.30884152590359,-4.93160574955951,
0.00236265628207036));
#85888=CARTESIAN_POINT('Ctrl Pts',(-1.23635336012139,-4.92283193517292,
-1.48758864232717));
#85889=CARTESIAN_POINT('Ctrl Pts',(-1.1638651943392,-4.199882729552,-2.98499340090942));
#85890=CARTESIAN_POINT('Ctrl Pts',(-1.091377028557,-3.02382304859632,-3.89748539694214));
#85891=CARTESIAN_POINT('Ctrl Pts',(-1.01239550631837,-1.74241410628069,
-4.89171674628795));
#85892=CARTESIAN_POINT('Ctrl Pts',(-0.933413984079733,0.0769187861785456,
-5.19155103167799));
#85893=CARTESIAN_POINT('Ctrl Pts',(-0.854432461841099,1.6104066882228,-4.66219169433051));
#85894=CARTESIAN_POINT('Ctrl Pts',(-0.775450939602464,3.14389459026709,
-4.13283235698302));
#85895=CARTESIAN_POINT('Ctrl Pts',(-0.696469417363827,4.39153750189643,
-2.77427939689798));
#85896=CARTESIAN_POINT('Ctrl Pts',(-0.617487895125191,4.78542010168994,
-1.20027826102703));
#85897=CARTESIAN_POINT('Ctrl Pts',(-0.54499193008346,5.14695908417373,0.244473980857804));
#85898=CARTESIAN_POINT('Ctrl Pts',(-0.472495965041731,4.78919380489134,
1.87074413694423));
#85899=CARTESIAN_POINT('Ctrl Pts',(-0.4,3.87692992261799,3.04758435726506));
#85900=CARTESIAN_POINT('',(-24.075,-2.36230756092325,-3.31488661006751));
#85901=CARTESIAN_POINT('Ctrl Pts',(-24.075,-2.36815640427391,-3.31717604989033));
#85902=CARTESIAN_POINT('Ctrl Pts',(-24.075,-2.46522217779123,-3.26269169255296));
#85903=CARTESIAN_POINT('Ctrl Pts',(-24.075,-2.55968914443286,-3.20413331253052));
#85904=CARTESIAN_POINT('Ctrl Pts',(-24.075,-2.65125836302674,-3.14156318060015));
#85905=CARTESIAN_POINT('Ctrl Pts',(-24.075,-2.75265715944677,-3.07227640315455));
#85906=CARTESIAN_POINT('Ctrl Pts',(-24.075,-2.85050398777766,-2.99807148801027));
#85907=CARTESIAN_POINT('Ctrl Pts',(-24.075,-2.94470883192884,-2.91935158607538));
#85908=CARTESIAN_POINT('Ctrl Pts',(-24.075,-3.00710083212058,-2.86721528479628));
#85909=CARTESIAN_POINT('Ctrl Pts',(-24.075,-3.06789492736163,-2.81309743864922));
#85910=CARTESIAN_POINT('Ctrl Pts',(-24.075,-3.12705945033238,-2.75710407731575));
#85911=CARTESIAN_POINT('Ctrl Pts',(-24.075,-3.14913589562531,-2.73621090829861));
#85912=CARTESIAN_POINT('Ctrl Pts',(-24.075,-3.17098540543271,-2.71505652816831));
#85913=CARTESIAN_POINT('Ctrl Pts',(-24.075,-3.1926061526888,-2.69364616544278));
#85914=CARTESIAN_POINT('Ctrl Pts',(-24.075,-3.21187742140056,-2.6745624192423));
#85915=CARTESIAN_POINT('Ctrl Pts',(-24.075,-3.23096928898991,-2.65527273168143));
#85916=CARTESIAN_POINT('Ctrl Pts',(-24.075,-3.24986239903768,-2.63579970423287));
#85917=CARTESIAN_POINT('Ctrl Pts',(-24.075,-3.33763886311812,-2.54532897230711));
#85918=CARTESIAN_POINT('Ctrl Pts',(-24.075,-3.42120552992453,-2.45082907208921));
#85919=CARTESIAN_POINT('Ctrl Pts',(-24.075,-3.50047047807597,-2.35272286112832));
#85920=CARTESIAN_POINT('Ctrl Pts',(-24.075,-3.58222055611672,-2.25154080538519));
#85921=CARTESIAN_POINT('Ctrl Pts',(-24.075,-3.65939552565808,-2.14652235759255));
#85922=CARTESIAN_POINT('Ctrl Pts',(-24.075,-3.73186566997445,-2.03808369899882));
#85923=CARTESIAN_POINT('Ctrl Pts',(-24.075,-3.76357135811286,-1.99064178586406));
#85924=CARTESIAN_POINT('Ctrl Pts',(-24.075,-3.79437609562932,-1.94254465774222));
#85925=CARTESIAN_POINT('Ctrl Pts',(-24.075,-3.82426691847838,-1.89382475550747));
#85926=CARTESIAN_POINT('Ctrl Pts',(-24.075,-3.83956001467533,-1.86889810309161));
#85927=CARTESIAN_POINT('Ctrl Pts',(-24.075,-3.85461385608546,-1.84380840731357));
#85928=CARTESIAN_POINT('Ctrl Pts',(-24.075,-3.86942656298479,-1.81855988523347));
#85929=CARTESIAN_POINT('Ctrl Pts',(-24.075,-3.88195432078001,-1.79720609949691));
#85930=CARTESIAN_POINT('Ctrl Pts',(-24.075,-3.8943111380858,-1.77573580108553));
#85931=CARTESIAN_POINT('Ctrl Pts',(-24.075,-3.90648349164623,-1.75417386639733));
#85932=CARTESIAN_POINT('Ctrl Pts',(-24.075,-3.97142359119054,-1.63913989387354));
#85933=CARTESIAN_POINT('Ctrl Pts',(-24.075,-4.0311892465264,-1.52137916274476));
#85934=CARTESIAN_POINT('Ctrl Pts',(-24.075,-4.08568055028152,-1.4013346551155));
#85935=CARTESIAN_POINT('Ctrl Pts',(-24.075,-4.14095875510494,-1.27955660204347));
#85936=CARTESIAN_POINT('Ctrl Pts',(-24.075,-4.19080969883921,-1.15542771938113));
#85937=CARTESIAN_POINT('Ctrl Pts',(-24.075,-4.23509479303713,-1.02936906546279));
#85938=CARTESIAN_POINT('Ctrl Pts',(-24.075,-4.27955865607226,-0.902801541474532));
#85939=CARTESIAN_POINT('Ctrl Pts',(-24.075,-4.31841214000889,-0.774287905363049));
#85940=CARTESIAN_POINT('Ctrl Pts',(-24.075,-4.35147302458191,-0.644223199816743));
#85941=CARTESIAN_POINT('Ctrl Pts',(-24.075,-4.37626868801167,-0.546674670657014));
#85942=CARTESIAN_POINT('Ctrl Pts',(-24.075,-4.39780520039582,-0.448252951430205));
#85943=CARTESIAN_POINT('Ctrl Pts',(-24.075,-4.41598771602322,-0.349117080270156));
#85944=CARTESIAN_POINT('Ctrl Pts',(-24.075,-4.42409435259613,-0.304917559406111));
#85945=CARTESIAN_POINT('Ctrl Pts',(-24.075,-4.43153406314493,-0.260576012738608));
#85946=CARTESIAN_POINT('Ctrl Pts',(-24.075,-4.43829734901448,-0.216106282184517));
#85947=CARTESIAN_POINT('Ctrl Pts',(-24.075,-4.44105429138625,-0.197978927110287));
#85948=CARTESIAN_POINT('Ctrl Pts',(-24.075,-4.44369882081601,-0.179829889752053));
#85949=CARTESIAN_POINT('Ctrl Pts',(-24.075,-4.44622832119494,-0.161675304990112));
#85950=CARTESIAN_POINT('Ctrl Pts',(-24.075,-4.46525383825745,-0.0251264572304002));
#85951=CARTESIAN_POINT('Ctrl Pts',(-24.075,-4.47780790977246,0.111941212499941));
#85952=CARTESIAN_POINT('Ctrl Pts',(-24.075,-4.48375110993555,0.249092150554736));
#85953=CARTESIAN_POINT('Ctrl Pts',(-24.075,-4.48812249139626,0.349970305669875));
#85954=CARTESIAN_POINT('Ctrl Pts',(-24.075,-4.48891660930822,0.45089430308268));
#85955=CARTESIAN_POINT('Ctrl Pts',(-24.075,-4.48606214368721,0.551699386922404));
#85956=CARTESIAN_POINT('Ctrl Pts',(-24.075,-4.48230147276619,0.684506993605575));
#85957=CARTESIAN_POINT('Ctrl Pts',(-24.075,-4.47221017375029,0.817108224592498));
#85958=CARTESIAN_POINT('Ctrl Pts',(-24.075,-4.45604820619817,0.949137326263566));
#85959=CARTESIAN_POINT('Ctrl Pts',(-24.075,-4.43963517353196,1.08321740974537));
#85960=CARTESIAN_POINT('Ctrl Pts',(-24.075,-4.41696130249557,1.21670818235846));
#85961=CARTESIAN_POINT('Ctrl Pts',(-24.075,-4.38824518180506,1.34922954103877));
#85962=CARTESIAN_POINT('Ctrl Pts',(-24.075,-4.37931508605012,1.39044083261068));
#85963=CARTESIAN_POINT('Ctrl Pts',(-24.075,-4.36980027908974,1.43155835145695));
#85964=CARTESIAN_POINT('Ctrl Pts',(-24.075,-4.35970632441813,1.47257054689663));
#85965=CARTESIAN_POINT('Ctrl Pts',(-24.075,-4.35444366245617,1.49395298103058));
#85966=CARTESIAN_POINT('Ctrl Pts',(-24.075,-4.3490235663563,1.5153067841905));
#85967=CARTESIAN_POINT('Ctrl Pts',(-24.075,-4.34344677462285,1.53663030771368));
#85968=CARTESIAN_POINT('Ctrl Pts',(-24.075,-4.33851478916861,1.55548833807884));
#85969=CARTESIAN_POINT('Ctrl Pts',(-24.075,-4.33346207484754,1.57431558186746));
#85970=CARTESIAN_POINT('Ctrl Pts',(-24.075,-4.32829137421139,1.59310410207121));
#85971=CARTESIAN_POINT('Ctrl Pts',(-24.075,-4.29192404049517,1.72525029121772));
#85972=CARTESIAN_POINT('Ctrl Pts',(-24.075,-4.24969695453619,1.85558580736706));
#85973=CARTESIAN_POINT('Ctrl Pts',(-24.075,-4.2019146732641,1.98372972318377));
#85974=CARTESIAN_POINT('Ctrl Pts',(-24.075,-4.15300946825373,2.11488512863962));
#85975=CARTESIAN_POINT('Ctrl Pts',(-24.075,-4.09828482443508,2.24374547578093));
#85976=CARTESIAN_POINT('Ctrl Pts',(-24.075,-4.03801214778829,2.36990589624912));
#85977=CARTESIAN_POINT('Ctrl Pts',(-24.075,-3.97819023957664,2.49512278577635));
#85978=CARTESIAN_POINT('Ctrl Pts',(-24.075,-3.9129026279478,2.61768076524124));
#85979=CARTESIAN_POINT('Ctrl Pts',(-24.075,-3.84236456925686,2.73717578743023));
#85980=CARTESIAN_POINT('Ctrl Pts',(-24.075,-3.79151963980002,2.82330965737785));
#85981=CARTESIAN_POINT('Ctrl Pts',(-24.075,-3.73794565441772,2.90785194850061));
#85982=CARTESIAN_POINT('Ctrl Pts',(-24.075,-3.68172933073621,2.99070582618902));
#85983=CARTESIAN_POINT('Ctrl Pts',(-24.075,-3.65713468912554,3.0269543976777));
#85984=CARTESIAN_POINT('Ctrl Pts',(-24.075,-3.63203413392643,3.06287971452895));
#85985=CARTESIAN_POINT('Ctrl Pts',(-24.075,-3.60643423361074,3.0984732479178));
#85986=CARTESIAN_POINT('Ctrl Pts',(-24.075,-3.59002992000832,3.12128144157202));
#85987=CARTESIAN_POINT('Ctrl Pts',(-24.075,-3.57342055722774,3.14395339301573));
#85988=CARTESIAN_POINT('Ctrl Pts',(-24.075,-3.55660778713698,3.16648679521622));
#85989=CARTESIAN_POINT('Ctrl Pts',(-24.075,-3.54464951465408,3.18251393185257));
#85990=CARTESIAN_POINT('Ctrl Pts',(-24.075,-3.53259319266495,3.19846442704866));
#85991=CARTESIAN_POINT('Ctrl Pts',(-24.075,-3.52044352982494,3.2143326587511));
#85992=CARTESIAN_POINT('Ctrl Pts',(-24.075,-3.43385204863387,3.32742663552169));
#85993=CARTESIAN_POINT('Ctrl Pts',(-24.075,-3.34246367499149,3.43642334193498));
#85994=CARTESIAN_POINT('Ctrl Pts',(-24.075,-3.24660658320202,3.54108838415155));
#85995=CARTESIAN_POINT('Ctrl Pts',(-24.075,-3.14949239534693,3.64712603229974));
#85996=CARTESIAN_POINT('Ctrl Pts',(-24.075,-3.04779120566173,3.74871830265496));
#85997=CARTESIAN_POINT('Ctrl Pts',(-24.075,-2.94179464465091,3.84560251040417));
#85998=CARTESIAN_POINT('Ctrl Pts',(-24.075,-2.83591529575862,3.94237958257149));
#85999=CARTESIAN_POINT('Ctrl Pts',(-24.075,-2.72574964233738,4.03445961903589));
#86000=CARTESIAN_POINT('Ctrl Pts',(-24.075,-2.61154486618463,4.12155256477766));
#86001=CARTESIAN_POINT('Ctrl Pts',(-24.075,-2.49884949462962,4.20749443350531));
#86002=CARTESIAN_POINT('Ctrl Pts',(-24.075,-2.38222058031806,4.28858070101923));
#86003=CARTESIAN_POINT('Ctrl Pts',(-24.075,-2.26186014424435,4.36449667397723));
#86004=CARTESIAN_POINT('Ctrl Pts',(-24.075,-2.23095061393297,4.38399250785596));
#86005=CARTESIAN_POINT('Ctrl Pts',(-24.075,-2.19979482468899,4.40314714871446));
#86006=CARTESIAN_POINT('Ctrl Pts',(-24.075,-2.16839587231048,4.42195480991686));
#86007=CARTESIAN_POINT('Ctrl Pts',(-24.075,-2.36815640427393,-3.31717604989031));
#86008=CARTESIAN_POINT('Ctrl Pts',(-24.0025040349583,-1.3617188644407,-4.02543705998425));
#86009=CARTESIAN_POINT('Ctrl Pts',(-23.8510265476779,1.47227864893343,-4.51291701816237));
#86010=CARTESIAN_POINT('Ctrl Pts',(-23.6205675381589,4.60615095363263,-1.3559766287573));
#86011=CARTESIAN_POINT('Ctrl Pts',(-23.383622971443,3.65518318625674,3.11589977766662));
#86012=CARTESIAN_POINT('Ctrl Pts',(-23.1466784047271,-0.612424310989975,
4.764040620714));
#86013=CARTESIAN_POINT('Ctrl Pts',(-22.9528665245548,-3.64803811708131,
2.57766597303378));
#86014=CARTESIAN_POINT('Ctrl Pts',(-22.8380361666211,-4.06550901707725,
0.614403937029799));
#86015=CARTESIAN_POINT('Ctrl Pts',(-22.8021873309261,-4.06417652423825,
0.000957366820343933));
#86016=CARTESIAN_POINT('Origin',(-24.075,-4.52129938221115E-16,0.));
#86017=CARTESIAN_POINT('',(-24.075,-4.925,-6.03138548580072E-16));
#86018=CARTESIAN_POINT('Origin',(-24.075,0.,0.));
#86019=CARTESIAN_POINT('Origin',(-24.075,0.,0.));
#86020=CARTESIAN_POINT('',(-24.075,2.36230756092324,-3.31488661006752));
#86021=CARTESIAN_POINT('Ctrl Pts',(-24.075,2.17492961456583,4.42583829068187));
#86022=CARTESIAN_POINT('Ctrl Pts',(-24.075,2.28965550950647,4.35795907372157));
#86023=CARTESIAN_POINT('Ctrl Pts',(-24.075,2.40120874042602,4.2852779095045));
#86024=CARTESIAN_POINT('Ctrl Pts',(-24.075,2.50923374297498,4.20778498795177));
#86025=CARTESIAN_POINT('Ctrl Pts',(-24.075,2.62615380967427,4.12391109447456));
#86026=CARTESIAN_POINT('Ctrl Pts',(-24.075,2.73894143904689,4.03440012317382));
#86027=CARTESIAN_POINT('Ctrl Pts',(-24.075,2.84740951963401,3.93967163892028));
#86028=CARTESIAN_POINT('Ctrl Pts',(-24.075,2.91362172535409,3.88184649945993));
#86029=CARTESIAN_POINT('Ctrl Pts',(-24.075,2.97822357748513,3.82207648115163));
#86030=CARTESIAN_POINT('Ctrl Pts',(-24.075,3.04116458918038,3.76045190069527));
#86031=CARTESIAN_POINT('Ctrl Pts',(-24.075,3.07749457133285,3.72488177165171));
#86032=CARTESIAN_POINT('Ctrl Pts',(-24.075,3.1132711002268,3.68869369961702));
#86033=CARTESIAN_POINT('Ctrl Pts',(-24.075,3.14848348994726,3.65190463013972));
#86034=CARTESIAN_POINT('Ctrl Pts',(-24.075,3.16457534766412,3.63509223892561));
#86035=CARTESIAN_POINT('Ctrl Pts',(-24.075,3.18054960258019,3.61815398695129));
#86036=CARTESIAN_POINT('Ctrl Pts',(-24.075,3.19639494117543,3.60110280017532));
#86037=CARTESIAN_POINT('Ctrl Pts',(-24.075,3.29344145236556,3.49667093976963));
#86038=CARTESIAN_POINT('Ctrl Pts',(-24.075,3.38575286062018,3.38790483579936));
#86039=CARTESIAN_POINT('Ctrl Pts',(-24.075,3.47315306439507,3.27521866189171));
#86040=CARTESIAN_POINT('Ctrl Pts',(-24.075,3.55797717983118,3.16585387084138));
#86041=CARTESIAN_POINT('Ctrl Pts',(-24.075,3.63817539662055,3.05279585502674));
#86042=CARTESIAN_POINT('Ctrl Pts',(-24.075,3.7135454129426,2.93640277138696));
#86043=CARTESIAN_POINT('Ctrl Pts',(-24.075,3.74871167292264,2.88209590455991));
#86044=CARTESIAN_POINT('Ctrl Pts',(-24.075,3.78282623953752,2.82706277914621));
#86045=CARTESIAN_POINT('Ctrl Pts',(-24.075,3.81586528773782,2.7713389298113));
#86046=CARTESIAN_POINT('Ctrl Pts',(-24.075,3.83534796990618,2.73847932564811));
#86047=CARTESIAN_POINT('Ctrl Pts',(-24.075,3.85445662143509,2.70537952834091));
#86048=CARTESIAN_POINT('Ctrl Pts',(-24.075,3.87318600005773,2.67204678176061));
#86049=CARTESIAN_POINT('Ctrl Pts',(-24.075,3.88234637995079,2.65574401872149));
#86050=CARTESIAN_POINT('Ctrl Pts',(-24.075,3.89141648248476,2.63938470305005));
#86051=CARTESIAN_POINT('Ctrl Pts',(-24.075,3.90039427182564,2.62297224029516));
#86052=CARTESIAN_POINT('Ctrl Pts',(-24.075,3.96798015327673,2.49941724028842));
#86053=CARTESIAN_POINT('Ctrl Pts',(-24.075,4.03013714290421,2.37322115583376));
#86054=CARTESIAN_POINT('Ctrl Pts',(-24.075,4.08669911225055,2.2447758702003));
#86055=CARTESIAN_POINT('Ctrl Pts',(-24.075,4.14305273718887,2.11680370912927));
#86056=CARTESIAN_POINT('Ctrl Pts',(-24.075,4.19385272226738,1.98659807729368));
#86057=CARTESIAN_POINT('Ctrl Pts',(-24.075,4.23888567590795,1.85453121402251));
#86058=CARTESIAN_POINT('Ctrl Pts',(-24.075,4.28463415928028,1.7203659370429));
#86059=CARTESIAN_POINT('Ctrl Pts',(-24.075,4.32443131919811,1.58427900590199));
#86060=CARTESIAN_POINT('Ctrl Pts',(-24.075,4.35799738760436,1.4466570002418));
#86061=CARTESIAN_POINT('Ctrl Pts',(-24.075,4.38317193890905,1.34344049599666));
#86062=CARTESIAN_POINT('Ctrl Pts',(-24.075,4.40484037060623,1.23936036076217));
#86063=CARTESIAN_POINT('Ctrl Pts',(-24.075,4.42286232376388,1.13458253413241));
#86064=CARTESIAN_POINT('Ctrl Pts',(-24.075,4.42983214075538,1.09406071776829));
#86065=CARTESIAN_POINT('Ctrl Pts',(-24.075,4.43625635126417,1.05343459359125));
#86066=CARTESIAN_POINT('Ctrl Pts',(-24.075,4.44212603033172,1.01271396551675));
#86067=CARTESIAN_POINT('Ctrl Pts',(-24.075,4.44613530083295,0.984899836149257));
#86068=CARTESIAN_POINT('Ctrl Pts',(-24.075,4.44988584300443,0.957041618230944));
#86069=CARTESIAN_POINT('Ctrl Pts',(-24.075,4.45337468872272,0.929142476094225));
#86070=CARTESIAN_POINT('Ctrl Pts',(-24.075,4.45563697462939,0.911051725983625));
#86071=CARTESIAN_POINT('Ctrl Pts',(-24.075,4.4577880479084,0.892953104338779));
#86072=CARTESIAN_POINT('Ctrl Pts',(-24.075,4.45982721955001,0.874849527478534));
#86073=CARTESIAN_POINT('Ctrl Pts',(-24.075,4.47478304533433,0.742073092150142));
#86074=CARTESIAN_POINT('Ctrl Pts',(-24.075,4.48372824823947,0.60899351884243));
#86075=CARTESIAN_POINT('Ctrl Pts',(-24.075,4.48646532204813,0.475939379020343));
#86076=CARTESIAN_POINT('Ctrl Pts',(-24.075,4.48847299247554,0.378342865210339));
#86077=CARTESIAN_POINT('Ctrl Pts',(-24.075,4.48713945358514,0.280759890275653));
#86078=CARTESIAN_POINT('Ctrl Pts',(-24.075,4.48236892158366,0.183321653579532));
#86079=CARTESIAN_POINT('Ctrl Pts',(-24.075,4.47578175720543,0.0487786546766431));
#86080=CARTESIAN_POINT('Ctrl Pts',(-24.075,4.46264317126887,-0.0854895344690163));
#86081=CARTESIAN_POINT('Ctrl Pts',(-24.075,4.44314296552314,-0.21904427821751));
#86082=CARTESIAN_POINT('Ctrl Pts',(-24.075,4.42369313349789,-0.352254017948207));
#86083=CARTESIAN_POINT('Ctrl Pts',(-24.075,4.39791402784372,-0.484754784643175));
#86084=CARTESIAN_POINT('Ctrl Pts',(-24.075,4.36594964169936,-0.61608509773256));
#86085=CARTESIAN_POINT('Ctrl Pts',(-24.075,4.35385913591727,-0.665760693021671));
#86086=CARTESIAN_POINT('Ctrl Pts',(-24.075,4.34088326963657,-0.715268498642894));
#86087=CARTESIAN_POINT('Ctrl Pts',(-24.075,4.32702839056672,-0.764582200478806));
#86088=CARTESIAN_POINT('Ctrl Pts',(-24.075,4.32173468134526,-0.78342411146457));
#86089=CARTESIAN_POINT('Ctrl Pts',(-24.075,4.3163121694248,-0.802239047480007));
#86090=CARTESIAN_POINT('Ctrl Pts',(-24.075,4.31076658107729,-0.821007896647057));
#86091=CARTESIAN_POINT('Ctrl Pts',(-24.075,4.27335222769683,-0.947635462790869));
#86092=CARTESIAN_POINT('Ctrl Pts',(-24.075,4.23028981465208,-1.07234901794428));
#86093=CARTESIAN_POINT('Ctrl Pts',(-24.075,4.18179488094431,-1.19475063707284));
#86094=CARTESIAN_POINT('Ctrl Pts',(-24.075,4.13349333262168,-1.3166641498685));
#86095=CARTESIAN_POINT('Ctrl Pts',(-24.075,4.07980199860719,-1.43628486967417));
#86096=CARTESIAN_POINT('Ctrl Pts',(-24.075,4.0208894094103,-1.55319433159216));
#86097=CARTESIAN_POINT('Ctrl Pts',(-24.075,3.96451542589954,-1.66506604132794));
#86098=CARTESIAN_POINT('Ctrl Pts',(-24.075,3.90335983940973,-1.77445551914991));
#86099=CARTESIAN_POINT('Ctrl Pts',(-24.075,3.83753818876811,-1.88096500634148));
#86100=CARTESIAN_POINT('Ctrl Pts',(-24.075,3.79191922374558,-1.95478346156703));
#86101=CARTESIAN_POINT('Ctrl Pts',(-24.075,3.74405823914087,-2.02721781351839));
#86102=CARTESIAN_POINT('Ctrl Pts',(-24.075,3.69401073517597,-2.09816998853326));
#86103=CARTESIAN_POINT('Ctrl Pts',(-24.075,3.66886589076295,-2.13381774836491));
#86104=CARTESIAN_POINT('Ctrl Pts',(-24.075,3.64316903300121,-2.16909123324359));
#86105=CARTESIAN_POINT('Ctrl Pts',(-24.075,3.61692676036711,-2.2039771396978));
#86106=CARTESIAN_POINT('Ctrl Pts',(-24.075,3.60244455312235,-2.22322947101209));
#86107=CARTESIAN_POINT('Ctrl Pts',(-24.075,3.58779623189004,-2.24236375257261));
#86108=CARTESIAN_POINT('Ctrl Pts',(-24.075,3.57298287249688,-2.26137766816133));
#86109=CARTESIAN_POINT('Ctrl Pts',(-24.075,3.56231194413342,-2.27507450260456));
#86110=CARTESIAN_POINT('Ctrl Pts',(-24.075,3.55155763390175,-2.28870591199351));
#86111=CARTESIAN_POINT('Ctrl Pts',(-24.075,3.5407265295119,-2.30226366689239));
#86112=CARTESIAN_POINT('Ctrl Pts',(-24.075,3.45910540154826,-2.40443231079706));
#86113=CARTESIAN_POINT('Ctrl Pts',(-24.075,3.37302709147514,-2.50254959411214));
#86114=CARTESIAN_POINT('Ctrl Pts',(-24.075,3.28274367897956,-2.59634605947702));
#86115=CARTESIAN_POINT('Ctrl Pts',(-24.075,3.19479267636066,-2.68771935766017));
#86116=CARTESIAN_POINT('Ctrl Pts',(-24.075,3.10285030444394,-2.77499251082065));
#86117=CARTESIAN_POINT('Ctrl Pts',(-24.075,3.00711854707771,-2.85787507032547));
#86118=CARTESIAN_POINT('Ctrl Pts',(-24.075,2.90757866320222,-2.94405462636194));
#86119=CARTESIAN_POINT('Ctrl Pts',(-24.075,2.80394144723911,-3.02548821247834));
#86120=CARTESIAN_POINT('Ctrl Pts',(-24.075,2.69640867303135,-3.10179438524463));
#86121=CARTESIAN_POINT('Ctrl Pts',(-24.075,2.59626634490311,-3.17285623450566));
#86122=CARTESIAN_POINT('Ctrl Pts',(-24.075,2.49274485090672,-3.23947105721393));
#86123=CARTESIAN_POINT('Ctrl Pts',(-24.075,2.38599459059339,-3.30128078051072));
#86124=CARTESIAN_POINT('Ctrl Pts',(-24.075,2.37811648292838,-3.30584230245407));
#86125=CARTESIAN_POINT('Ctrl Pts',(-24.075,2.37022078672256,-3.3103776307273));
#86126=CARTESIAN_POINT('Ctrl Pts',(-24.075,2.3623075609233,-3.31488661006747));
#86127=CARTESIAN_POINT('Origin',(-24.075,0.,0.));
#86128=CARTESIAN_POINT('Origin',(-26.8478126690739,0.,0.));
#86129=CARTESIAN_POINT('Ctrl Pts',(-24.075,2.36230756092323,-3.31488661006752));
#86130=CARTESIAN_POINT('Ctrl Pts',(-24.0355092388807,2.91065117590484,-2.92411720524959));
#86131=CARTESIAN_POINT('Ctrl Pts',(-23.956527716642,3.8009161537758,-1.86677512529004));
#86132=CARTESIAN_POINT('Ctrl Pts',(-23.7985646721648,4.40104888295471,0.856562345338821));
#86133=CARTESIAN_POINT('Ctrl Pts',(-23.6011108665681,2.46349467463415,4.12278630825743));
#86134=CARTESIAN_POINT('Ctrl Pts',(-23.3641662998523,-2.11355533076443,
4.31564323485309));
#86135=CARTESIAN_POINT('Ctrl Pts',(-23.1964002340208,-3.99108416375442,
1.67729393881811));
#86136=CARTESIAN_POINT('Ctrl Pts',(-23.107615690428,-4.07555252481818,0.169077405975379));
#86137=CARTESIAN_POINT('Ctrl Pts',(-23.0978126690739,-4.07427440555673,
0.002413955370523));
#86138=CARTESIAN_POINT('Ctrl Pts',(-24.5683458050225,2.8582151425001,-4.01076441581691));
#86139=CARTESIAN_POINT('Ctrl Pts',(-24.5288550439032,3.52166982958631,-3.53796271609248));
#86140=CARTESIAN_POINT('Ctrl Pts',(-24.4498735216646,4.59882374581641,-2.25865802531723));
#86141=CARTESIAN_POINT('Ctrl Pts',(-24.2919104771873,5.32493938055571,1.03637625618311));
#86142=CARTESIAN_POINT('Ctrl Pts',(-24.0944566715907,2.9806439682038,4.9882625152113));
#86143=CARTESIAN_POINT('Ctrl Pts',(-23.8575121048748,-2.55724358285579,
5.22160494574418));
#86144=CARTESIAN_POINT('Ctrl Pts',(-23.6205675381589,-5.76563780154427,
0.713091159141606));
#86145=CARTESIAN_POINT('Ctrl Pts',(-23.383622971443,-3.75101053411091,-4.43862093040455));
#86146=CARTESIAN_POINT('Ctrl Pts',(-23.1466784047271,1.66791135734842,-5.56707796774283));
#86147=CARTESIAN_POINT('Ctrl Pts',(-22.9097338380112,5.57288068372362,-1.64625563203397));
#86148=CARTESIAN_POINT('Ctrl Pts',(-22.6727892712953,4.42499321806552,3.76694508752895));
#86149=CARTESIAN_POINT('Ctrl Pts',(-22.4358447045794,-0.735970718489106,
5.76444706334991));
#86150=CARTESIAN_POINT('Ctrl Pts',(-22.1989001378635,-5.22933511388625,
2.53448853123921));
#86151=CARTESIAN_POINT('Ctrl Pts',(-21.9619555711475,-4.98072793392136,
-2.99373285471432));
#86152=CARTESIAN_POINT('Ctrl Pts',(-21.7250110044317,-0.215429665592803,
-5.80720569596091));
#86153=CARTESIAN_POINT('Ctrl Pts',(-21.4880664377157,4.74519617498286,-3.35455594069076));
#86154=CARTESIAN_POINT('Ctrl Pts',(-21.2511218709998,5.40278690230385,2.14007065312858));
#86155=CARTESIAN_POINT('Ctrl Pts',(-21.0141773042839,1.16100167435296,5.69403825692435));
#86156=CARTESIAN_POINT('Ctrl Pts',(-20.777232737568,-4.13360179746769,4.08452187604581));
#86157=CARTESIAN_POINT('Ctrl Pts',(-20.5402881708521,-5.67976472349785,
-1.22892904398937));
#86158=CARTESIAN_POINT('Ctrl Pts',(-20.3033436041362,-2.07538872218816,
-5.42796029465347));
#86159=CARTESIAN_POINT('Ctrl Pts',(-20.0663990374203,3.41099566797876,-4.70479524800842));
#86160=CARTESIAN_POINT('Ctrl Pts',(-19.8294544707044,5.80421311058715,0.284783282234712));
#86161=CARTESIAN_POINT('Ctrl Pts',(-19.5925099039885,2.9340399889667,5.0161140549384));
#86162=CARTESIAN_POINT('Ctrl Pts',(-19.3555653372726,-2.59678620885327,
5.19872023686729));
#86163=CARTESIAN_POINT('Ctrl Pts',(-19.1186207705567,-5.77278857082837,
0.667010532133052));
#86164=CARTESIAN_POINT('Ctrl Pts',(-18.8816762038408,-3.71389697834065,
-4.46955927193808));
#86165=CARTESIAN_POINT('Ctrl Pts',(-18.6447316371249,1.71283953929854,-5.55303264456375));
#86166=CARTESIAN_POINT('Ctrl Pts',(-18.407787070409,5.58633481703289,-1.60089168284028));
#86167=CARTESIAN_POINT('Ctrl Pts',(-18.170842503693,4.39401659788682,3.80297370387212));
#86168=CARTESIAN_POINT('Ctrl Pts',(-17.9338979369771,-0.782894255534373,
5.75821738380674));
#86169=CARTESIAN_POINT('Ctrl Pts',(-17.6969533702612,-5.24985906935669,
2.4917806103693));
#86170=CARTESIAN_POINT('Ctrl Pts',(-17.4600088035453,-4.95613413085725,
-3.0342586134341));
#86171=CARTESIAN_POINT('Ctrl Pts',(-17.2230642368294,-0.168075791623614,
-5.80876418738683));
#86172=CARTESIAN_POINT('Ctrl Pts',(-16.9861196701135,4.77239743889964,-3.31575233424595));
#86173=CARTESIAN_POINT('Ctrl Pts',(-16.7491751033976,5.38515381465317,2.18405797750162));
#86174=CARTESIAN_POINT('Ctrl Pts',(-16.5122305366817,1.11453213417911,5.70331561273725));
#86175=CARTESIAN_POINT('Ctrl Pts',(-16.2752859699658,-4.16677224069193,
4.05067894936963));
#86176=CARTESIAN_POINT('Ctrl Pts',(-16.0383414032499,-5.66955425092678,
-1.2752040826549));
#86177=CARTESIAN_POINT('Ctrl Pts',(-15.801396836534,-2.03105752138112,-5.44470349986785));
#86178=CARTESIAN_POINT('Ctrl Pts',(-15.564452269818,3.44924764526761,-4.67682387291358));
#86179=CARTESIAN_POINT('Ctrl Pts',(-15.3275077031022,5.8016978162655,0.332104359158765));
#86180=CARTESIAN_POINT('Ctrl Pts',(-15.0905631363862,2.89303850364856,5.03987292231073));
#86181=CARTESIAN_POINT('Ctrl Pts',(-14.8536185696703,-2.63909290111009,
5.17737187344555));
#86182=CARTESIAN_POINT('Ctrl Pts',(-14.6166740029544,-5.77803577211796,
0.619914084981969));
#86183=CARTESIAN_POINT('Ctrl Pts',(-14.3797294362385,-3.67732643095217,
-4.49969567602683));
#86184=CARTESIAN_POINT('Ctrl Pts',(-14.1427848695226,1.75806485555589,-5.53888064687201));
#86185=CARTESIAN_POINT('Ctrl Pts',(-13.9058403028067,5.59920356681868,-1.55528462795688));
#86186=CARTESIAN_POINT('Ctrl Pts',(-13.6688957360908,4.36285911384371,3.83867831543423));
#86187=CARTESIAN_POINT('Ctrl Pts',(-13.4319511693749,-0.829823670846763,
5.75164181186002));
#86188=CARTESIAN_POINT('Ctrl Pts',(-13.195006602659,-5.2700037705162,2.44888773025208));
#86189=CARTESIAN_POINT('Ctrl Pts',(-12.9580620359431,-4.93122645223466,
-3.07457257735367));
#86190=CARTESIAN_POINT('Ctrl Pts',(-12.7211174692272,-0.120702573666628,
-5.80994163011507));
#86191=CARTESIAN_POINT('Ctrl Pts',(-12.4841729025113,4.79927710131223,-3.27672552427787));
#86192=CARTESIAN_POINT('Ctrl Pts',(-12.2472283357954,5.3671648418537,2.22789865501186));
#86193=CARTESIAN_POINT('Ctrl Pts',(-12.0102837690794,1.06798732945511,5.71221444982219));
#86194=CARTESIAN_POINT('Ctrl Pts',(-11.7733392023636,-4.19966500623136,
4.01656628129922));
#86195=CARTESIAN_POINT('Ctrl Pts',(-11.5363946356476,-5.6589670810085,-1.32139412466384));
#86196=CARTESIAN_POINT('Ctrl Pts',(-11.2994500689317,-1.98659109873622,
-5.4610847514991));
#86197=CARTESIAN_POINT('Ctrl Pts',(-11.0625055022158,3.48727017294997,-4.64854144839944));
#86198=CARTESIAN_POINT('Ctrl Pts',(-10.8255609354999,5.79879676953481,0.379403324006022));
#86199=CARTESIAN_POINT('Ctrl Pts',(-10.588616368784,2.85184461663589,5.06329666711314));
#86200=CARTESIAN_POINT('Ctrl Pts',(-10.3516718020681,-2.68122408930307,
5.15567922194299));
#86201=CARTESIAN_POINT('Ctrl Pts',(-10.1147272353522,-5.78289875669314,
0.572776419269867));
#86202=CARTESIAN_POINT('Ctrl Pts',(-9.87778266863627,-3.6405113486111,-4.52953286523761));
#86203=CARTESIAN_POINT('Ctrl Pts',(-9.6408381019204,1.80317326383209,-5.52436032833061));
#86204=CARTESIAN_POINT('Ctrl Pts',(-9.40389353520446,5.61169998639889,-1.50957415163656));
#86205=CARTESIAN_POINT('Ctrl Pts',(-9.16694896848858,4.33141151164837,3.87412766611946));
#86206=CARTESIAN_POINT('Ctrl Pts',(-8.93000440177265,-0.876697905012197,
5.74468377197292));
#86207=CARTESIAN_POINT('Ctrl Pts',(-8.69305983505676,-5.28979803156989,
2.4058320061605));
#86208=CARTESIAN_POINT('Ctrl Pts',(-8.45611526834085,-4.90599086103837,
-3.11468209100355));
#86209=CARTESIAN_POINT('Ctrl Pts',(-8.21917070162494,-0.0733213293745337,
-5.8107327282556));
#86210=CARTESIAN_POINT('Ctrl Pts',(-7.98222613490903,4.82583762550951,-3.23748082142428));
#86211=CARTESIAN_POINT('Ctrl Pts',(-7.74528156819313,5.3488189678476,2.27159118364012));
#86212=CARTESIAN_POINT('Ctrl Pts',(-7.50833700147721,1.02137150668363,5.72073344087819));
#86213=CARTESIAN_POINT('Ctrl Pts',(-7.27139243476131,-4.23227850613741,
3.9821865231059));
#86214=CARTESIAN_POINT('Ctrl Pts',(-7.0344478680454,-5.64800360567914,-1.36749629789557));
#86215=CARTESIAN_POINT('Ctrl Pts',(-6.7975033013295,-1.94199257388176,-5.47710285624032));
#86216=CARTESIAN_POINT('Ctrl Pts',(-6.56055873461358,3.52506080794271,-4.61994990973791));
#86217=CARTESIAN_POINT('Ctrl Pts',(-6.32361416789768,5.79551011773543,0.426677060786518));
#86218=CARTESIAN_POINT('Ctrl Pts',(-6.08666960118177,2.81046109317731,5.08638371486386));
#86219=CARTESIAN_POINT('Ctrl Pts',(-5.84972503446586,-2.72317698967916,
5.13364373679603));
#86220=CARTESIAN_POINT('Ctrl Pts',(-5.61278046774996,-5.78737718356205,
0.525600657238108));
#86221=CARTESIAN_POINT('Ctrl Pts',(-5.37583590103405,-3.60345420458392,
-4.55906883743519));
#86222=CARTESIAN_POINT('Ctrl Pts',(-5.13889133431814,1.84816180838766,-5.50947268628944));
#86223=CARTESIAN_POINT('Ctrl Pts',(-4.90194676760224,5.62382316291067,-1.46376323391524));
#86224=CARTESIAN_POINT('Ctrl Pts',(-4.66500220088632,4.29967603859304,3.90931928494839));
#86225=CARTESIAN_POINT('Ctrl Pts',(-4.42805763417043,-0.923514140359199,
5.73734394489365));
#86226=CARTESIAN_POINT('Ctrl Pts',(-4.19111306745451,-5.30923996143927,
2.36261588240264));
#86227=CARTESIAN_POINT('Ctrl Pts',(-3.95416850073861,-4.88043013966745,
-3.15458368267413));
#86228=CARTESIAN_POINT('Ctrl Pts',(-3.71722393402269,-0.0259330876983714,
-5.81113897502467));
#86229=CARTESIAN_POINT('Ctrl Pts',(-3.4802793673068,4.85207316848768,-3.19801786516862));
#86230=CARTESIAN_POINT('Ctrl Pts',(-3.24333480059088,5.33012524590221,2.3151269509498));
#86231=CARTESIAN_POINT('Ctrl Pts',(-3.00639023387499,0.9746727144288,5.72888298509305));
#86232=CARTESIAN_POINT('Ctrl Pts',(-2.76944566715907,-4.26458165159571,
3.94752089103779));
#86233=CARTESIAN_POINT('Ctrl Pts',(-2.53250110044317,-5.63672012231858,
-1.41346705206928));
#86234=CARTESIAN_POINT('Ctrl Pts',(-2.29555653372726,-1.89715814085517,
-5.49283453792041));
#86235=CARTESIAN_POINT('Ctrl Pts',(-2.05861196701135,3.56241187898916,-4.59090168980564));
#86236=CARTESIAN_POINT('Ctrl Pts',(-1.82166740029544,5.79223230496278,0.473635218544011));
#86237=CARTESIAN_POINT('Ctrl Pts',(-1.58472283357953,2.76813296477938,5.10968449907998));
#86238=CARTESIAN_POINT('Ctrl Pts',(-1.34777826686363,-2.76349068556974,
5.11020522979376));
#86239=CARTESIAN_POINT('Ctrl Pts',(-1.11083370014772,-5.79429292799479,
0.480439815238698));
#86240=CARTESIAN_POINT('Ctrl Pts',(-0.873889133431811,-3.56054538524804,
-4.59233251686338));
#86241=CARTESIAN_POINT('Ctrl Pts',(-0.676435327835228,0.973652097174675,
-5.33676463268154));
#86242=CARTESIAN_POINT('Ctrl Pts',(-0.518472283357948,3.77810762024814,
-3.46072517404051));
#86243=CARTESIAN_POINT('Ctrl Pts',(-0.439490761119318,4.57738664511715,
-1.99170029627505));
#86244=CARTESIAN_POINT('Ctrl Pts',(-0.4,4.77615934004777,-1.20163511869221));
#86245=CARTESIAN_POINT('Ctrl Pts',(-24.4038972033484,2.69291261530781,-3.77880514723378));
#86246=CARTESIAN_POINT('Ctrl Pts',(-24.364406442229,3.31799694502582,-3.33334754581152));
#86247=CARTESIAN_POINT('Ctrl Pts',(-24.2854249199904,4.33285454846954,-2.12803039197483));
#86248=CARTESIAN_POINT('Ctrl Pts',(-24.1274618755131,5.01697588135538,0.976438285901677));
#86249=CARTESIAN_POINT('Ctrl Pts',(-23.9300080699166,2.80826087034725,4.69977044622668));
#86250=CARTESIAN_POINT('Ctrl Pts',(-23.6930635032006,-2.40934749882534,
4.91961770878048));
#86251=CARTESIAN_POINT('Ctrl Pts',(-23.4561189364847,-5.43218687082214,
0.671850117145879));
#86252=CARTESIAN_POINT('Ctrl Pts',(-23.2191743697688,-3.53407391811104,
-4.18191693141772));
#86253=CARTESIAN_POINT('Ctrl Pts',(-22.9822298030529,1.57144907275594,-5.24511058206187));
#86254=CARTESIAN_POINT('Ctrl Pts',(-22.745285236337,5.25057770272587,-1.55104578854338));
#86255=CARTESIAN_POINT('Ctrl Pts',(-22.5083406696211,4.1690773666383,3.54908690970877));
#86256=CARTESIAN_POINT('Ctrl Pts',(-22.2713961029052,-0.693406455954522,
5.43106499799406));
#86257=CARTESIAN_POINT('Ctrl Pts',(-22.0344515361893,-4.92690080899178,
2.38790846694518));
#86258=CARTESIAN_POINT('Ctrl Pts',(-21.7975069694733,-4.69267162126242,
-2.82059277184779));
#86259=CARTESIAN_POINT('Ctrl Pts',(-21.5605624027575,-0.202970467674054,
-5.47135072017758));
#86260=CARTESIAN_POINT('Ctrl Pts',(-21.3236178360415,4.47076164831466,-3.16054795075367));
#86261=CARTESIAN_POINT('Ctrl Pts',(-21.0866732693257,5.09032115556824,2.01630142313886));
#86262=CARTESIAN_POINT('Ctrl Pts',(-20.8497287026097,1.09385609528459,5.36472822710765));
#86263=CARTESIAN_POINT('Ctrl Pts',(-20.6127841358939,-3.89453832972245,
3.84829690527888));
#86264=CARTESIAN_POINT('Ctrl Pts',(-20.3758395691779,-5.35128019177339,
-1.15785494124226));
#86265=CARTESIAN_POINT('Ctrl Pts',(-20.138895002462,-1.95536031859356,-5.1140386654297));
#86266=CARTESIAN_POINT('Ctrl Pts',(-19.9019504357461,3.21372353273086,-4.43269727579702));
#86267=CARTESIAN_POINT('Ctrl Pts',(-19.6650058690302,5.46853120852308,0.268313074812095));
#86268=CARTESIAN_POINT('Ctrl Pts',(-19.4280613023143,2.7643521940041,4.72601121500983));
#86269=CARTESIAN_POINT('Ctrl Pts',(-19.1911167355984,-2.44660320949863,
4.89805651826131));
#86270=CARTESIAN_POINT('Ctrl Pts',(-18.9541721688825,-5.43892408123292,
0.628434525384623));
#86271=CARTESIAN_POINT('Ctrl Pts',(-18.7172276021666,-3.49910679438177,
-4.21106597935799));
#86272=CARTESIAN_POINT('Ctrl Pts',(-18.4802830354507,1.61377887017298,-5.23187755862264));
#86273=CARTESIAN_POINT('Ctrl Pts',(-18.2433384687348,5.26325372727624,-1.50830542612371));
#86274=CARTESIAN_POINT('Ctrl Pts',(-18.0063939020189,4.13989225386688,3.58303184059237));
#86275=CARTESIAN_POINT('Ctrl Pts',(-17.769449335303,-0.737616208742238,
5.42519560685493));
#86276=CARTESIAN_POINT('Ctrl Pts',(-17.532504768587,-4.94623777834044,2.34767052363083));
#86277=CARTESIAN_POINT('Ctrl Pts',(-17.2955602018711,-4.66950018061578,
-2.85877475656918));
#86278=CARTESIAN_POINT('Ctrl Pts',(-17.0586156351552,-0.158355266145258,
-5.47281907753085));
#86279=CARTESIAN_POINT('Ctrl Pts',(-16.8216710684393,4.49638974945534,-3.12398851904368));
#86280=CARTESIAN_POINT('Ctrl Pts',(-16.5847265017234,5.07370786307136,2.05774477670468));
#86281=CARTESIAN_POINT('Ctrl Pts',(-16.3477819350075,1.05007408283181,5.3734690346605));
#86282=CARTESIAN_POINT('Ctrl Pts',(-16.1108373682916,-3.92579038758392,
3.81641125649406));
#86283=CARTESIAN_POINT('Ctrl Pts',(-15.8738928015757,-5.3416602335043,-1.20145370102185));
#86284=CARTESIAN_POINT('Ctrl Pts',(-15.6369482348598,-1.91359297640511,
-5.1298135411107));
#86285=CARTESIAN_POINT('Ctrl Pts',(-15.4000036681439,3.24976323830444,-4.40634360222628));
#86286=CARTESIAN_POINT('Ctrl Pts',(-15.163059101428,5.46616138418435,0.312897376085954));
#86287=CARTESIAN_POINT('Ctrl Pts',(-14.926114534712,2.72572199594175,4.74839600778522));
#86288=CARTESIAN_POINT('Ctrl Pts',(-14.6891699679962,-2.48646312892746,
4.87794281991868));
#86289=CARTESIAN_POINT('Ctrl Pts',(-14.4522254012802,-5.443867814942,0.584061862605154));
#86290=CARTESIAN_POINT('Ctrl Pts',(-14.2152808345644,-3.46465127459014,
-4.2394594692475));
#86291=CARTESIAN_POINT('Ctrl Pts',(-13.9783362678484,1.65638861737841,-5.21854403010367));
#86292=CARTESIAN_POINT('Ctrl Pts',(-13.7413917011325,5.27537822347882,-1.46533601783238));
#86293=CARTESIAN_POINT('Ctrl Pts',(-13.5044471344166,4.11053673734424,3.61667150524551));
#86294=CARTESIAN_POINT('Ctrl Pts',(-13.2675025677007,-0.781831499832336,
5.41900032771556));
#86295=CARTESIAN_POINT('Ctrl Pts',(-13.0305580009848,-4.96521742723999,
2.30725831803544));
#86296=CARTESIAN_POINT('Ctrl Pts',(-12.7936134342689,-4.64603301714601,
-2.89675719546884));
#86297=CARTESIAN_POINT('Ctrl Pts',(-12.556668867553,-0.113721839372316,
-5.47392842382517));
#86298=CARTESIAN_POINT('Ctrl Pts',(-12.3197243008371,4.52171484865091,-3.08721879260303));
#86299=CARTESIAN_POINT('Ctrl Pts',(-12.0827797341212,5.05675926775122,2.09904996460866));
#86300=CARTESIAN_POINT('Ctrl Pts',(-11.8458351674053,1.00622115869235,5.3818532148054));
#86301=CARTESIAN_POINT('Ctrl Pts',(-11.6088906006894,-3.95678082702158,
3.78427146658718));
#86302=CARTESIAN_POINT('Ctrl Pts',(-11.3719460339735,-5.33168536386997,
-1.24497237985674));
#86303=CARTESIAN_POINT('Ctrl Pts',(-11.1350014672575,-1.87169823282282,
-5.14524739649701));
#86304=CARTESIAN_POINT('Ctrl Pts',(-10.8980569005417,3.28558676430121,-4.37969686852414));
#86305=CARTESIAN_POINT('Ctrl Pts',(-10.6611123338257,5.46342811711062,0.357460844116834));
#86306=CARTESIAN_POINT('Ctrl Pts',(-10.4241677671098,2.68691052357899,4.77046505952951));
#86307=CARTESIAN_POINT('Ctrl Pts',(-10.1872232003939,-2.52615769442597,
4.85750474511386));
#86308=CARTESIAN_POINT('Ctrl Pts',(-9.95027863367801,-5.44844955279505,
0.539650365106313));
#86309=CARTESIAN_POINT('Ctrl Pts',(-9.71333406696212,-3.42996536232423,
-4.26757104910595));
#86310=CARTESIAN_POINT('Ctrl Pts',(-9.47638950024621,1.69888821787986,-5.20486348226912));
#86311=CARTESIAN_POINT('Ctrl Pts',(-9.23944493353029,5.2871519228877,-1.42226916939806));
#86312=CARTESIAN_POINT('Ctrl Pts',(-9.00250036681439,4.08090788141461,3.65007067182512));
#86313=CARTESIAN_POINT('Ctrl Pts',(-8.76555580009848,-0.825994801131819,
5.41244470035525));
#86314=CARTESIAN_POINT('Ctrl Pts',(-8.52861123338258,-4.98386690344967,
2.26669268641333));
#86315=CARTESIAN_POINT('Ctrl Pts',(-8.29166666666667,-4.62225690565715,
-2.93454700831237));
#86316=CARTESIAN_POINT('Ctrl Pts',(-8.05472209995076,-0.0690808504607675,
-5.47467376945395));
#86317=CARTESIAN_POINT('Ctrl Pts',(-7.81777753323485,4.54673926672794,-3.05024377493309));
#86318=CARTESIAN_POINT('Ctrl Pts',(-7.58083296651895,5.03947441231285,2.14021557169967));
#86319=CARTESIAN_POINT('Ctrl Pts',(-7.34388839980303,0.962301323775909,
5.38987951700474));
#86320=CARTESIAN_POINT('Ctrl Pts',(-7.10694383308713,-3.98750815192461,
3.75188003349546));
#86321=CARTESIAN_POINT('Ctrl Pts',(-6.86999926637122,-5.32135595213918,
-1.28840827173304));
#86322=CARTESIAN_POINT('Ctrl Pts',(-6.63305469965532,-1.82967902705385,
-5.16033910729566));
#86323=CARTESIAN_POINT('Ctrl Pts',(-6.39611013293941,3.32119180893176,-4.35275889803766));
#86324=CARTESIAN_POINT('Ctrl Pts',(-6.1591655662235,5.46033154612088,0.402000543125495));
#86325=CARTESIAN_POINT('Ctrl Pts',(-5.92222099950759,2.64792038223854,4.79221688681979));
#86326=CARTESIAN_POINT('Ctrl Pts',(-5.68527643279169,-2.56568428323716,
4.83674366416711));
#86327=CARTESIAN_POINT('Ctrl Pts',(-5.44833186607578,-5.45266897352119,
0.495202974557197));
#86328=CARTESIAN_POINT('Ctrl Pts',(-5.21138729935988,-3.39505138781118,
-4.29539883258997));
#86329=CARTESIAN_POINT('Ctrl Pts',(-4.97444273264396,1.7412748868806,-5.19083685478796));
#86330=CARTESIAN_POINT('Ctrl Pts',(-4.73749816592806,5.29857396543472,-1.37910768850874));
#86331=CARTESIAN_POINT('Ctrl Pts',(-4.50055359921215,4.05100780339995,3.68322701225883));
#86332=CARTESIAN_POINT('Ctrl Pts',(-4.26360903249624,-0.870103457926947,
5.40552936615175));
#86333=CARTESIAN_POINT('Ctrl Pts',(-4.02666446578034,-5.00218442525993,
2.22597593170799));
#86334=CARTESIAN_POINT('Ctrl Pts',(-3.78971989906444,-4.5981744676305,-2.97214092417364));
#86335=CARTESIAN_POINT('Ctrl Pts',(-3.55277533234852,-0.0244332688531125,
-5.47505652127451));
#86336=CARTESIAN_POINT('Ctrl Pts',(-3.31583076563262,4.57145749860798,-3.01306312636748));
#86337=CARTESIAN_POINT('Ctrl Pts',(-3.0788861989167,5.0218618264353,2.18123348363432));
#86338=CARTESIAN_POINT('Ctrl Pts',(-2.84194163220081,0.918303317848106,
5.39755773901779));
#86339=CARTESIAN_POINT('Ctrl Pts',(-2.60499706548489,-4.01794307147468,
3.7192192598099));
#86340=CARTESIAN_POINT('Ctrl Pts',(-2.36805249876899,-5.31072503977907,
-1.33172034506469));
#86341=CARTESIAN_POINT('Ctrl Pts',(-2.13110793205308,-1.78743755666829,
-5.17516096007589));
#86342=CARTESIAN_POINT('Ctrl Pts',(-1.89416336533717,3.35638271143614,-4.32539065806695));
#86343=CARTESIAN_POINT('Ctrl Pts',(-1.65721879862126,5.45724330296002,0.446242914364961));
#86344=CARTESIAN_POINT('Ctrl Pts',(-1.42027423190536,2.60804026641022,4.8141700893024));
#86345=CARTESIAN_POINT('Ctrl Pts',(-1.18332966518945,-2.60366646960906,
4.81466070398266));
#86346=CARTESIAN_POINT('Ctrl Pts',(-0.946385098473544,-5.45918475155002,
0.452653972793905));
#86347=CARTESIAN_POINT('Ctrl Pts',(-0.709440531757633,-3.35462416482876,
-4.32673873441604));
#86348=CARTESIAN_POINT('Ctrl Pts',(-0.51198672616105,0.917341727155359,
-5.02811722972881));
#86349=CARTESIAN_POINT('Ctrl Pts',(-0.354023681683771,3.55960386650859,
-3.26057697361968));
#86350=CARTESIAN_POINT('Ctrl Pts',(-0.27504215944514,4.31265724489702,-1.87651194411482));
#86351=CARTESIAN_POINT('Ctrl Pts',(-0.235551398325822,4.49993408413774,
-1.13213953771605));
#86352=CARTESIAN_POINT('Ctrl Pts',(-24.2394486016742,2.52761008811552,-3.54684587865065));
#86353=CARTESIAN_POINT('Ctrl Pts',(-24.1999578405549,3.11432406046533,-3.12873237553055));
#86354=CARTESIAN_POINT('Ctrl Pts',(-24.1209763183162,4.06688535112267,-1.99740275863244));
#86355=CARTESIAN_POINT('Ctrl Pts',(-23.963013273839,4.70901238215504,0.916500315620253));
#86356=CARTESIAN_POINT('Ctrl Pts',(-23.7655594682423,2.6358777724907,4.41127837724205));
#86357=CARTESIAN_POINT('Ctrl Pts',(-23.5286149015265,-2.26145141479489,
4.61763047181679));
#86358=CARTESIAN_POINT('Ctrl Pts',(-23.2916703348105,-5.0987359401,0.630609075150145));
#86359=CARTESIAN_POINT('Ctrl Pts',(-23.0547257680947,-3.31713730211117,
-3.92521293243088));
#86360=CARTESIAN_POINT('Ctrl Pts',(-22.8177812013787,1.47498678816346,-4.9231431963809));
#86361=CARTESIAN_POINT('Ctrl Pts',(-22.5808366346628,4.92827472172813,-1.45583594505279));
#86362=CARTESIAN_POINT('Ctrl Pts',(-22.3438920679469,3.91316151521107,3.33122873188859));
#86363=CARTESIAN_POINT('Ctrl Pts',(-22.106947501231,-0.650842193419926,
5.09768293263822));
#86364=CARTESIAN_POINT('Ctrl Pts',(-21.8700029345151,-4.62446650409733,
2.24132840265115));
#86365=CARTESIAN_POINT('Ctrl Pts',(-21.6330583677992,-4.40461530860346,
-2.64745268898125));
#86366=CARTESIAN_POINT('Ctrl Pts',(-21.3961138010833,-0.190511269755314,
-5.13549574439427));
#86367=CARTESIAN_POINT('Ctrl Pts',(-21.1591692343674,4.19632712164646,-2.96653996081657));
#86368=CARTESIAN_POINT('Ctrl Pts',(-20.9222246676515,4.77785540883261,1.89253219314915));
#86369=CARTESIAN_POINT('Ctrl Pts',(-20.6852801009356,1.02671051621624,5.03541819729095));
#86370=CARTESIAN_POINT('Ctrl Pts',(-20.4483355342197,-3.65547486197721,
3.61207193451195));
#86371=CARTESIAN_POINT('Ctrl Pts',(-20.2113909675038,-5.02279566004892,
-1.08678083849515));
#86372=CARTESIAN_POINT('Ctrl Pts',(-19.9744464007879,-1.83533191499897,
-4.80011703620592));
#86373=CARTESIAN_POINT('Ctrl Pts',(-19.7375018340719,3.01645139748298,-4.16059930358563));
#86374=CARTESIAN_POINT('Ctrl Pts',(-19.500557267356,5.132849306459,0.25184286738948));
#86375=CARTESIAN_POINT('Ctrl Pts',(-19.2636127006401,2.59466439904151,4.43590837508125));
#86376=CARTESIAN_POINT('Ctrl Pts',(-19.0266681339242,-2.29642021014399,
4.59739279965534));
#86377=CARTESIAN_POINT('Ctrl Pts',(-18.7897235672083,-5.10505959163747,
0.58985851863619));
#86378=CARTESIAN_POINT('Ctrl Pts',(-18.5527790004924,-3.2843166104229,-3.9525726867779));
#86379=CARTESIAN_POINT('Ctrl Pts',(-18.3158344337765,1.51471820104741,-4.91072247268154));
#86380=CARTESIAN_POINT('Ctrl Pts',(-18.0788898670606,4.94017263751959,-1.41571916940714));
#86381=CARTESIAN_POINT('Ctrl Pts',(-17.8419453003447,3.88576790984695,3.36308997731261));
#86382=CARTESIAN_POINT('Ctrl Pts',(-17.6050007336288,-0.692338161950112,
5.09217382990313));
#86383=CARTESIAN_POINT('Ctrl Pts',(-17.3680561669129,-4.64261648732419,
2.20356043689236));
#86384=CARTESIAN_POINT('Ctrl Pts',(-17.131111600197,-4.38286623037431,-2.68329089970427));
#86385=CARTESIAN_POINT('Ctrl Pts',(-16.8941670334811,-0.1486347406669,-5.13687396767488));
#86386=CARTESIAN_POINT('Ctrl Pts',(-16.6572224667652,4.22038206001104,-2.93222470384142));
#86387=CARTESIAN_POINT('Ctrl Pts',(-16.4202779000492,4.76226191148954,1.93143157590774));
#86388=CARTESIAN_POINT('Ctrl Pts',(-16.1833333333333,0.985616031484506,
5.04362245658377));
#86389=CARTESIAN_POINT('Ctrl Pts',(-15.9463887666174,-3.6848085344759,3.58214356361848));
#86390=CARTESIAN_POINT('Ctrl Pts',(-15.7094441999015,-5.01376621608183,
-1.12770331938881));
#86391=CARTESIAN_POINT('Ctrl Pts',(-15.4724996331856,-1.7961284314291,-4.81492358235354));
#86392=CARTESIAN_POINT('Ctrl Pts',(-15.2355550664697,3.05027883134127,-4.13586333153898));
#86393=CARTESIAN_POINT('Ctrl Pts',(-14.9986104997538,5.13062495210321,0.293690393013142));
#86394=CARTESIAN_POINT('Ctrl Pts',(-14.7616659330379,2.55840548823495,4.45691909325972));
#86395=CARTESIAN_POINT('Ctrl Pts',(-14.524721366322,-2.33383335674485,4.57851376639182));
#86396=CARTESIAN_POINT('Ctrl Pts',(-14.2877767996061,-5.10969985776604,
0.548209640228335));
#86397=CARTESIAN_POINT('Ctrl Pts',(-14.0508322328902,-3.25197611822812,
-3.97922326246816));
#86398=CARTESIAN_POINT('Ctrl Pts',(-13.8138876661743,1.55471237920095,-4.89820741333533));
#86399=CARTESIAN_POINT('Ctrl Pts',(-13.5769430994583,4.95155288013896,-1.37538740770787));
#86400=CARTESIAN_POINT('Ctrl Pts',(-13.3399985327425,3.85821436084477,3.3946646950568));
#86401=CARTESIAN_POINT('Ctrl Pts',(-13.1030539660265,-0.733839328817908,
5.0863588435711));
#86402=CARTESIAN_POINT('Ctrl Pts',(-12.8661093993107,-4.66043108396379,
2.16562890581881));
#86403=CARTESIAN_POINT('Ctrl Pts',(-12.6291648325947,-4.36083958205737,
-2.718941813584));
#86404=CARTESIAN_POINT('Ctrl Pts',(-12.3922202658788,-0.106741105077996,
-5.13791521753527));
#86405=CARTESIAN_POINT('Ctrl Pts',(-12.1552756991629,4.24415259598959,-2.89771206092819));
#86406=CARTESIAN_POINT('Ctrl Pts',(-11.918331132447,4.74635369364874,1.97020127420546));
#86407=CARTESIAN_POINT('Ctrl Pts',(-11.6813865657311,0.944454987929595,
5.05149197978862));
#86408=CARTESIAN_POINT('Ctrl Pts',(-11.4444419990152,-3.71389664781181,
3.55197665187513));
#86409=CARTESIAN_POINT('Ctrl Pts',(-11.2074974322993,-5.00440364673143,
-1.16855063504964));
#86410=CARTESIAN_POINT('Ctrl Pts',(-10.9705528655834,-1.75680536690942,
-4.82941004149492));
#86411=CARTESIAN_POINT('Ctrl Pts',(-10.7336082988675,3.08390335565245,-4.11085228864884));
#86412=CARTESIAN_POINT('Ctrl Pts',(-10.4966637321515,5.12805946468642,0.335518364227643));
#86413=CARTESIAN_POINT('Ctrl Pts',(-10.2597191654357,2.52197643052209,4.4776334519459));
#86414=CARTESIAN_POINT('Ctrl Pts',(-10.0227745987197,-2.37109129954888,
4.55933026828472));
#86415=CARTESIAN_POINT('Ctrl Pts',(-9.78583003200384,-5.11400034889696,
0.506524310942766));
#86416=CARTESIAN_POINT('Ctrl Pts',(-9.54888546528793,-3.21941937603737,
-4.00560923297429));
#86417=CARTESIAN_POINT('Ctrl Pts',(-9.31194089857203,1.59460317192763,-4.88536663620762));
#86418=CARTESIAN_POINT('Ctrl Pts',(-9.07499633185612,4.96260385937652,-1.33496418715956));
#86419=CARTESIAN_POINT('Ctrl Pts',(-8.83805176514022,3.83040425118085,3.42601367753078));
#86420=CARTESIAN_POINT('Ctrl Pts',(-8.60110719842429,-0.775291697251443,
5.0802056287376));
#86421=CARTESIAN_POINT('Ctrl Pts',(-8.36416263170841,-4.67793577532945,
2.12755336666615));
#86422=CARTESIAN_POINT('Ctrl Pts',(-8.12721806499248,-4.33852295027593,
-2.75441192562119));
#86423=CARTESIAN_POINT('Ctrl Pts',(-7.8902734982766,-0.0648403715470012,
-5.13861481065229));
#86424=CARTESIAN_POINT('Ctrl Pts',(-7.65332893156067,4.26764090794638,-2.8630067284419));
#86425=CARTESIAN_POINT('Ctrl Pts',(-7.41638436484477,4.7301298567781,2.00883995975922));
#86426=CARTESIAN_POINT('Ctrl Pts',(-7.17943979812886,0.903231140868191,
5.05902559313128));
#86427=CARTESIAN_POINT('Ctrl Pts',(-6.94249523141296,-3.74273779771181,
3.52157354388502));
#86428=CARTESIAN_POINT('Ctrl Pts',(-6.70555066469705,-4.99470829859922,
-1.20932024557051));
#86429=CARTESIAN_POINT('Ctrl Pts',(-6.46860609798114,-1.71736548022594,
-4.84357535835101));
#86430=CARTESIAN_POINT('Ctrl Pts',(-6.23166153126523,3.11732280992082,-4.0855678863374));
#86431=CARTESIAN_POINT('Ctrl Pts',(-5.99471696454932,5.12515297450633,0.377324025464465));
#86432=CARTESIAN_POINT('Ctrl Pts',(-5.75777239783342,2.48537967129977,4.49805005877574));
#86433=CARTESIAN_POINT('Ctrl Pts',(-5.52082783111751,-2.40819157679517,
4.53984359153818));
#86434=CARTESIAN_POINT('Ctrl Pts',(-5.28388326440161,-5.11796076348032,
0.464805291876296));
#86435=CARTESIAN_POINT('Ctrl Pts',(-5.04693869768569,-3.18664857103844,
-4.03172882774475));
#86436=CARTESIAN_POINT('Ctrl Pts',(-4.8099941309698,1.63438796537354,-4.87220102328648));
#86437=CARTESIAN_POINT('Ctrl Pts',(-4.57304956425387,4.97332476795878,-1.29445214310224));
#86438=CARTESIAN_POINT('Ctrl Pts',(-4.33610499753798,3.80233956820685,3.45713473956928));
#86439=CARTESIAN_POINT('Ctrl Pts',(-4.09916043082206,-0.816692775494692,
5.07371478740984));
#86440=CARTESIAN_POINT('Ctrl Pts',(-3.86221586410616,-4.6951288890806,2.08933598101334));
#86441=CARTESIAN_POINT('Ctrl Pts',(-3.62527129739025,-4.31591879559353,
-2.78969816567315));
#86442=CARTESIAN_POINT('Ctrl Pts',(-3.38832673067434,-0.0229334500078643,
-5.13897406752435));
#86443=CARTESIAN_POINT('Ctrl Pts',(-3.15138216395844,4.29084182872829,-2.82810838756633));
#86444=CARTESIAN_POINT('Ctrl Pts',(-2.91443759724252,4.71359840696839,2.04734001631884));
#86445=CARTESIAN_POINT('Ctrl Pts',(-2.67749303052663,0.861933921267414,
5.06623249294253));
#86446=CARTESIAN_POINT('Ctrl Pts',(-2.44054846381071,-3.77130449135365,
3.49091762858201));
#86447=CARTESIAN_POINT('Ctrl Pts',(-2.20360389709481,-4.98472995723955,
-1.2499736380601));
#86448=CARTESIAN_POINT('Ctrl Pts',(-1.9666593303789,-1.67771697248142,-4.85748738223137));
#86449=CARTESIAN_POINT('Ctrl Pts',(-1.729714763663,3.15035354388312,-4.05987962632826));
#86450=CARTESIAN_POINT('Ctrl Pts',(-1.49277019694709,5.12225430095726,0.418850610185909));
#86451=CARTESIAN_POINT('Ctrl Pts',(-1.25582563023118,2.44794756804106,4.51865567952482));
#86452=CARTESIAN_POINT('Ctrl Pts',(-1.01888106351527,-2.44384225364839,
4.51911617817157));
#86453=CARTESIAN_POINT('Ctrl Pts',(-0.781936496799366,-5.12407657510525,
0.424868130349103));
#86454=CARTESIAN_POINT('Ctrl Pts',(-0.544991930083454,-3.14870294440949,
-4.06114495196868));
#86455=CARTESIAN_POINT('Ctrl Pts',(-0.347538124486872,0.861031357136043,
-4.7194698267761));
#86456=CARTESIAN_POINT('Ctrl Pts',(-0.189575080009593,3.34110011276904,
-3.06042877319883));
#86457=CARTESIAN_POINT('Ctrl Pts',(-0.110593557770963,4.04792784467689,
-1.7613235919546));
#86458=CARTESIAN_POINT('Ctrl Pts',(-0.0711027966516446,4.2237088282277,
-1.06264395673989));
#86459=CARTESIAN_POINT('Ctrl Pts',(-24.075,2.36230756092323,-3.31488661006752));
#86460=CARTESIAN_POINT('Ctrl Pts',(-24.0355092388807,2.91065117590484,-2.92411720524959));
#86461=CARTESIAN_POINT('Ctrl Pts',(-23.956527716642,3.8009161537758,-1.86677512529004));
#86462=CARTESIAN_POINT('Ctrl Pts',(-23.7985646721648,4.40104888295471,0.856562345338821));
#86463=CARTESIAN_POINT('Ctrl Pts',(-23.6011108665681,2.46349467463415,4.12278630825743));
#86464=CARTESIAN_POINT('Ctrl Pts',(-23.3641662998523,-2.11355533076443,
4.31564323485309));
#86465=CARTESIAN_POINT('Ctrl Pts',(-23.1272217331364,-4.76528500937787,
0.589368033154422));
#86466=CARTESIAN_POINT('Ctrl Pts',(-22.8902771664205,-3.1002006861113,-3.66850893344406));
#86467=CARTESIAN_POINT('Ctrl Pts',(-22.6533325997046,1.37852450357098,-4.60117581069992));
#86468=CARTESIAN_POINT('Ctrl Pts',(-22.4163880329887,4.60597174073038,-1.36062610156221));
#86469=CARTESIAN_POINT('Ctrl Pts',(-22.1794434662727,3.65724566378385,3.11337055406841));
#86470=CARTESIAN_POINT('Ctrl Pts',(-21.9424988995569,-0.608277930885338,
4.76430086728238));
#86471=CARTESIAN_POINT('Ctrl Pts',(-21.7055543328409,-4.32203219920287,
2.09474833835713));
#86472=CARTESIAN_POINT('Ctrl Pts',(-21.468609766125,-4.11655899594451,-2.47431260611472));
#86473=CARTESIAN_POINT('Ctrl Pts',(-21.2316651994091,-0.178052071836572,
-4.79964076861094));
#86474=CARTESIAN_POINT('Ctrl Pts',(-20.9947206326932,3.92189259497827,-2.77253197087948));
#86475=CARTESIAN_POINT('Ctrl Pts',(-20.7577760659773,4.46538966209699,1.76876296315944));
#86476=CARTESIAN_POINT('Ctrl Pts',(-20.5208314992614,0.959564937147886,
4.70610816747424));
#86477=CARTESIAN_POINT('Ctrl Pts',(-20.2838869325455,-3.41641139423198,
3.37584696374503));
#86478=CARTESIAN_POINT('Ctrl Pts',(-20.0469423658296,-4.69431112832445,
-1.01570673574804));
#86479=CARTESIAN_POINT('Ctrl Pts',(-19.8099977991137,-1.71530351140438,
-4.48619540698215));
#86480=CARTESIAN_POINT('Ctrl Pts',(-19.5730532323978,2.8191792622351,-3.88850133137423));
#86481=CARTESIAN_POINT('Ctrl Pts',(-19.3361086656818,4.79716740439492,0.23537265996686));
#86482=CARTESIAN_POINT('Ctrl Pts',(-19.099164098966,2.42497660407891,4.14580553515268));
#86483=CARTESIAN_POINT('Ctrl Pts',(-18.86221953225,-2.14623721078936,4.29672908104936));
#86484=CARTESIAN_POINT('Ctrl Pts',(-18.6252749655341,-4.77119510204201,
0.551282511887758));
#86485=CARTESIAN_POINT('Ctrl Pts',(-18.3883303988183,-3.06952642646402,
-3.69407939419781));
#86486=CARTESIAN_POINT('Ctrl Pts',(-18.1513858321023,1.41565753192185,-4.58956738674043));
#86487=CARTESIAN_POINT('Ctrl Pts',(-17.9144412653864,4.61709154776294,-1.32313291269056));
#86488=CARTESIAN_POINT('Ctrl Pts',(-17.6774966986705,3.63164356582701,3.14314811403285));
#86489=CARTESIAN_POINT('Ctrl Pts',(-17.4405521319546,-0.647060115157983,
4.75915205295132));
#86490=CARTESIAN_POINT('Ctrl Pts',(-17.2036075652387,-4.33899519630793,
2.05945035015389));
#86491=CARTESIAN_POINT('Ctrl Pts',(-16.9666629985228,-4.09623228013284,
-2.50780704283935));
#86492=CARTESIAN_POINT('Ctrl Pts',(-16.7297184318069,-0.138914215188535,
-4.80092885781891));
#86493=CARTESIAN_POINT('Ctrl Pts',(-16.492773865091,3.94437437056674,-2.74046088863915));
#86494=CARTESIAN_POINT('Ctrl Pts',(-16.2558292983751,4.45081595990773,1.8051183751108));
#86495=CARTESIAN_POINT('Ctrl Pts',(-16.0188847316592,0.921157980137197,
4.71377587850701));
#86496=CARTESIAN_POINT('Ctrl Pts',(-15.7819401649433,-3.44382668136788,
3.34787587074291));
#86497=CARTESIAN_POINT('Ctrl Pts',(-15.5449955982273,-4.68587219865936,
-1.05395293775576));
#86498=CARTESIAN_POINT('Ctrl Pts',(-15.3080510315115,-1.6786638864531,-4.50003362359639));
#86499=CARTESIAN_POINT('Ctrl Pts',(-15.0711064647955,2.85079442437809,-3.86538306085168));
#86500=CARTESIAN_POINT('Ctrl Pts',(-14.8341618980796,4.79508852002207,0.274483409940331));
#86501=CARTESIAN_POINT('Ctrl Pts',(-14.5972173313637,2.39108898052815,4.16544217873422));
#86502=CARTESIAN_POINT('Ctrl Pts',(-14.3602727646478,-2.18120358456222,
4.27908471286496));
#86503=CARTESIAN_POINT('Ctrl Pts',(-14.1233281979319,-4.77553190059009,
0.512357417851518));
#86504=CARTESIAN_POINT('Ctrl Pts',(-13.886383631216,-3.0393009618661,-3.71898705568882));
#86505=CARTESIAN_POINT('Ctrl Pts',(-13.6494390645001,1.45303614102348,-4.57787079656698));
#86506=CARTESIAN_POINT('Ctrl Pts',(-13.4124944977842,4.6277275367991,-1.28543879758337));
#86507=CARTESIAN_POINT('Ctrl Pts',(-13.1755499310683,3.6058919843453,3.17265788486808));
#86508=CARTESIAN_POINT('Ctrl Pts',(-12.9386053643524,-0.68584715780348,
4.75371735942664));
#86509=CARTESIAN_POINT('Ctrl Pts',(-12.7016607976364,-4.35564474068758,
2.02399949360218));
#86510=CARTESIAN_POINT('Ctrl Pts',(-12.4647162309206,-4.07564614696872,
-2.54112643169917));
#86511=CARTESIAN_POINT('Ctrl Pts',(-12.2277716642046,-0.0997603707836814,
-4.80190201124536));
#86512=CARTESIAN_POINT('Ctrl Pts',(-11.9908270974887,3.96659034332826,-2.70820532925335));
#86513=CARTESIAN_POINT('Ctrl Pts',(-11.7538825307728,4.43594811954626,1.84135258380226));
#86514=CARTESIAN_POINT('Ctrl Pts',(-11.5169379640569,0.882688817166835,
4.72113074477184));
#86515=CARTESIAN_POINT('Ctrl Pts',(-11.279993397341,-3.47101246860204,3.31968183716308));
#86516=CARTESIAN_POINT('Ctrl Pts',(-11.0430488306251,-4.67712192959289,
-1.09212889024254));
#86517=CARTESIAN_POINT('Ctrl Pts',(-10.8061042639092,-1.64191250099602,
-4.51357268649284));
#86518=CARTESIAN_POINT('Ctrl Pts',(-10.5691596971933,2.88221994700369,-3.84200770877353));
#86519=CARTESIAN_POINT('Ctrl Pts',(-10.3322151304774,4.79269081226222,0.313575884338453));
#86520=CARTESIAN_POINT('Ctrl Pts',(-10.0952705637615,2.35704233746519,4.18480184436228));
#86521=CARTESIAN_POINT('Ctrl Pts',(-9.85832599704557,-2.21602490467178,
4.26115579145559));
#86522=CARTESIAN_POINT('Ctrl Pts',(-9.62138143032966,-4.77955114499888,
0.473398256779212));
#86523=CARTESIAN_POINT('Ctrl Pts',(-9.38443686361375,-3.00887338975049,
-3.74364741684263));
#86524=CARTESIAN_POINT('Ctrl Pts',(-9.14749229689786,1.49031812597541,-4.56586979014612));
#86525=CARTESIAN_POINT('Ctrl Pts',(-8.91054773018194,4.63805579586533,-1.24765920492107));
#86526=CARTESIAN_POINT('Ctrl Pts',(-8.67360316346604,3.57990062094709,3.20195668323646));
#86527=CARTESIAN_POINT('Ctrl Pts',(-8.43665859675013,-0.724588593371072,
4.74796655711994));
#86528=CARTESIAN_POINT('Ctrl Pts',(-8.19971403003422,-4.37200464720922,
1.98841404691898));
#86529=CARTESIAN_POINT('Ctrl Pts',(-7.96276946331832,-4.05478899489471,
-2.57427684293));
#86530=CARTESIAN_POINT('Ctrl Pts',(-7.7258248966024,-0.0605998926332336,
-4.80255585185065));
#86531=CARTESIAN_POINT('Ctrl Pts',(-7.48888032988651,3.98854254916481,-2.67576968195071));
#86532=CARTESIAN_POINT('Ctrl Pts',(-7.25193576317058,4.42078530124335,1.87746434781877));
#86533=CARTESIAN_POINT('Ctrl Pts',(-7.01499119645469,0.844160957960478,
4.72817166925782));
#86534=CARTESIAN_POINT('Ctrl Pts',(-6.77804662973878,-3.49796744349901,
3.29126705427458));
#86535=CARTESIAN_POINT('Ctrl Pts',(-6.54110206302287,-4.66806064505926,
-1.13023221940798));
#86536=CARTESIAN_POINT('Ctrl Pts',(-6.30415749630696,-1.60505193339804,
-4.52681160940636));
#86537=CARTESIAN_POINT('Ctrl Pts',(-6.06721292959105,2.91345381090988,-3.81837687463714));
#86538=CARTESIAN_POINT('Ctrl Pts',(-5.83026836287515,4.78997440289178,0.352647507803434));
#86539=CARTESIAN_POINT('Ctrl Pts',(-5.59332379615923,2.322838960361,4.20388323073168));
#86540=CARTESIAN_POINT('Ctrl Pts',(-5.35637922944334,-2.25069887035317,
4.24294351890926));
#86541=CARTESIAN_POINT('Ctrl Pts',(-5.11943466272741,-4.78325255343947,
0.434407609195393));
#86542=CARTESIAN_POINT('Ctrl Pts',(-4.88249009601153,-2.9782457542657,-3.76805882289953));
#86543=CARTESIAN_POINT('Ctrl Pts',(-4.6455455292956,1.52750104386647,-4.55356519178499));
#86544=CARTESIAN_POINT('Ctrl Pts',(-4.40860096257971,4.64807557048283,-1.20979659769575));
#86545=CARTESIAN_POINT('Ctrl Pts',(-4.17165639586379,3.55367133301375,3.23104246687973));
#86546=CARTESIAN_POINT('Ctrl Pts',(-3.93471182914789,-0.763282093062437,
4.74190020866793));
#86547=CARTESIAN_POINT('Ctrl Pts',(-3.69776726243198,-4.38807335290126,
1.9526960303187));
#86548=CARTESIAN_POINT('Ctrl Pts',(-3.46082269571607,-4.03366312355658,
-2.60725540717266));
#86549=CARTESIAN_POINT('Ctrl Pts',(-3.22387812900017,-0.021433631162604,
-4.80289161377419));
#86550=CARTESIAN_POINT('Ctrl Pts',(-2.98693356228425,4.01022615884859,-2.64315364876519));
#86551=CARTESIAN_POINT('Ctrl Pts',(-2.74998899556836,4.40533498750148,1.91344654900335));
#86552=CARTESIAN_POINT('Ctrl Pts',(-2.51304442885244,0.805564524686711,
4.73490724686727));
#86553=CARTESIAN_POINT('Ctrl Pts',(-2.27609986213654,-3.52466591123261,
3.26261599735412));
#86554=CARTESIAN_POINT('Ctrl Pts',(-2.03915529542063,-4.65873487470004,
-1.16822693105551));
#86555=CARTESIAN_POINT('Ctrl Pts',(-1.80221072870472,-1.56799638829454,
-4.53981380438684));
#86556=CARTESIAN_POINT('Ctrl Pts',(-1.56526616198882,2.94432437633009,-3.79436859458956));
#86557=CARTESIAN_POINT('Ctrl Pts',(-1.32832159527291,4.78726529895451,0.391458306006858));
#86558=CARTESIAN_POINT('Ctrl Pts',(-1.091377028557,2.2878548696719,4.22314126974725));
#86559=CARTESIAN_POINT('Ctrl Pts',(-0.854432461841093,-2.28401803768771,
4.22357165236047));
#86560=CARTESIAN_POINT('Ctrl Pts',(-0.617487895125189,-4.78896839866047,
0.397082287904312));
#86561=CARTESIAN_POINT('Ctrl Pts',(-0.380543328409276,-2.94278172399022,
-3.79555116952135));
#86562=CARTESIAN_POINT('Ctrl Pts',(-0.183089522812695,0.804720987116727,
-4.41082242382338));
#86563=CARTESIAN_POINT('Ctrl Pts',(-0.0251264783354149,3.1225963590295,
-2.860280572778));
#86564=CARTESIAN_POINT('Ctrl Pts',(0.0538550439032153,3.78319844445675,
-1.64613523979437));
#86565=CARTESIAN_POINT('Ctrl Pts',(0.0933458050225333,3.94748357231767,
-0.993148375763724));
#86566=CARTESIAN_POINT('Ctrl Pts',(-0.400000000000003,4.77615934004775,
-1.20163511869228));
#86567=CARTESIAN_POINT('Ctrl Pts',(-0.439490761119319,4.57738664511713,
-1.99170029627507));
#86568=CARTESIAN_POINT('Ctrl Pts',(-0.478981522238631,4.17774713268266,
-2.72621273515775));
#86569=CARTESIAN_POINT('Ctrl Pts',(-0.518472283357947,3.62737043608126,
-3.32797388692922));
#86570=CARTESIAN_POINT('Ctrl Pts',(-0.557963044477266,3.07699373947981,
-3.92973503870074));
#86571=CARTESIAN_POINT('Ctrl Pts',(-0.597453805596586,2.37587985871143,
-4.39874490336101));
#86572=CARTESIAN_POINT('Ctrl Pts',(-0.636944566715907,1.60619077270431,
-4.66178933874665));
#86573=CARTESIAN_POINT('Ctrl Pts',(-0.715926088954544,0.0668126006901387,
-5.1878782095179));
#86574=CARTESIAN_POINT('Ctrl Pts',(-0.794907611193176,-1.74686639227891,
-4.89010536319065));
#86575=CARTESIAN_POINT('Ctrl Pts',(-0.873889133431811,-3.02599714588792,
-3.89575688467669));
#86576=CARTESIAN_POINT('Ctrl Pts',(-0.946312246986672,-4.19891239485264,
-2.98397637283827));
#86577=CARTESIAN_POINT('Ctrl Pts',(-1.01873536054154,-4.92236843052219,
-1.48650066533691));
#86578=CARTESIAN_POINT('Ctrl Pts',(-1.0911584740964,-4.93200687334489,0.00268308223936954));
#86579=CARTESIAN_POINT('Origin',(-0.4,0.,0.));
#86580=CARTESIAN_POINT('',(0.,-6.52124420545966E-16,5.325));
#86581=CARTESIAN_POINT('Origin',(-0.4,-6.52124420545966E-16,5.325));
#86582=CARTESIAN_POINT('Origin',(0.,0.,0.));
#86583=CARTESIAN_POINT('Origin',(-0.4,0.,0.));
#86584=CARTESIAN_POINT('Origin',(-12.,0.,0.));
#86585=CARTESIAN_POINT('Origin',(0.,8.,0.));
#86586=CARTESIAN_POINT('',(0.,-8.,-9.79717439317883E-16));
#86587=CARTESIAN_POINT('Origin',(0.,0.,0.));
#86588=CARTESIAN_POINT('Origin',(0.3,7.53377931054339,-1.32840855915202));
#86589=CARTESIAN_POINT('',(0.3,7.84576201581982,-1.56333566169231));
#86590=CARTESIAN_POINT('',(9.,7.84576201581982,-1.56333566169231));
#86591=CARTESIAN_POINT('',(4.5,7.84576201581982,-1.56333566169231));
#86592=CARTESIAN_POINT('',(0.3,7.53377931054339,-1.32840855915202));
#86593=CARTESIAN_POINT('',(0.3,8.02680208495337,-1.69966122771225));
#86594=CARTESIAN_POINT('',(9.,7.53377931054339,-1.32840855915202));
#86595=CARTESIAN_POINT('',(0.3,7.53377931054339,-1.32840855915202));
#86596=CARTESIAN_POINT('',(9.,8.02680208495337,-1.69966122771225));
#86597=CARTESIAN_POINT('Origin',(9.,7.80460144262175,-1.37616180801042));
#86598=CARTESIAN_POINT('',(9.,7.90729695778639,-1.21435366404606));
#86599=CARTESIAN_POINT('Origin',(9.,0.,0.));
#86600=CARTESIAN_POINT('',(9.,7.53377931054339,-1.32840855915202));
#86601=CARTESIAN_POINT('Origin',(0.3,8.12404506444685,-1.14816888602541));
#86602=CARTESIAN_POINT('',(0.3,7.90729695778639,-1.21435366404606));
#86603=CARTESIAN_POINT('',(4.5,7.90729695778639,-1.21435366404606));
#86604=CARTESIAN_POINT('',(0.3,7.53377931054339,-1.32840855915202));
#86605=CARTESIAN_POINT('Origin',(0.3,7.80460144262175,-1.37616180801042));
#86606=CARTESIAN_POINT('Origin',(0.3,0.,0.));
#86607=CARTESIAN_POINT('Origin',(0.3,7.1886485490122,-2.61645409644137));
#86608=CARTESIAN_POINT('',(0.3,7.45509687273345,-2.9019873566506));
#86609=CARTESIAN_POINT('',(9.,7.45509687273345,-2.9019873566506));
#86610=CARTESIAN_POINT('',(4.5,7.45509687273345,-2.9019873566506));
#86611=CARTESIAN_POINT('',(0.3,7.1886485490122,-2.61645409644137));
#86612=CARTESIAN_POINT('',(0.3,7.60971385031326,-3.06767910909054));
#86613=CARTESIAN_POINT('',(9.,7.1886485490122,-2.61645409644137));
#86614=CARTESIAN_POINT('',(0.3,7.1886485490122,-2.61645409644137));
#86615=CARTESIAN_POINT('',(9.,7.60971385031326,-3.06767910909054));
#86616=CARTESIAN_POINT('Origin',(9.,7.44706401972832,-2.71050963585593));
#86617=CARTESIAN_POINT('',(9.,7.57629704859312,-2.56899261024222));
#86618=CARTESIAN_POINT('Origin',(9.,0.,0.));
#86619=CARTESIAN_POINT('',(9.,7.1886485490122,-2.61645409644137));
#86620=CARTESIAN_POINT('Origin',(0.3,7.80124513057563,-2.54145124145043));
#86621=CARTESIAN_POINT('',(0.3,7.57629704859312,-2.56899261024222));
#86622=CARTESIAN_POINT('',(4.5,7.57629704859312,-2.56899261024222));
#86623=CARTESIAN_POINT('',(0.3,7.1886485490122,-2.61645409644137));
#86624=CARTESIAN_POINT('Origin',(0.3,7.44706401972832,-2.71050963585593));
#86625=CARTESIAN_POINT('Origin',(0.3,0.,0.));
#86626=CARTESIAN_POINT('Origin',(0.3,6.62509433895095,-3.825));
#86627=CARTESIAN_POINT('',(0.3,6.83791238363012,-4.15246363425351));
#86628=CARTESIAN_POINT('',(9.,6.83791238363012,-4.15246363425351));
#86629=CARTESIAN_POINT('',(4.5,6.83791238363012,-4.15246363425351));
#86630=CARTESIAN_POINT('',(0.3,6.62509433895095,-3.825));
#86631=CARTESIAN_POINT('',(0.3,6.96140831103239,-4.34248711305965));
#86632=CARTESIAN_POINT('',(9.,6.62509433895095,-3.825));
#86633=CARTESIAN_POINT('',(0.3,6.62509433895095,-3.825));
#86634=CARTESIAN_POINT('',(9.,6.96140831103239,-4.34248711305965));
#86635=CARTESIAN_POINT('Origin',(9.,6.86325132499167,-3.9625));
#86636=CARTESIAN_POINT('',(9.,7.01509518736965,-3.84557401594914));
#86637=CARTESIAN_POINT('Origin',(9.,0.,0.));
#86638=CARTESIAN_POINT('',(9.,6.62509433895095,-3.825));
#86639=CARTESIAN_POINT('Origin',(0.3,7.24140831103239,-3.85751288694036));
#86640=CARTESIAN_POINT('',(0.3,7.01509518736965,-3.84557401594914));
#86641=CARTESIAN_POINT('',(4.5,7.01509518736965,-3.84557401594914));
#86642=CARTESIAN_POINT('',(0.3,6.62509433895095,-3.825));
#86643=CARTESIAN_POINT('Origin',(0.3,6.86325132499167,-3.9625));
#86644=CARTESIAN_POINT('Origin',(0.3,0.,0.));
#86645=CARTESIAN_POINT('Origin',(0.3,5.86023998986018,-4.91732521410203));
#86646=CARTESIAN_POINT('',(0.3,6.01296138690081,-5.27676940557761));
#86647=CARTESIAN_POINT('',(9.,6.01296138690081,-5.27676940557761));
#86648=CARTESIAN_POINT('',(4.5,6.01296138690081,-5.27676940557761));
#86649=CARTESIAN_POINT('',(0.3,5.86023998986018,-4.91732521410203));
#86650=CARTESIAN_POINT('',(0.3,6.10158390286339,-5.48535084350294));
#86651=CARTESIAN_POINT('',(9.,5.86023998986018,-4.91732521410203));
#86652=CARTESIAN_POINT('',(0.3,5.86023998986018,-4.91732521410203));
#86653=CARTESIAN_POINT('',(9.,6.10158390286339,-5.48535084350294));
#86654=CARTESIAN_POINT('Origin',(9.,6.0709022117179,-5.09409180676583));
#86655=CARTESIAN_POINT('',(9.,6.24074320868739,-5.0053096011358));
#86656=CARTESIAN_POINT('Origin',(9.,0.,0.));
#86657=CARTESIAN_POINT('',(9.,5.86023998986018,-4.91732521410203));
#86658=CARTESIAN_POINT('Origin',(0.3,6.46154496428785,-5.05636595535631));
#86659=CARTESIAN_POINT('',(0.3,6.24074320868739,-5.0053096011358));
#86660=CARTESIAN_POINT('',(4.5,6.24074320868739,-5.0053096011358));
#86661=CARTESIAN_POINT('',(0.3,5.86023998986018,-4.91732521410203));
#86662=CARTESIAN_POINT('Origin',(0.3,6.0709022117179,-5.09409180676583));
#86663=CARTESIAN_POINT('Origin',(0.3,0.,0.));
#86664=CARTESIAN_POINT('Origin',(0.3,4.91732521410202,-5.86023998986018));
#86665=CARTESIAN_POINT('',(0.3,5.0053096011358,-6.24074320868739));
#86666=CARTESIAN_POINT('',(9.,5.0053096011358,-6.24074320868739));
#86667=CARTESIAN_POINT('',(4.5,5.0053096011358,-6.24074320868739));
#86668=CARTESIAN_POINT('',(0.3,4.91732521410202,-5.86023998986018));
#86669=CARTESIAN_POINT('',(0.3,5.05636595535631,-6.46154496428785));
#86670=CARTESIAN_POINT('',(9.,4.91732521410202,-5.86023998986018));
#86671=CARTESIAN_POINT('',(0.3,4.91732521410202,-5.86023998986018));
#86672=CARTESIAN_POINT('',(9.,5.05636595535631,-6.46154496428785));
#86673=CARTESIAN_POINT('Origin',(9.,5.09409180676582,-6.0709022117179));
#86674=CARTESIAN_POINT('',(9.,5.27676940557761,-6.01296138690081));
#86675=CARTESIAN_POINT('Origin',(9.,0.,0.));
#86676=CARTESIAN_POINT('',(9.,4.91732521410202,-5.86023998986018));
#86677=CARTESIAN_POINT('Origin',(0.3,5.48535084350294,-6.10158390286339));
#86678=CARTESIAN_POINT('',(0.3,5.27676940557761,-6.01296138690081));
#86679=CARTESIAN_POINT('',(4.5,5.27676940557761,-6.01296138690081));
#86680=CARTESIAN_POINT('',(0.3,4.91732521410202,-5.86023998986018));
#86681=CARTESIAN_POINT('Origin',(0.3,5.09409180676582,-6.0709022117179));
#86682=CARTESIAN_POINT('Origin',(0.3,0.,0.));
#86683=CARTESIAN_POINT('Origin',(0.3,3.825,-6.62509433895096));
#86684=CARTESIAN_POINT('',(0.3,3.84557401594914,-7.01509518736965));
#86685=CARTESIAN_POINT('',(9.,3.84557401594914,-7.01509518736965));
#86686=CARTESIAN_POINT('',(4.5,3.84557401594914,-7.01509518736965));
#86687=CARTESIAN_POINT('',(0.3,3.825,-6.62509433895096));
#86688=CARTESIAN_POINT('',(0.3,3.85751288694036,-7.2414083110324));
#86689=CARTESIAN_POINT('',(9.,3.825,-6.62509433895096));
#86690=CARTESIAN_POINT('',(0.3,3.825,-6.62509433895096));
#86691=CARTESIAN_POINT('',(9.,3.85751288694036,-7.2414083110324));
#86692=CARTESIAN_POINT('Origin',(9.,3.9625,-6.86325132499168));
#86693=CARTESIAN_POINT('',(9.,4.15246363425351,-6.83791238363012));
#86694=CARTESIAN_POINT('Origin',(9.,0.,0.));
#86695=CARTESIAN_POINT('',(9.,3.825,-6.62509433895096));
#86696=CARTESIAN_POINT('Origin',(0.3,4.34248711305964,-6.96140831103239));
#86697=CARTESIAN_POINT('',(0.3,4.15246363425351,-6.83791238363012));
#86698=CARTESIAN_POINT('',(4.5,4.15246363425351,-6.83791238363012));
#86699=CARTESIAN_POINT('',(0.3,3.825,-6.62509433895096));
#86700=CARTESIAN_POINT('Origin',(0.3,3.9625,-6.86325132499168));
#86701=CARTESIAN_POINT('Origin',(0.3,0.,0.));
#86702=CARTESIAN_POINT('Origin',(0.3,2.61645409644136,-7.1886485490122));
#86703=CARTESIAN_POINT('',(0.3,2.56899261024221,-7.57629704859313));
#86704=CARTESIAN_POINT('',(9.,2.56899261024221,-7.57629704859313));
#86705=CARTESIAN_POINT('',(4.5,2.56899261024221,-7.57629704859313));
#86706=CARTESIAN_POINT('',(0.3,2.61645409644136,-7.1886485490122));
#86707=CARTESIAN_POINT('',(0.3,2.54145124145042,-7.80124513057564));
#86708=CARTESIAN_POINT('',(9.,2.61645409644136,-7.1886485490122));
#86709=CARTESIAN_POINT('',(0.3,2.61645409644136,-7.1886485490122));
#86710=CARTESIAN_POINT('',(9.,2.54145124145042,-7.80124513057564));
#86711=CARTESIAN_POINT('Origin',(9.,2.71050963585592,-7.44706401972833));
#86712=CARTESIAN_POINT('',(9.,2.90198735665059,-7.45509687273345));
#86713=CARTESIAN_POINT('Origin',(9.,0.,0.));
#86714=CARTESIAN_POINT('',(9.,2.61645409644136,-7.1886485490122));
#86715=CARTESIAN_POINT('Origin',(0.3,3.06767910909053,-7.60971385031326));
#86716=CARTESIAN_POINT('',(0.3,2.90198735665059,-7.45509687273345));
#86717=CARTESIAN_POINT('',(4.5,2.90198735665059,-7.45509687273345));
#86718=CARTESIAN_POINT('',(0.3,2.61645409644136,-7.1886485490122));
#86719=CARTESIAN_POINT('Origin',(0.3,2.71050963585592,-7.44706401972833));
#86720=CARTESIAN_POINT('Origin',(0.3,0.,0.));
#86721=CARTESIAN_POINT('Origin',(0.3,1.32840855915201,-7.53377931054339));
#86722=CARTESIAN_POINT('',(0.3,1.21435366404606,-7.90729695778639));
#86723=CARTESIAN_POINT('',(9.,1.21435366404606,-7.90729695778639));
#86724=CARTESIAN_POINT('',(4.5,1.21435366404606,-7.90729695778639));
#86725=CARTESIAN_POINT('',(0.3,1.32840855915201,-7.53377931054339));
#86726=CARTESIAN_POINT('',(0.3,1.14816888602541,-8.12404506444685));
#86727=CARTESIAN_POINT('',(9.,1.32840855915201,-7.53377931054339));
#86728=CARTESIAN_POINT('',(0.3,1.32840855915201,-7.53377931054339));
#86729=CARTESIAN_POINT('',(9.,1.14816888602541,-8.12404506444685));
#86730=CARTESIAN_POINT('Origin',(9.,1.37616180801042,-7.80460144262175));
#86731=CARTESIAN_POINT('',(9.,1.56333566169231,-7.84576201581982));
#86732=CARTESIAN_POINT('Origin',(9.,0.,0.));
#86733=CARTESIAN_POINT('',(9.,1.32840855915201,-7.53377931054339));
#86734=CARTESIAN_POINT('Origin',(0.3,1.69966122771224,-8.02680208495337));
#86735=CARTESIAN_POINT('',(0.3,1.56333566169231,-7.84576201581982));
#86736=CARTESIAN_POINT('',(4.5,1.56333566169231,-7.84576201581982));
#86737=CARTESIAN_POINT('',(0.3,1.32840855915201,-7.53377931054339));
#86738=CARTESIAN_POINT('Origin',(0.3,1.37616180801042,-7.80460144262175));
#86739=CARTESIAN_POINT('Origin',(0.3,0.,0.));
#86740=CARTESIAN_POINT('Origin',(0.3,-1.40528220202159E-15,-7.65));
#86741=CARTESIAN_POINT('',(0.3,-0.177182803739528,-7.99803765020264));
#86742=CARTESIAN_POINT('',(9.,-0.177182803739528,-7.99803765020264));
#86743=CARTESIAN_POINT('',(4.5,-0.177182803739529,-7.99803765020264));
#86744=CARTESIAN_POINT('',(0.3,-1.40528220202159E-15,-7.65));
#86745=CARTESIAN_POINT('',(0.3,-0.280000000000001,-8.2));
#86746=CARTESIAN_POINT('',(9.,-1.40528220202159E-15,-7.65));
#86747=CARTESIAN_POINT('',(0.3,-1.40528220202159E-15,-7.65));
#86748=CARTESIAN_POINT('',(9.,-0.280000000000001,-8.2));
#86749=CARTESIAN_POINT('Origin',(9.,-1.45579888248642E-15,-7.925));
#86750=CARTESIAN_POINT('',(9.,0.177182803739525,-7.99803765020264));
#86751=CARTESIAN_POINT('Origin',(9.,0.,0.));
#86752=CARTESIAN_POINT('',(9.,-1.40528220202159E-15,-7.65));
#86753=CARTESIAN_POINT('Origin',(0.3,0.279999999999998,-8.2));
#86754=CARTESIAN_POINT('',(0.3,0.177182803739525,-7.99803765020264));
#86755=CARTESIAN_POINT('',(4.5,0.177182803739526,-7.99803765020264));
#86756=CARTESIAN_POINT('',(0.3,-1.40528220202159E-15,-7.65));
#86757=CARTESIAN_POINT('Origin',(0.3,-1.45579888248642E-15,-7.925));
#86758=CARTESIAN_POINT('Origin',(0.3,0.,0.));
#86759=CARTESIAN_POINT('Origin',(0.3,-1.32840855915202,-7.53377931054339));
#86760=CARTESIAN_POINT('',(0.3,-1.56333566169232,-7.84576201581982));
#86761=CARTESIAN_POINT('',(9.,-1.56333566169232,-7.84576201581982));
#86762=CARTESIAN_POINT('',(4.5,-1.56333566169231,-7.84576201581982));
#86763=CARTESIAN_POINT('',(0.3,-1.32840855915202,-7.53377931054339));
#86764=CARTESIAN_POINT('',(0.3,-1.69966122771225,-8.02680208495337));
#86765=CARTESIAN_POINT('',(9.,-1.32840855915202,-7.53377931054339));
#86766=CARTESIAN_POINT('',(0.3,-1.32840855915202,-7.53377931054339));
#86767=CARTESIAN_POINT('',(9.,-1.69966122771225,-8.02680208495337));
#86768=CARTESIAN_POINT('Origin',(9.,-1.37616180801042,-7.80460144262175));
#86769=CARTESIAN_POINT('',(9.,-1.21435366404606,-7.90729695778639));
#86770=CARTESIAN_POINT('Origin',(9.,0.,0.));
#86771=CARTESIAN_POINT('',(9.,-1.32840855915202,-7.53377931054339));
#86772=CARTESIAN_POINT('Origin',(0.3,-1.14816888602541,-8.12404506444685));
#86773=CARTESIAN_POINT('',(0.3,-1.21435366404606,-7.90729695778639));
#86774=CARTESIAN_POINT('',(4.5,-1.21435366404606,-7.90729695778639));
#86775=CARTESIAN_POINT('',(0.3,-1.32840855915202,-7.53377931054339));
#86776=CARTESIAN_POINT('Origin',(0.3,-1.37616180801042,-7.80460144262175));
#86777=CARTESIAN_POINT('Origin',(0.3,0.,0.));
#86778=CARTESIAN_POINT('Origin',(0.3,-2.61645409644137,-7.1886485490122));
#86779=CARTESIAN_POINT('',(0.3,-2.9019873566506,-7.45509687273345));
#86780=CARTESIAN_POINT('',(9.,-2.9019873566506,-7.45509687273345));
#86781=CARTESIAN_POINT('',(4.5,-2.9019873566506,-7.45509687273345));
#86782=CARTESIAN_POINT('',(0.3,-2.61645409644137,-7.1886485490122));
#86783=CARTESIAN_POINT('',(0.3,-3.06767910909054,-7.60971385031326));
#86784=CARTESIAN_POINT('',(9.,-2.61645409644137,-7.1886485490122));
#86785=CARTESIAN_POINT('',(0.3,-2.61645409644137,-7.1886485490122));
#86786=CARTESIAN_POINT('',(9.,-3.06767910909054,-7.60971385031326));
#86787=CARTESIAN_POINT('Origin',(9.,-2.71050963585593,-7.44706401972832));
#86788=CARTESIAN_POINT('',(9.,-2.56899261024222,-7.57629704859313));
#86789=CARTESIAN_POINT('Origin',(9.,0.,0.));
#86790=CARTESIAN_POINT('',(9.,-2.61645409644137,-7.1886485490122));
#86791=CARTESIAN_POINT('Origin',(0.3,-2.54145124145043,-7.80124513057563));
#86792=CARTESIAN_POINT('',(0.3,-2.56899261024222,-7.57629704859313));
#86793=CARTESIAN_POINT('',(4.5,-2.56899261024222,-7.57629704859312));
#86794=CARTESIAN_POINT('',(0.3,-2.61645409644137,-7.1886485490122));
#86795=CARTESIAN_POINT('Origin',(0.3,-2.71050963585593,-7.44706401972832));
#86796=CARTESIAN_POINT('Origin',(0.3,0.,0.));
#86797=CARTESIAN_POINT('Origin',(0.3,-3.825,-6.62509433895095));
#86798=CARTESIAN_POINT('',(0.3,-4.15246363425351,-6.83791238363012));
#86799=CARTESIAN_POINT('',(9.,-4.15246363425351,-6.83791238363012));
#86800=CARTESIAN_POINT('',(4.5,-4.15246363425351,-6.83791238363012));
#86801=CARTESIAN_POINT('',(0.3,-3.825,-6.62509433895095));
#86802=CARTESIAN_POINT('',(0.3,-4.34248711305965,-6.96140831103239));
#86803=CARTESIAN_POINT('',(9.,-3.825,-6.62509433895095));
#86804=CARTESIAN_POINT('',(0.3,-3.825,-6.62509433895095));
#86805=CARTESIAN_POINT('',(9.,-4.34248711305965,-6.96140831103239));
#86806=CARTESIAN_POINT('Origin',(9.,-3.9625,-6.86325132499167));
#86807=CARTESIAN_POINT('',(9.,-3.84557401594914,-7.01509518736965));
#86808=CARTESIAN_POINT('Origin',(9.,0.,0.));
#86809=CARTESIAN_POINT('',(9.,-3.825,-6.62509433895095));
#86810=CARTESIAN_POINT('Origin',(0.3,-3.85751288694036,-7.24140831103239));
#86811=CARTESIAN_POINT('',(0.3,-3.84557401594914,-7.01509518736965));
#86812=CARTESIAN_POINT('',(4.5,-3.84557401594914,-7.01509518736965));
#86813=CARTESIAN_POINT('',(0.3,-3.825,-6.62509433895095));
#86814=CARTESIAN_POINT('Origin',(0.3,-3.9625,-6.86325132499167));
#86815=CARTESIAN_POINT('Origin',(0.3,0.,0.));
#86816=CARTESIAN_POINT('Origin',(0.3,-4.91732521410203,-5.86023998986018));
#86817=CARTESIAN_POINT('',(0.3,-5.27676940557761,-6.01296138690081));
#86818=CARTESIAN_POINT('',(9.,-5.27676940557761,-6.01296138690081));
#86819=CARTESIAN_POINT('',(4.5,-5.27676940557761,-6.01296138690081));
#86820=CARTESIAN_POINT('',(0.3,-4.91732521410203,-5.86023998986018));
#86821=CARTESIAN_POINT('',(0.3,-5.48535084350294,-6.10158390286339));
#86822=CARTESIAN_POINT('',(9.,-4.91732521410203,-5.86023998986018));
#86823=CARTESIAN_POINT('',(0.3,-4.91732521410203,-5.86023998986018));
#86824=CARTESIAN_POINT('',(9.,-5.48535084350294,-6.10158390286339));
#86825=CARTESIAN_POINT('Origin',(9.,-5.09409180676582,-6.0709022117179));
#86826=CARTESIAN_POINT('',(9.,-5.0053096011358,-6.24074320868739));
#86827=CARTESIAN_POINT('Origin',(9.,0.,0.));
#86828=CARTESIAN_POINT('',(9.,-4.91732521410203,-5.86023998986018));
#86829=CARTESIAN_POINT('Origin',(0.3,-5.05636595535631,-6.46154496428785));
#86830=CARTESIAN_POINT('',(0.3,-5.0053096011358,-6.24074320868739));
#86831=CARTESIAN_POINT('',(4.5,-5.0053096011358,-6.24074320868739));
#86832=CARTESIAN_POINT('',(0.3,-4.91732521410203,-5.86023998986018));
#86833=CARTESIAN_POINT('Origin',(0.3,-5.09409180676582,-6.0709022117179));
#86834=CARTESIAN_POINT('Origin',(0.3,0.,0.));
#86835=CARTESIAN_POINT('Origin',(0.3,-5.86023998986018,-4.91732521410203));
#86836=CARTESIAN_POINT('',(0.3,-6.24074320868739,-5.0053096011358));
#86837=CARTESIAN_POINT('',(9.,-6.24074320868739,-5.0053096011358));
#86838=CARTESIAN_POINT('',(4.5,-6.24074320868739,-5.0053096011358));
#86839=CARTESIAN_POINT('',(0.3,-5.86023998986018,-4.91732521410203));
#86840=CARTESIAN_POINT('',(0.3,-6.46154496428785,-5.05636595535631));
#86841=CARTESIAN_POINT('',(9.,-5.86023998986018,-4.91732521410203));
#86842=CARTESIAN_POINT('',(0.3,-5.86023998986018,-4.91732521410203));
#86843=CARTESIAN_POINT('',(9.,-6.46154496428785,-5.05636595535631));
#86844=CARTESIAN_POINT('Origin',(9.,-6.0709022117179,-5.09409180676582));
#86845=CARTESIAN_POINT('',(9.,-6.01296138690081,-5.27676940557761));
#86846=CARTESIAN_POINT('Origin',(9.,0.,0.));
#86847=CARTESIAN_POINT('',(9.,-5.86023998986018,-4.91732521410203));
#86848=CARTESIAN_POINT('Origin',(0.3,-6.10158390286339,-5.48535084350294));
#86849=CARTESIAN_POINT('',(0.3,-6.01296138690081,-5.27676940557761));
#86850=CARTESIAN_POINT('',(4.5,-6.01296138690081,-5.27676940557761));
#86851=CARTESIAN_POINT('',(0.3,-5.86023998986018,-4.91732521410203));
#86852=CARTESIAN_POINT('Origin',(0.3,-6.0709022117179,-5.09409180676582));
#86853=CARTESIAN_POINT('Origin',(0.3,0.,0.));
#86854=CARTESIAN_POINT('Origin',(0.3,-6.62509433895096,-3.825));
#86855=CARTESIAN_POINT('',(0.3,-7.01509518736965,-3.84557401594914));
#86856=CARTESIAN_POINT('',(9.,-7.01509518736965,-3.84557401594914));
#86857=CARTESIAN_POINT('',(4.5,-7.01509518736965,-3.84557401594914));
#86858=CARTESIAN_POINT('',(0.3,-6.62509433895096,-3.825));
#86859=CARTESIAN_POINT('',(0.3,-7.2414083110324,-3.85751288694035));
#86860=CARTESIAN_POINT('',(9.,-6.62509433895096,-3.825));
#86861=CARTESIAN_POINT('',(0.3,-6.62509433895096,-3.825));
#86862=CARTESIAN_POINT('',(9.,-7.2414083110324,-3.85751288694035));
#86863=CARTESIAN_POINT('Origin',(9.,-6.86325132499168,-3.9625));
#86864=CARTESIAN_POINT('',(9.,-6.83791238363012,-4.1524636342535));
#86865=CARTESIAN_POINT('Origin',(9.,0.,0.));
#86866=CARTESIAN_POINT('',(9.,-6.62509433895096,-3.825));
#86867=CARTESIAN_POINT('Origin',(0.3,-6.9614083110324,-4.34248711305964));
#86868=CARTESIAN_POINT('',(0.3,-6.83791238363012,-4.1524636342535));
#86869=CARTESIAN_POINT('',(4.5,-6.83791238363012,-4.1524636342535));
#86870=CARTESIAN_POINT('',(0.3,-6.62509433895096,-3.825));
#86871=CARTESIAN_POINT('Origin',(0.3,-6.86325132499168,-3.9625));
#86872=CARTESIAN_POINT('Origin',(0.3,0.,0.));
#86873=CARTESIAN_POINT('Origin',(0.3,-7.1886485490122,-2.61645409644137));
#86874=CARTESIAN_POINT('',(0.3,-7.57629704859313,-2.56899261024221));
#86875=CARTESIAN_POINT('',(9.,-7.57629704859313,-2.56899261024221));
#86876=CARTESIAN_POINT('',(4.5,-7.57629704859313,-2.56899261024221));
#86877=CARTESIAN_POINT('',(0.3,-7.1886485490122,-2.61645409644137));
#86878=CARTESIAN_POINT('',(0.3,-7.80124513057564,-2.54145124145043));
#86879=CARTESIAN_POINT('',(9.,-7.1886485490122,-2.61645409644137));
#86880=CARTESIAN_POINT('',(0.3,-7.1886485490122,-2.61645409644137));
#86881=CARTESIAN_POINT('',(9.,-7.80124513057564,-2.54145124145043));
#86882=CARTESIAN_POINT('Origin',(9.,-7.44706401972832,-2.71050963585592));
#86883=CARTESIAN_POINT('',(9.,-7.45509687273345,-2.90198735665059));
#86884=CARTESIAN_POINT('Origin',(9.,0.,0.));
#86885=CARTESIAN_POINT('',(9.,-7.1886485490122,-2.61645409644137));
#86886=CARTESIAN_POINT('Origin',(0.3,-7.60971385031326,-3.06767910909054));
#86887=CARTESIAN_POINT('',(0.3,-7.45509687273345,-2.90198735665059));
#86888=CARTESIAN_POINT('',(4.5,-7.45509687273345,-2.90198735665059));
#86889=CARTESIAN_POINT('',(0.3,-7.1886485490122,-2.61645409644137));
#86890=CARTESIAN_POINT('Origin',(0.3,-7.44706401972832,-2.71050963585592));
#86891=CARTESIAN_POINT('Origin',(0.3,0.,0.));
#86892=CARTESIAN_POINT('Origin',(0.3,-7.53377931054339,-1.32840855915201));
#86893=CARTESIAN_POINT('',(0.3,-7.90729695778639,-1.21435366404606));
#86894=CARTESIAN_POINT('',(9.,-7.90729695778639,-1.21435366404606));
#86895=CARTESIAN_POINT('',(4.5,-7.90729695778639,-1.21435366404606));
#86896=CARTESIAN_POINT('',(0.3,-7.53377931054339,-1.32840855915201));
#86897=CARTESIAN_POINT('',(0.3,-8.12404506444685,-1.14816888602541));
#86898=CARTESIAN_POINT('',(9.,-7.53377931054339,-1.32840855915201));
#86899=CARTESIAN_POINT('',(0.3,-7.53377931054339,-1.32840855915201));
#86900=CARTESIAN_POINT('',(9.,-8.12404506444685,-1.14816888602541));
#86901=CARTESIAN_POINT('Origin',(9.,-7.80460144262175,-1.37616180801042));
#86902=CARTESIAN_POINT('',(9.,-7.84576201581982,-1.56333566169231));
#86903=CARTESIAN_POINT('Origin',(9.,0.,0.));
#86904=CARTESIAN_POINT('',(9.,-7.53377931054339,-1.32840855915201));
#86905=CARTESIAN_POINT('Origin',(0.3,-8.02680208495337,-1.69966122771224));
#86906=CARTESIAN_POINT('',(0.3,-7.84576201581982,-1.56333566169231));
#86907=CARTESIAN_POINT('',(4.5,-7.84576201581982,-1.56333566169231));
#86908=CARTESIAN_POINT('',(0.3,-7.53377931054339,-1.32840855915201));
#86909=CARTESIAN_POINT('Origin',(0.3,-7.80460144262175,-1.37616180801042));
#86910=CARTESIAN_POINT('Origin',(0.3,0.,0.));
#86911=CARTESIAN_POINT('Origin',(0.3,-7.65,9.36854801347725E-16));
#86912=CARTESIAN_POINT('',(0.3,-7.99803765020264,0.177182803739527));
#86913=CARTESIAN_POINT('',(9.,-7.99803765020264,0.177182803739527));
#86914=CARTESIAN_POINT('',(4.5,-7.99803765020264,0.177182803739528));
#86915=CARTESIAN_POINT('',(0.3,-7.65,9.36854801347725E-16));
#86916=CARTESIAN_POINT('',(0.3,-8.2,0.280000000000001));
#86917=CARTESIAN_POINT('',(9.,-7.65,9.36854801347725E-16));
#86918=CARTESIAN_POINT('',(0.3,-7.65,9.36854801347725E-16));
#86919=CARTESIAN_POINT('',(9.,-8.2,0.280000000000001));
#86920=CARTESIAN_POINT('Origin',(9.,-7.925,9.70532588324277E-16));
#86921=CARTESIAN_POINT('',(9.,-8.,-9.79717439317883E-16));
#86922=CARTESIAN_POINT('Origin',(9.,0.,0.));
#86923=CARTESIAN_POINT('',(9.,-7.99803765020264,-0.177182803739526));
#86924=CARTESIAN_POINT('',(9.,-7.65,9.36854801347725E-16));
#86925=CARTESIAN_POINT('Origin',(9.,0.,0.));
#86926=CARTESIAN_POINT('Origin',(0.3,-8.2,-0.279999999999999));
#86927=CARTESIAN_POINT('',(0.3,-7.99803765020264,-0.177182803739526));
#86928=CARTESIAN_POINT('',(4.5,-7.99803765020264,-0.177182803739526));
#86929=CARTESIAN_POINT('',(0.3,-7.65,9.36854801347725E-16));
#86930=CARTESIAN_POINT('Origin',(0.3,-7.925,9.70532588324277E-16));
#86931=CARTESIAN_POINT('',(0.3,-8.,-9.79717439317883E-16));
#86932=CARTESIAN_POINT('Origin',(0.3,0.,0.));
#86933=CARTESIAN_POINT('Origin',(0.3,0.,0.));
#86934=CARTESIAN_POINT('Origin',(0.3,-7.53377931054339,1.32840855915202));
#86935=CARTESIAN_POINT('',(0.3,-7.84576201581982,1.56333566169232));
#86936=CARTESIAN_POINT('',(9.,-7.84576201581982,1.56333566169232));
#86937=CARTESIAN_POINT('',(4.5,-7.84576201581982,1.56333566169232));
#86938=CARTESIAN_POINT('',(0.3,-7.53377931054339,1.32840855915202));
#86939=CARTESIAN_POINT('',(0.3,-8.02680208495337,1.69966122771225));
#86940=CARTESIAN_POINT('',(9.,-7.53377931054339,1.32840855915202));
#86941=CARTESIAN_POINT('',(0.3,-7.53377931054339,1.32840855915202));
#86942=CARTESIAN_POINT('',(9.,-8.02680208495337,1.69966122771225));
#86943=CARTESIAN_POINT('Origin',(9.,-7.80460144262175,1.37616180801043));
#86944=CARTESIAN_POINT('',(9.,-7.90729695778639,1.21435366404606));
#86945=CARTESIAN_POINT('Origin',(9.,0.,0.));
#86946=CARTESIAN_POINT('',(9.,-7.53377931054339,1.32840855915202));
#86947=CARTESIAN_POINT('Origin',(0.3,-8.12404506444685,1.14816888602541));
#86948=CARTESIAN_POINT('',(0.3,-7.90729695778639,1.21435366404606));
#86949=CARTESIAN_POINT('',(4.5,-7.90729695778639,1.21435366404606));
#86950=CARTESIAN_POINT('',(0.3,-7.53377931054339,1.32840855915202));
#86951=CARTESIAN_POINT('Origin',(0.3,-7.80460144262175,1.37616180801043));
#86952=CARTESIAN_POINT('Origin',(0.3,0.,0.));
#86953=CARTESIAN_POINT('Origin',(0.3,-7.1886485490122,2.61645409644137));
#86954=CARTESIAN_POINT('',(0.3,-7.45509687273345,2.90198735665059));
#86955=CARTESIAN_POINT('',(9.,-7.45509687273345,2.90198735665059));
#86956=CARTESIAN_POINT('',(4.5,-7.45509687273345,2.90198735665059));
#86957=CARTESIAN_POINT('',(0.3,-7.1886485490122,2.61645409644137));
#86958=CARTESIAN_POINT('',(0.3,-7.60971385031326,3.06767910909054));
#86959=CARTESIAN_POINT('',(9.,-7.1886485490122,2.61645409644137));
#86960=CARTESIAN_POINT('',(0.3,-7.1886485490122,2.61645409644137));
#86961=CARTESIAN_POINT('',(9.,-7.60971385031326,3.06767910909054));
#86962=CARTESIAN_POINT('Origin',(9.,-7.44706401972832,2.71050963585593));
#86963=CARTESIAN_POINT('',(9.,-7.57629704859313,2.56899261024221));
#86964=CARTESIAN_POINT('Origin',(9.,0.,0.));
#86965=CARTESIAN_POINT('',(9.,-7.1886485490122,2.61645409644137));
#86966=CARTESIAN_POINT('Origin',(0.3,-7.80124513057564,2.54145124145043));
#86967=CARTESIAN_POINT('',(0.3,-7.57629704859313,2.56899261024221));
#86968=CARTESIAN_POINT('',(4.5,-7.57629704859313,2.56899261024221));
#86969=CARTESIAN_POINT('',(0.3,-7.1886485490122,2.61645409644137));
#86970=CARTESIAN_POINT('Origin',(0.3,-7.44706401972832,2.71050963585593));
#86971=CARTESIAN_POINT('Origin',(0.3,0.,0.));
#86972=CARTESIAN_POINT('Origin',(0.3,-6.62509433895096,3.825));
#86973=CARTESIAN_POINT('',(0.3,-6.83791238363012,4.1524636342535));
#86974=CARTESIAN_POINT('',(9.,-6.83791238363012,4.1524636342535));
#86975=CARTESIAN_POINT('',(4.5,-6.83791238363012,4.1524636342535));
#86976=CARTESIAN_POINT('',(0.3,-6.62509433895096,3.825));
#86977=CARTESIAN_POINT('',(0.3,-6.9614083110324,4.34248711305964));
#86978=CARTESIAN_POINT('',(9.,-6.62509433895096,3.825));
#86979=CARTESIAN_POINT('',(0.3,-6.62509433895096,3.825));
#86980=CARTESIAN_POINT('',(9.,-6.9614083110324,4.34248711305964));
#86981=CARTESIAN_POINT('Origin',(9.,-6.86325132499168,3.9625));
#86982=CARTESIAN_POINT('',(9.,-7.01509518736965,3.84557401594914));
#86983=CARTESIAN_POINT('Origin',(9.,0.,0.));
#86984=CARTESIAN_POINT('',(9.,-6.62509433895096,3.825));
#86985=CARTESIAN_POINT('Origin',(0.3,-7.2414083110324,3.85751288694036));
#86986=CARTESIAN_POINT('',(0.3,-7.01509518736965,3.84557401594914));
#86987=CARTESIAN_POINT('',(4.5,-7.01509518736965,3.84557401594914));
#86988=CARTESIAN_POINT('',(0.3,-6.62509433895096,3.825));
#86989=CARTESIAN_POINT('Origin',(0.3,-6.86325132499168,3.9625));
#86990=CARTESIAN_POINT('Origin',(0.3,0.,0.));
#86991=CARTESIAN_POINT('Origin',(0.3,-5.86023998986018,4.91732521410203));
#86992=CARTESIAN_POINT('',(0.3,-6.01296138690081,5.27676940557761));
#86993=CARTESIAN_POINT('',(9.,-6.01296138690081,5.27676940557761));
#86994=CARTESIAN_POINT('',(4.5,-6.01296138690081,5.27676940557761));
#86995=CARTESIAN_POINT('',(0.3,-5.86023998986018,4.91732521410203));
#86996=CARTESIAN_POINT('',(0.3,-6.10158390286339,5.48535084350294));
#86997=CARTESIAN_POINT('',(9.,-5.86023998986018,4.91732521410203));
#86998=CARTESIAN_POINT('',(0.3,-5.86023998986018,4.91732521410203));
#86999=CARTESIAN_POINT('',(9.,-6.10158390286339,5.48535084350294));
#87000=CARTESIAN_POINT('Origin',(9.,-6.0709022117179,5.09409180676582));
#87001=CARTESIAN_POINT('',(9.,-6.24074320868739,5.0053096011358));
#87002=CARTESIAN_POINT('Origin',(9.,0.,0.));
#87003=CARTESIAN_POINT('',(9.,-5.86023998986018,4.91732521410203));
#87004=CARTESIAN_POINT('Origin',(0.3,-6.46154496428785,5.05636595535631));
#87005=CARTESIAN_POINT('',(0.3,-6.24074320868739,5.0053096011358));
#87006=CARTESIAN_POINT('',(4.5,-6.24074320868739,5.0053096011358));
#87007=CARTESIAN_POINT('',(0.3,-5.86023998986018,4.91732521410203));
#87008=CARTESIAN_POINT('Origin',(0.3,-6.0709022117179,5.09409180676582));
#87009=CARTESIAN_POINT('Origin',(0.3,0.,0.));
#87010=CARTESIAN_POINT('Origin',(0.3,-4.91732521410203,5.86023998986018));
#87011=CARTESIAN_POINT('',(0.3,-5.0053096011358,6.24074320868739));
#87012=CARTESIAN_POINT('',(9.,-5.0053096011358,6.24074320868739));
#87013=CARTESIAN_POINT('',(4.5,-5.0053096011358,6.24074320868739));
#87014=CARTESIAN_POINT('',(0.3,-4.91732521410203,5.86023998986018));
#87015=CARTESIAN_POINT('',(0.3,-5.05636595535631,6.46154496428785));
#87016=CARTESIAN_POINT('',(9.,-4.91732521410203,5.86023998986018));
#87017=CARTESIAN_POINT('',(0.3,-4.91732521410203,5.86023998986018));
#87018=CARTESIAN_POINT('',(9.,-5.05636595535631,6.46154496428785));
#87019=CARTESIAN_POINT('Origin',(9.,-5.09409180676582,6.0709022117179));
#87020=CARTESIAN_POINT('',(9.,-5.27676940557761,6.01296138690081));
#87021=CARTESIAN_POINT('Origin',(9.,0.,0.));
#87022=CARTESIAN_POINT('',(9.,-4.91732521410203,5.86023998986018));
#87023=CARTESIAN_POINT('Origin',(0.3,-5.48535084350294,6.10158390286339));
#87024=CARTESIAN_POINT('',(0.3,-5.27676940557761,6.01296138690081));
#87025=CARTESIAN_POINT('',(4.5,-5.27676940557761,6.01296138690081));
#87026=CARTESIAN_POINT('',(0.3,-4.91732521410203,5.86023998986018));
#87027=CARTESIAN_POINT('Origin',(0.3,-5.09409180676582,6.0709022117179));
#87028=CARTESIAN_POINT('Origin',(0.3,0.,0.));
#87029=CARTESIAN_POINT('Origin',(0.3,-3.825,6.62509433895096));
#87030=CARTESIAN_POINT('',(0.3,-3.84557401594914,7.01509518736965));
#87031=CARTESIAN_POINT('',(9.,-3.84557401594914,7.01509518736965));
#87032=CARTESIAN_POINT('',(4.5,-3.84557401594914,7.01509518736965));
#87033=CARTESIAN_POINT('',(0.3,-3.825,6.62509433895096));
#87034=CARTESIAN_POINT('',(0.3,-3.85751288694036,7.2414083110324));
#87035=CARTESIAN_POINT('',(9.,-3.825,6.62509433895096));
#87036=CARTESIAN_POINT('',(0.3,-3.825,6.62509433895096));
#87037=CARTESIAN_POINT('',(9.,-3.85751288694036,7.2414083110324));
#87038=CARTESIAN_POINT('Origin',(9.,-3.9625,6.86325132499168));
#87039=CARTESIAN_POINT('',(9.,-4.1524636342535,6.83791238363012));
#87040=CARTESIAN_POINT('Origin',(9.,0.,0.));
#87041=CARTESIAN_POINT('',(9.,-3.825,6.62509433895096));
#87042=CARTESIAN_POINT('Origin',(0.3,-4.34248711305964,6.9614083110324));
#87043=CARTESIAN_POINT('',(0.3,-4.1524636342535,6.83791238363012));
#87044=CARTESIAN_POINT('',(4.5,-4.1524636342535,6.83791238363012));
#87045=CARTESIAN_POINT('',(0.3,-3.825,6.62509433895096));
#87046=CARTESIAN_POINT('Origin',(0.3,-3.9625,6.86325132499168));
#87047=CARTESIAN_POINT('Origin',(0.3,0.,0.));
#87048=CARTESIAN_POINT('Origin',(0.3,-2.61645409644137,7.1886485490122));
#87049=CARTESIAN_POINT('',(0.3,-2.56899261024221,7.57629704859313));
#87050=CARTESIAN_POINT('',(9.,-2.56899261024221,7.57629704859313));
#87051=CARTESIAN_POINT('',(4.5,-2.56899261024221,7.57629704859313));
#87052=CARTESIAN_POINT('',(0.3,-2.61645409644137,7.1886485490122));
#87053=CARTESIAN_POINT('',(0.3,-2.54145124145043,7.80124513057564));
#87054=CARTESIAN_POINT('',(9.,-2.61645409644137,7.1886485490122));
#87055=CARTESIAN_POINT('',(0.3,-2.61645409644137,7.1886485490122));
#87056=CARTESIAN_POINT('',(9.,-2.54145124145043,7.80124513057564));
#87057=CARTESIAN_POINT('Origin',(9.,-2.71050963585592,7.44706401972832));
#87058=CARTESIAN_POINT('',(9.,-2.90198735665059,7.45509687273345));
#87059=CARTESIAN_POINT('Origin',(9.,0.,0.));
#87060=CARTESIAN_POINT('',(9.,-2.61645409644137,7.1886485490122));
#87061=CARTESIAN_POINT('Origin',(0.3,-3.06767910909054,7.60971385031326));
#87062=CARTESIAN_POINT('',(0.3,-2.90198735665059,7.45509687273345));
#87063=CARTESIAN_POINT('',(4.5,-2.90198735665059,7.45509687273345));
#87064=CARTESIAN_POINT('',(0.3,-2.61645409644137,7.1886485490122));
#87065=CARTESIAN_POINT('Origin',(0.3,-2.71050963585592,7.44706401972832));
#87066=CARTESIAN_POINT('Origin',(0.3,0.,0.));
#87067=CARTESIAN_POINT('Origin',(0.3,-1.32840855915202,7.53377931054339));
#87068=CARTESIAN_POINT('',(0.3,-1.21435366404606,7.90729695778639));
#87069=CARTESIAN_POINT('',(9.,-1.21435366404606,7.90729695778639));
#87070=CARTESIAN_POINT('',(4.5,-1.21435366404606,7.90729695778639));
#87071=CARTESIAN_POINT('',(0.3,-1.32840855915202,7.53377931054339));
#87072=CARTESIAN_POINT('',(0.3,-1.14816888602541,8.12404506444685));
#87073=CARTESIAN_POINT('',(9.,-1.32840855915202,7.53377931054339));
#87074=CARTESIAN_POINT('',(0.3,-1.32840855915202,7.53377931054339));
#87075=CARTESIAN_POINT('',(9.,-1.14816888602541,8.12404506444685));
#87076=CARTESIAN_POINT('Origin',(9.,-1.37616180801042,7.80460144262175));
#87077=CARTESIAN_POINT('',(9.,-1.56333566169231,7.84576201581982));
#87078=CARTESIAN_POINT('Origin',(9.,0.,0.));
#87079=CARTESIAN_POINT('',(9.,-1.32840855915202,7.53377931054339));
#87080=CARTESIAN_POINT('Origin',(0.3,-1.69966122771225,8.02680208495337));
#87081=CARTESIAN_POINT('',(0.3,-1.56333566169231,7.84576201581982));
#87082=CARTESIAN_POINT('',(4.5,-1.56333566169231,7.84576201581982));
#87083=CARTESIAN_POINT('',(0.3,-1.32840855915202,7.53377931054339));
#87084=CARTESIAN_POINT('Origin',(0.3,-1.37616180801042,7.80460144262175));
#87085=CARTESIAN_POINT('Origin',(0.3,0.,0.));
#87086=CARTESIAN_POINT('Origin',(0.3,4.68427400673863E-16,7.65));
#87087=CARTESIAN_POINT('',(0.3,0.177182803739527,7.99803765020264));
#87088=CARTESIAN_POINT('',(9.,0.177182803739527,7.99803765020264));
#87089=CARTESIAN_POINT('',(4.5,0.177182803739527,7.99803765020264));
#87090=CARTESIAN_POINT('',(0.3,4.68427400673863E-16,7.65));
#87091=CARTESIAN_POINT('',(0.3,0.28,8.2));
#87092=CARTESIAN_POINT('',(9.,4.68427400673863E-16,7.65));
#87093=CARTESIAN_POINT('',(0.3,4.68427400673863E-16,7.65));
#87094=CARTESIAN_POINT('',(9.,0.28,8.2));
#87095=CARTESIAN_POINT('Origin',(9.,4.85266294162139E-16,7.925));
#87096=CARTESIAN_POINT('',(9.,-0.177182803739526,7.99803765020264));
#87097=CARTESIAN_POINT('Origin',(9.,0.,0.));
#87098=CARTESIAN_POINT('',(9.,4.68427400673863E-16,7.65));
#87099=CARTESIAN_POINT('Origin',(0.3,-0.279999999999999,8.2));
#87100=CARTESIAN_POINT('',(0.3,-0.177182803739526,7.99803765020264));
#87101=CARTESIAN_POINT('',(4.5,-0.177182803739526,7.99803765020264));
#87102=CARTESIAN_POINT('',(0.3,4.68427400673863E-16,7.65));
#87103=CARTESIAN_POINT('Origin',(0.3,4.85266294162139E-16,7.925));
#87104=CARTESIAN_POINT('Origin',(0.3,0.,0.));
#87105=CARTESIAN_POINT('Origin',(0.3,1.32840855915202,7.53377931054339));
#87106=CARTESIAN_POINT('',(0.3,1.56333566169231,7.84576201581982));
#87107=CARTESIAN_POINT('',(9.,1.56333566169231,7.84576201581982));
#87108=CARTESIAN_POINT('',(4.5,1.56333566169231,7.84576201581982));
#87109=CARTESIAN_POINT('',(0.3,1.32840855915202,7.53377931054339));
#87110=CARTESIAN_POINT('',(0.3,1.69966122771225,8.02680208495337));
#87111=CARTESIAN_POINT('',(9.,1.32840855915202,7.53377931054339));
#87112=CARTESIAN_POINT('',(0.3,1.32840855915202,7.53377931054339));
#87113=CARTESIAN_POINT('',(9.,1.69966122771225,8.02680208495337));
#87114=CARTESIAN_POINT('Origin',(9.,1.37616180801042,7.80460144262175));
#87115=CARTESIAN_POINT('',(9.,1.21435366404606,7.90729695778639));
#87116=CARTESIAN_POINT('Origin',(9.,0.,0.));
#87117=CARTESIAN_POINT('',(9.,1.32840855915202,7.53377931054339));
#87118=CARTESIAN_POINT('Origin',(0.3,1.14816888602541,8.12404506444685));
#87119=CARTESIAN_POINT('',(0.3,1.21435366404606,7.90729695778639));
#87120=CARTESIAN_POINT('',(4.5,1.21435366404606,7.90729695778639));
#87121=CARTESIAN_POINT('',(0.3,1.32840855915202,7.53377931054339));
#87122=CARTESIAN_POINT('Origin',(0.3,1.37616180801042,7.80460144262175));
#87123=CARTESIAN_POINT('Origin',(0.3,0.,0.));
#87124=CARTESIAN_POINT('Origin',(0.3,2.61645409644137,7.1886485490122));
#87125=CARTESIAN_POINT('',(0.3,2.90198735665059,7.45509687273345));
#87126=CARTESIAN_POINT('',(9.,2.90198735665059,7.45509687273345));
#87127=CARTESIAN_POINT('',(4.5,2.90198735665059,7.45509687273345));
#87128=CARTESIAN_POINT('',(0.3,2.61645409644137,7.1886485490122));
#87129=CARTESIAN_POINT('',(0.3,3.06767910909054,7.60971385031326));
#87130=CARTESIAN_POINT('',(9.,2.61645409644137,7.1886485490122));
#87131=CARTESIAN_POINT('',(0.3,2.61645409644137,7.1886485490122));
#87132=CARTESIAN_POINT('',(9.,3.06767910909054,7.60971385031326));
#87133=CARTESIAN_POINT('Origin',(9.,2.71050963585593,7.44706401972832));
#87134=CARTESIAN_POINT('',(9.,2.56899261024221,7.57629704859313));
#87135=CARTESIAN_POINT('Origin',(9.,0.,0.));
#87136=CARTESIAN_POINT('',(9.,2.61645409644137,7.1886485490122));
#87137=CARTESIAN_POINT('Origin',(0.3,2.54145124145043,7.80124513057564));
#87138=CARTESIAN_POINT('',(0.3,2.56899261024221,7.57629704859313));
#87139=CARTESIAN_POINT('',(4.5,2.56899261024221,7.57629704859313));
#87140=CARTESIAN_POINT('',(0.3,2.61645409644137,7.1886485490122));
#87141=CARTESIAN_POINT('Origin',(0.3,2.71050963585593,7.44706401972832));
#87142=CARTESIAN_POINT('Origin',(0.3,0.,0.));
#87143=CARTESIAN_POINT('Origin',(0.3,3.825,6.62509433895096));
#87144=CARTESIAN_POINT('',(0.3,4.15246363425351,6.83791238363012));
#87145=CARTESIAN_POINT('',(9.,4.15246363425351,6.83791238363012));
#87146=CARTESIAN_POINT('',(4.5,4.15246363425351,6.83791238363012));
#87147=CARTESIAN_POINT('',(0.3,3.825,6.62509433895096));
#87148=CARTESIAN_POINT('',(0.3,4.34248711305964,6.96140831103239));
#87149=CARTESIAN_POINT('',(9.,3.825,6.62509433895096));
#87150=CARTESIAN_POINT('',(0.3,3.825,6.62509433895096));
#87151=CARTESIAN_POINT('',(9.,4.34248711305964,6.96140831103239));
#87152=CARTESIAN_POINT('Origin',(9.,3.9625,6.86325132499168));
#87153=CARTESIAN_POINT('',(9.,3.84557401594914,7.01509518736965));
#87154=CARTESIAN_POINT('Origin',(9.,0.,0.));
#87155=CARTESIAN_POINT('',(9.,3.825,6.62509433895096));
#87156=CARTESIAN_POINT('Origin',(0.3,3.85751288694036,7.2414083110324));
#87157=CARTESIAN_POINT('',(0.3,3.84557401594914,7.01509518736965));
#87158=CARTESIAN_POINT('',(4.5,3.84557401594914,7.01509518736965));
#87159=CARTESIAN_POINT('',(0.3,3.825,6.62509433895096));
#87160=CARTESIAN_POINT('Origin',(0.3,3.9625,6.86325132499168));
#87161=CARTESIAN_POINT('Origin',(0.3,0.,0.));
#87162=CARTESIAN_POINT('Origin',(0.3,4.91732521410203,5.86023998986018));
#87163=CARTESIAN_POINT('',(0.3,5.27676940557761,6.01296138690081));
#87164=CARTESIAN_POINT('',(9.,5.27676940557761,6.01296138690081));
#87165=CARTESIAN_POINT('',(4.5,5.27676940557761,6.01296138690081));
#87166=CARTESIAN_POINT('',(0.3,4.91732521410203,5.86023998986018));
#87167=CARTESIAN_POINT('',(0.3,5.48535084350294,6.10158390286339));
#87168=CARTESIAN_POINT('',(9.,4.91732521410203,5.86023998986018));
#87169=CARTESIAN_POINT('',(0.3,4.91732521410203,5.86023998986018));
#87170=CARTESIAN_POINT('',(9.,5.48535084350294,6.10158390286339));
#87171=CARTESIAN_POINT('Origin',(9.,5.09409180676582,6.0709022117179));
#87172=CARTESIAN_POINT('',(9.,5.0053096011358,6.24074320868739));
#87173=CARTESIAN_POINT('Origin',(9.,0.,0.));
#87174=CARTESIAN_POINT('',(9.,4.91732521410203,5.86023998986018));
#87175=CARTESIAN_POINT('Origin',(0.3,5.05636595535631,6.46154496428785));
#87176=CARTESIAN_POINT('',(0.3,5.0053096011358,6.24074320868739));
#87177=CARTESIAN_POINT('',(4.5,5.0053096011358,6.24074320868739));
#87178=CARTESIAN_POINT('',(0.3,4.91732521410203,5.86023998986018));
#87179=CARTESIAN_POINT('Origin',(0.3,5.09409180676582,6.0709022117179));
#87180=CARTESIAN_POINT('Origin',(0.3,0.,0.));
#87181=CARTESIAN_POINT('Origin',(0.3,5.86023998986018,4.91732521410203));
#87182=CARTESIAN_POINT('',(0.3,6.24074320868739,5.0053096011358));
#87183=CARTESIAN_POINT('',(9.,6.24074320868739,5.0053096011358));
#87184=CARTESIAN_POINT('',(4.5,6.24074320868739,5.0053096011358));
#87185=CARTESIAN_POINT('',(0.3,5.86023998986018,4.91732521410203));
#87186=CARTESIAN_POINT('',(0.3,6.46154496428785,5.05636595535631));
#87187=CARTESIAN_POINT('',(9.,5.86023998986018,4.91732521410203));
#87188=CARTESIAN_POINT('',(0.3,5.86023998986018,4.91732521410203));
#87189=CARTESIAN_POINT('',(9.,6.46154496428785,5.05636595535631));
#87190=CARTESIAN_POINT('Origin',(9.,6.0709022117179,5.09409180676582));
#87191=CARTESIAN_POINT('',(9.,6.01296138690081,5.27676940557761));
#87192=CARTESIAN_POINT('Origin',(9.,0.,0.));
#87193=CARTESIAN_POINT('',(9.,5.86023998986018,4.91732521410203));
#87194=CARTESIAN_POINT('Origin',(0.3,6.10158390286339,5.48535084350294));
#87195=CARTESIAN_POINT('',(0.3,6.01296138690081,5.27676940557761));
#87196=CARTESIAN_POINT('',(4.5,6.01296138690081,5.27676940557761));
#87197=CARTESIAN_POINT('',(0.3,5.86023998986018,4.91732521410203));
#87198=CARTESIAN_POINT('Origin',(0.3,6.0709022117179,5.09409180676582));
#87199=CARTESIAN_POINT('Origin',(0.3,0.,0.));
#87200=CARTESIAN_POINT('Origin',(0.3,6.62509433895096,3.825));
#87201=CARTESIAN_POINT('',(0.3,7.01509518736965,3.84557401594914));
#87202=CARTESIAN_POINT('',(9.,7.01509518736965,3.84557401594914));
#87203=CARTESIAN_POINT('',(4.5,7.01509518736965,3.84557401594914));
#87204=CARTESIAN_POINT('',(0.3,6.62509433895096,3.825));
#87205=CARTESIAN_POINT('',(0.3,7.2414083110324,3.85751288694036));
#87206=CARTESIAN_POINT('',(9.,6.62509433895096,3.825));
#87207=CARTESIAN_POINT('',(0.3,6.62509433895096,3.825));
#87208=CARTESIAN_POINT('',(9.,7.2414083110324,3.85751288694036));
#87209=CARTESIAN_POINT('Origin',(9.,6.86325132499168,3.9625));
#87210=CARTESIAN_POINT('',(9.,6.83791238363012,4.1524636342535));
#87211=CARTESIAN_POINT('Origin',(9.,0.,0.));
#87212=CARTESIAN_POINT('',(9.,6.62509433895096,3.825));
#87213=CARTESIAN_POINT('Origin',(0.3,6.9614083110324,4.34248711305964));
#87214=CARTESIAN_POINT('',(0.3,6.83791238363012,4.1524636342535));
#87215=CARTESIAN_POINT('',(4.5,6.83791238363012,4.1524636342535));
#87216=CARTESIAN_POINT('',(0.3,6.62509433895096,3.825));
#87217=CARTESIAN_POINT('Origin',(0.3,6.86325132499168,3.9625));
#87218=CARTESIAN_POINT('Origin',(0.3,0.,0.));
#87219=CARTESIAN_POINT('Origin',(0.3,7.1886485490122,2.61645409644137));
#87220=CARTESIAN_POINT('',(0.3,7.57629704859313,2.56899261024221));
#87221=CARTESIAN_POINT('',(9.,7.57629704859313,2.56899261024221));
#87222=CARTESIAN_POINT('',(4.5,7.57629704859313,2.56899261024221));
#87223=CARTESIAN_POINT('',(0.3,7.1886485490122,2.61645409644137));
#87224=CARTESIAN_POINT('',(0.3,7.80124513057564,2.54145124145043));
#87225=CARTESIAN_POINT('',(9.,7.1886485490122,2.61645409644137));
#87226=CARTESIAN_POINT('',(0.3,7.1886485490122,2.61645409644137));
#87227=CARTESIAN_POINT('',(9.,7.80124513057564,2.54145124145043));
#87228=CARTESIAN_POINT('Origin',(9.,7.44706401972832,2.71050963585592));
#87229=CARTESIAN_POINT('',(9.,7.45509687273345,2.90198735665059));
#87230=CARTESIAN_POINT('Origin',(9.,0.,0.));
#87231=CARTESIAN_POINT('',(9.,7.1886485490122,2.61645409644137));
#87232=CARTESIAN_POINT('Origin',(0.3,7.60971385031326,3.06767910909054));
#87233=CARTESIAN_POINT('',(0.3,7.45509687273345,2.90198735665059));
#87234=CARTESIAN_POINT('',(4.5,7.45509687273345,2.90198735665059));
#87235=CARTESIAN_POINT('',(0.3,7.1886485490122,2.61645409644137));
#87236=CARTESIAN_POINT('Origin',(0.3,7.44706401972832,2.71050963585592));
#87237=CARTESIAN_POINT('Origin',(0.3,0.,0.));
#87238=CARTESIAN_POINT('Origin',(0.3,7.53377931054339,1.32840855915202));
#87239=CARTESIAN_POINT('',(0.3,7.90729695778639,1.21435366404606));
#87240=CARTESIAN_POINT('',(9.,7.90729695778639,1.21435366404606));
#87241=CARTESIAN_POINT('',(4.5,7.90729695778639,1.21435366404606));
#87242=CARTESIAN_POINT('',(0.3,7.53377931054339,1.32840855915202));
#87243=CARTESIAN_POINT('',(0.3,8.12404506444685,1.14816888602541));
#87244=CARTESIAN_POINT('',(9.,7.53377931054339,1.32840855915202));
#87245=CARTESIAN_POINT('',(0.3,7.53377931054339,1.32840855915202));
#87246=CARTESIAN_POINT('',(9.,8.12404506444685,1.14816888602541));
#87247=CARTESIAN_POINT('Origin',(9.,7.80460144262175,1.37616180801042));
#87248=CARTESIAN_POINT('',(9.,7.84576201581982,1.56333566169231));
#87249=CARTESIAN_POINT('Origin',(9.,0.,0.));
#87250=CARTESIAN_POINT('',(9.,7.53377931054339,1.32840855915202));
#87251=CARTESIAN_POINT('Origin',(0.3,8.02680208495337,1.69966122771225));
#87252=CARTESIAN_POINT('',(0.3,7.84576201581982,1.56333566169231));
#87253=CARTESIAN_POINT('',(4.5,7.84576201581982,1.56333566169232));
#87254=CARTESIAN_POINT('',(0.3,7.53377931054339,1.32840855915202));
#87255=CARTESIAN_POINT('Origin',(0.3,7.80460144262175,1.37616180801042));
#87256=CARTESIAN_POINT('Origin',(0.3,0.,0.));
#87257=CARTESIAN_POINT('Origin',(9.,7.925,0.));
#87258=CARTESIAN_POINT('',(9.,7.99803765020264,-0.177182803739528));
#87259=CARTESIAN_POINT('',(9.,7.99803765020264,0.177182803739527));
#87260=CARTESIAN_POINT('Origin',(9.,0.,0.));
#87261=CARTESIAN_POINT('',(9.,7.65,0.));
#87262=CARTESIAN_POINT('',(9.,8.2,-0.28));
#87263=CARTESIAN_POINT('',(9.,7.65,0.));
#87264=CARTESIAN_POINT('Origin',(0.3,7.65,0.));
#87265=CARTESIAN_POINT('',(0.3,7.99803765020264,-0.177182803739528));
#87266=CARTESIAN_POINT('',(4.5,7.99803765020264,-0.177182803739527));
#87267=CARTESIAN_POINT('',(0.3,7.65,0.));
#87268=CARTESIAN_POINT('',(0.3,8.2,-0.28));
#87269=CARTESIAN_POINT('',(0.3,7.65,0.));
#87270=CARTESIAN_POINT('Origin',(0.3,8.2,0.28));
#87271=CARTESIAN_POINT('',(0.3,7.99803765020264,0.177182803739527));
#87272=CARTESIAN_POINT('',(4.5,7.99803765020264,0.177182803739528));
#87273=CARTESIAN_POINT('',(0.3,7.65,0.));
#87274=CARTESIAN_POINT('Origin',(0.3,7.925,0.));
#87275=CARTESIAN_POINT('Origin',(0.3,0.,0.));
#87276=CARTESIAN_POINT('Origin',(3.80327876194488,0.,0.));
#87277=CARTESIAN_POINT('',(2.59655752388976,0.,0.));
#87278=CARTESIAN_POINT('',(5.,-3.98342616391485,4.87829010127814E-16));
#87279=CARTESIAN_POINT('',(3.80327876194488,-2.,-2.44929359829471E-16));
#87280=CARTESIAN_POINT('Origin',(5.,0.,0.));
#87281=CARTESIAN_POINT('Origin',(5.,2.82820063659975E-16,4.61880215351701));
#87282=CARTESIAN_POINT('',(10.,-4.,2.3094010767585));
#87283=CARTESIAN_POINT('',(10.,2.82820063659975E-16,4.61880215351701));
#87284=CARTESIAN_POINT('',(10.,-1.,4.04145188432738));
#87285=CARTESIAN_POINT('',(5.,-4.,2.3094010767585));
#87286=CARTESIAN_POINT('',(5.,-4.,2.3094010767585));
#87287=CARTESIAN_POINT('',(5.,2.82820063659975E-16,4.61880215351701));
#87288=CARTESIAN_POINT('',(5.,2.82820063659975E-16,4.61880215351701));
#87289=CARTESIAN_POINT('',(5.,2.82820063659975E-16,4.61880215351701));
#87290=CARTESIAN_POINT('Origin',(5.,4.,2.3094010767585));
#87291=CARTESIAN_POINT('',(10.,4.,2.3094010767585));
#87292=CARTESIAN_POINT('',(10.,3.,2.88675134594813));
#87293=CARTESIAN_POINT('',(5.,4.,2.3094010767585));
#87294=CARTESIAN_POINT('',(5.,4.,2.3094010767585));
#87295=CARTESIAN_POINT('',(5.,4.,2.3094010767585));
#87296=CARTESIAN_POINT('Origin',(5.,4.,-2.30940107675851));
#87297=CARTESIAN_POINT('',(10.,4.,-2.30940107675851));
#87298=CARTESIAN_POINT('',(10.,4.,-1.15470053837925));
#87299=CARTESIAN_POINT('',(5.,4.,-2.30940107675851));
#87300=CARTESIAN_POINT('',(5.,4.,-2.30940107675851));
#87301=CARTESIAN_POINT('',(5.,4.,-2.30940107675851));
#87302=CARTESIAN_POINT('Origin',(5.,-8.48460190979926E-16,-4.61880215351701));
#87303=CARTESIAN_POINT('',(10.,-8.48460190979926E-16,-4.61880215351701));
#87304=CARTESIAN_POINT('',(10.,0.999999999999999,-4.04145188432738));
#87305=CARTESIAN_POINT('',(5.,-8.48460190979926E-16,-4.61880215351701));
#87306=CARTESIAN_POINT('',(5.,-8.48460190979926E-16,-4.61880215351701));
#87307=CARTESIAN_POINT('',(5.,-8.48460190979926E-16,-4.61880215351701));
#87308=CARTESIAN_POINT('Origin',(5.,-4.,-2.3094010767585));
#87309=CARTESIAN_POINT('',(10.,-4.,-2.3094010767585));
#87310=CARTESIAN_POINT('',(10.,-3.,-2.88675134594813));
#87311=CARTESIAN_POINT('',(5.,-4.,-2.3094010767585));
#87312=CARTESIAN_POINT('',(5.,-4.,-2.3094010767585));
#87313=CARTESIAN_POINT('',(5.,-4.,-2.3094010767585));
#87314=CARTESIAN_POINT('Origin',(5.,-4.,2.3094010767585));
#87315=CARTESIAN_POINT('',(10.,-4.,1.15470053837925));
#87316=CARTESIAN_POINT('',(5.,-4.,2.3094010767585));
#87317=CARTESIAN_POINT('Origin',(5.,0.,0.));
#87318=CARTESIAN_POINT('Origin',(-25.,4.,0.));
#87319=CARTESIAN_POINT('',(-25.,-4.,-4.89858719658941E-16));
#87320=CARTESIAN_POINT('Origin',(-25.,0.,0.));
#87321=CARTESIAN_POINT('Origin',(-24.5,0.,0.));
#87322=CARTESIAN_POINT('',(-24.5,-4.5,-5.51091059616309E-16));
#87323=CARTESIAN_POINT('Origin',(4.5,0.,0.));
#87324=CARTESIAN_POINT('Origin',(9.,0.,0.));
#87325=CARTESIAN_POINT('Origin',(9.,0.,0.));
#87326=CARTESIAN_POINT('Origin',(9.,0.,0.));
#87327=CARTESIAN_POINT('Origin',(9.,0.,0.));
#87328=CARTESIAN_POINT('Origin',(9.,0.,0.));
#87329=CARTESIAN_POINT('Origin',(9.,0.,0.));
#87330=CARTESIAN_POINT('Origin',(9.,0.,0.));
#87331=CARTESIAN_POINT('Origin',(9.,0.,0.));
#87332=CARTESIAN_POINT('Origin',(9.,0.,0.));
#87333=CARTESIAN_POINT('Origin',(9.,0.,0.));
#87334=CARTESIAN_POINT('Origin',(9.,0.,0.));
#87335=CARTESIAN_POINT('Origin',(9.,0.,0.));
#87336=CARTESIAN_POINT('Origin',(9.,0.,0.));
#87337=CARTESIAN_POINT('Origin',(9.,0.,0.));
#87338=CARTESIAN_POINT('Origin',(9.,0.,0.));
#87339=CARTESIAN_POINT('Origin',(9.,0.,0.));
#87340=CARTESIAN_POINT('Origin',(9.,0.,0.));
#87341=CARTESIAN_POINT('',(4.5,-8.,-9.79717439317883E-16));
#87342=CARTESIAN_POINT('Origin',(9.,0.,0.));
#87343=CARTESIAN_POINT('Origin',(9.,0.,0.));
#87344=CARTESIAN_POINT('Origin',(9.,0.,0.));
#87345=CARTESIAN_POINT('Origin',(9.,0.,0.));
#87346=CARTESIAN_POINT('Origin',(9.,0.,0.));
#87347=CARTESIAN_POINT('Origin',(9.,0.,0.));
#87348=CARTESIAN_POINT('Origin',(9.,0.,0.));
#87349=CARTESIAN_POINT('Origin',(9.,0.,0.));
#87350=CARTESIAN_POINT('Origin',(9.,0.,0.));
#87351=CARTESIAN_POINT('Origin',(9.,0.,0.));
#87352=CARTESIAN_POINT('Origin',(9.,0.,0.));
#87353=CARTESIAN_POINT('Origin',(9.,0.,0.));
#87354=CARTESIAN_POINT('Origin',(9.,0.,0.));
#87355=CARTESIAN_POINT('Origin',(9.,0.,0.));
#87356=CARTESIAN_POINT('Origin',(9.,0.,0.));
#87357=CARTESIAN_POINT('Origin',(9.,0.,0.));
#87358=CARTESIAN_POINT('Origin',(9.,0.,0.));
#87359=CARTESIAN_POINT('Origin',(9.,0.,0.));
#87360=CARTESIAN_POINT('Origin',(9.,0.,0.));
#87361=CARTESIAN_POINT('Origin',(9.5,0.,0.));
#87362=CARTESIAN_POINT('',(10.,-7.,-8.57252759403147E-16));
#87363=CARTESIAN_POINT('Origin',(10.,0.,0.));
#87364=CARTESIAN_POINT('',(9.5,-7.5,-9.18485099360515E-16));
#87365=CARTESIAN_POINT('Origin',(10.,0.,0.));
#94276=UNCERTAINTY_MEASURE_WITH_UNIT(LENGTH_MEASURE(0.01),#94302,
'DISTANCE_ACCURACY_VALUE',
'Maximum model space distance between geometric entities at asserted c
onnectivities');
#94285=UNCERTAINTY_MEASURE_WITH_UNIT(LENGTH_MEASURE(0.01),#94302,
'DISTANCE_ACCURACY_VALUE',
'Maximum model space distance between geometric entities at asserted c
onnectivities');
#94292=(
GEOMETRIC_REPRESENTATION_CONTEXT(3)
GLOBAL_UNCERTAINTY_ASSIGNED_CONTEXT((#94276))
GLOBAL_UNIT_ASSIGNED_CONTEXT((#94302,#94304,#94305))
REPRESENTATION_CONTEXT('','3D')
);
#94301=(
GEOMETRIC_REPRESENTATION_CONTEXT(3)
GLOBAL_UNCERTAINTY_ASSIGNED_CONTEXT((#94285))
GLOBAL_UNIT_ASSIGNED_CONTEXT((#94302,#94304,#94305))
REPRESENTATION_CONTEXT('','3D')
);
#94302=(
LENGTH_UNIT()
NAMED_UNIT(*)
SI_UNIT(.MILLI.,.METRE.)
);
#94304=(
NAMED_UNIT(*)
PLANE_ANGLE_UNIT()
SI_UNIT($,.RADIAN.)
);
#94305=(
NAMED_UNIT(*)
SI_UNIT($,.STERADIAN.)
SOLID_ANGLE_UNIT()
);
#94312=SHAPE_DEFINITION_REPRESENTATION(#94327,#94376);
#94327=PRODUCT_DEFINITION_SHAPE('',$,#94392);
#94376=SHAPE_REPRESENTATION('',(#54491),#94292);
#94385=PRODUCT_DEFINITION_CONTEXT('part definition',#94432,'design');
#94392=PRODUCT_DEFINITION('2026-10-11-08-26-38-736',
'06_ISO_4762_M10x25_SHCS',#94407,#94385);
#94407=PRODUCT_DEFINITION_FORMATION('',$,#94440);
#94432=APPLICATION_CONTEXT(
'Core Data for Automotive Mechanical Design Process');
#94433=PRODUCT_CONTEXT('part definition',#94432,'mechanical');
#94440=PRODUCT('2026-10-11-08-26-38-736','06_ISO_4762_M10x25_SHCS',$,(#94433));
#94582=COLOUR_RGB('Black',0.12,0.14,0.17);
#94583=FILL_AREA_STYLE_COLOUR('',#94582);
#94584=FILL_AREA_STYLE('',(#94583));
#94585=SURFACE_STYLE_FILL_AREA(#94584);
#94586=SURFACE_SIDE_STYLE('',(#94585));
#94587=SURFACE_STYLE_USAGE(.BOTH.,#94586);
#94588=PRESENTATION_STYLE_ASSIGNMENT((#94587));
ENDSEC;
END-ISO-10303-21;
